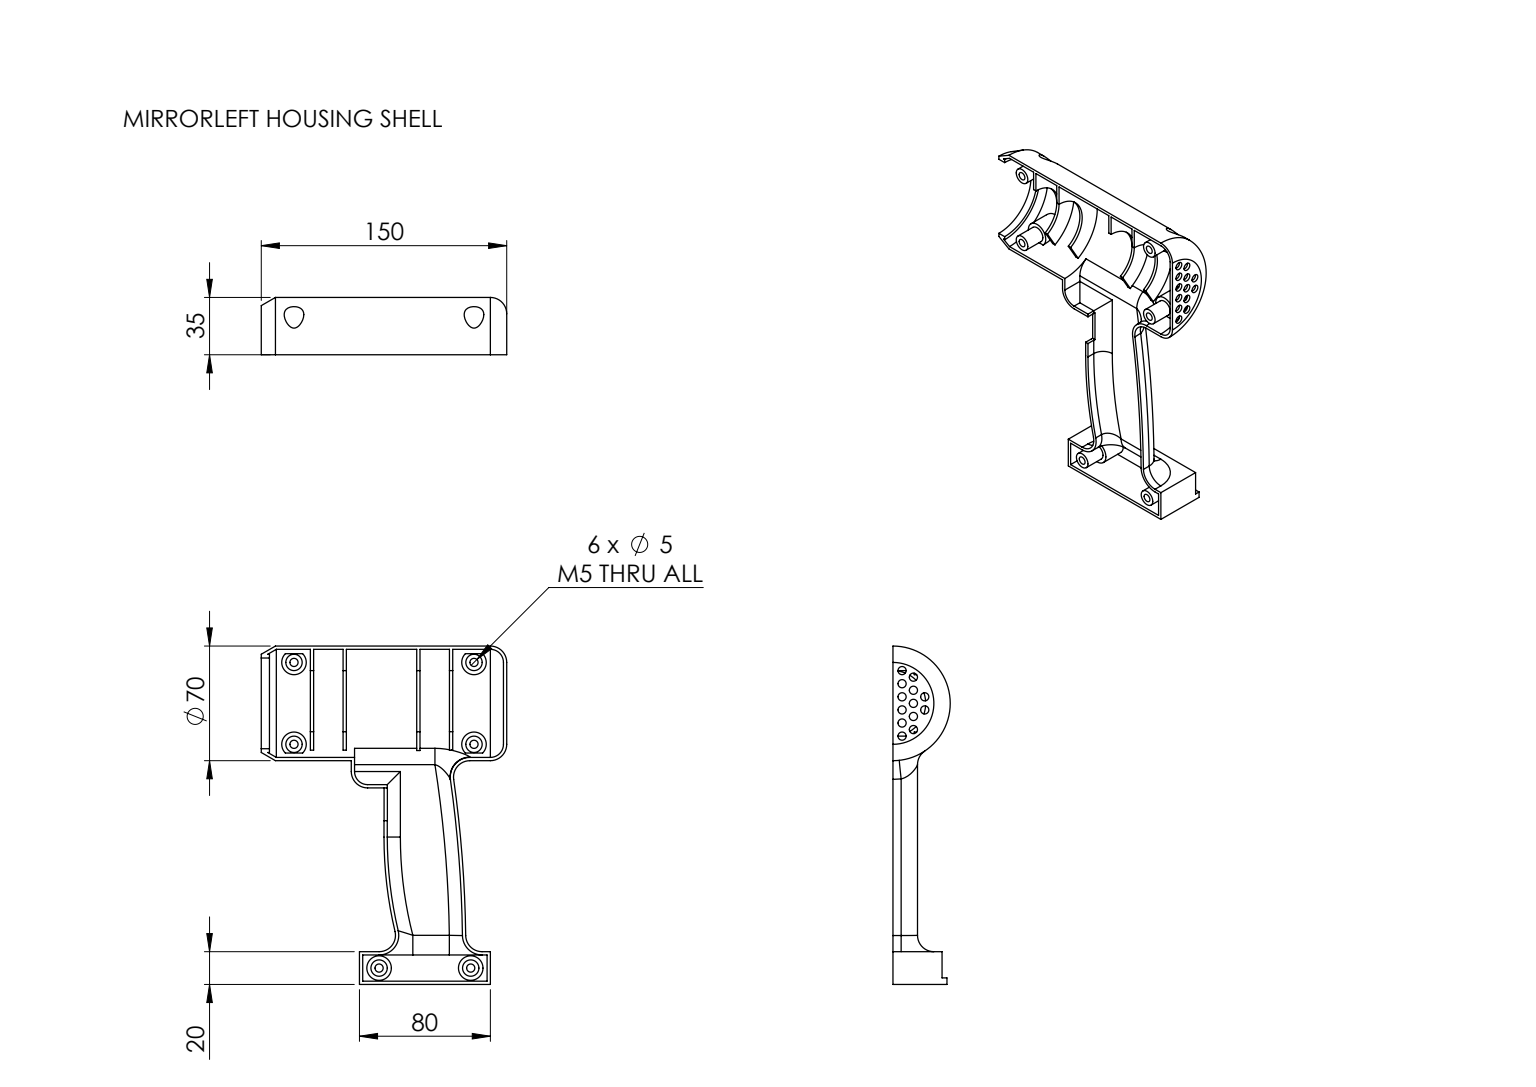
ISO-10303-21;
HEADER;
FILE_DESCRIPTION (('STEP AP214'),
    '1' );
FILE_NAME ('MirrorLeft Housing Shell.step',
    '2026-10-05T20:22:16',
    ( '' ),
    ( '' ),
    'SwSTEP 2.0',
    'SolidWorks 2026',
    '' );
FILE_SCHEMA (( 'AUTOMOTIVE_DESIGN' ));
ENDSEC;

DATA;
#1=B_SPLINE_CURVE_WITH_KNOTS ( 'NONE', 3,
 ( #12352, #9685, #8096, #1383, #14752, #16256, #12262, #13513, #2624, #1474, #13417, #8273, #9424, #10672, #226, #14828, #5538, #2709, #8188, #5630, #16442, #6792, #7929, #6603, #12185, #55, #13336, #5455, #10843, #10926, #4124, #11996, #2798, #16348, #13681, #6869, #9602, #15004, #9865, #16607, #8540, #3321, #16516, #15178, #7128, #4646, #4480, #11188, #15272, #15441 ),
 .UNSPECIFIED., .F., .F.,
 ( 4, 2, 2, 2, 2, 2, 2, 2, 2, 2, 2, 2, 2, 2, 2, 2, 2, 2, 2, 2, 2, 2, 2, 2, 4 ),
 ( 0.02172192739389853383, 0.02251948391625541862, 0.02331704043861230341, 0.02491215348332601748, 0.02650726652803973155, 0.02810237957275344908, 0.02969749261746715968, 0.03129260566218088069, 0.03209016218453770303, 0.03288771870689453231, 0.03328649696807296082, 0.03368527522925138240, 0.03448283175160819780, 0.03528038827396501320, 0.03567916653514340702, 0.03607794479632180085, 0.03687550131867862319, 0.03767305784103544553, 0.03847061436339226786, 0.03926817088574909020, 0.04086328393046270713, 0.04245839697517631711, 0.04405351001988992710, 0.04564862306460354402, 0.04724373610931716094 ),
 .UNSPECIFIED. ) ;
#5=DIRECTION ( 'NONE',  ( 0.000000000000000000, 0.000000000000000000, 1.000000000000000000 ) ) ;
#6=CARTESIAN_POINT ( 'NONE',  ( 27.15273249069231198, 18.00000000000000000, -20.88767039909325973 ) ) ;
#7=CARTESIAN_POINT ( 'NONE',  ( 25.49876332522149625, 18.00000000000000000, -21.99427390110736624 ) ) ;
#8=CYLINDRICAL_SURFACE ( 'NONE', #14336, 2.500000000000000444 ) ;
#9=DIRECTION ( 'NONE',  ( -1.000000000000000000, 0.000000000000000000, 0.000000000000000000 ) ) ;
#10=DIRECTION ( 'NONE',  ( -1.000000000000000000, -0.000000000000000000, -0.000000000000000000 ) ) ;
#13=CARTESIAN_POINT ( 'NONE',  ( 16.03791926353974162, 127.7299327228906520, -9.742640703122631862 ) ) ;
#14=CIRCLE ( 'NONE', #9896, 10.00000000000000178 ) ;
#18=CIRCLE ( 'NONE', #14435, 20.00000000000000355 ) ;
#23=ORIENTED_EDGE ( 'NONE', *, *, #10609, .T. ) ;
#26=AXIS2_PLACEMENT_3D ( 'NONE', #12707, #5981, #16782 ) ;
#28=AXIS2_PLACEMENT_3D ( 'NONE', #8615, #16596, #11271 ) ;
#31=DIRECTION ( 'NONE',  ( 0.000000000000000000, 0.000000000000000000, -1.000000000000000000 ) ) ;
#35=ORIENTED_EDGE ( 'NONE', *, *, #2235, .F. ) ;
#37=ORIENTED_EDGE ( 'NONE', *, *, #4762, .T. ) ;
#38=CARTESIAN_POINT ( 'NONE',  ( -80.30638721710498373, 189.1234298779548624, -27.97726104294732963 ) ) ;
#43=ORIENTED_EDGE ( 'NONE', *, *, #9422, .T. ) ;
#48=FACE_OUTER_BOUND ( 'NONE', #5615, .T. ) ;
#50=CARTESIAN_POINT ( 'NONE',  ( -48.00000000000000000, 143.0439382767972347, -16.49999999999984368 ) ) ;
#55=CARTESIAN_POINT ( 'NONE',  ( -79.71276265205243305, 202.6220268295897711, -16.24950730846250835 ) ) ;
#57=CARTESIAN_POINT ( 'NONE',  ( -95.00000000000000000, 171.6227766016838245, 0.000000000000000000 ) ) ;
#60=DIRECTION ( 'NONE',  ( 1.000000000000000000, 0.000000000000000000, 0.000000000000000000 ) ) ;
#62=ORIENTED_EDGE ( 'NONE', *, *, #6340, .T. ) ;
#65=SHAPE_REPRESENTATION_RELATIONSHIP ( 'NONE' , 'NONE' ,  #7924, #8036 ) ;
#67=DIRECTION ( 'NONE',  ( 8.673617379884037937E-17, 0.000000000000000000, 1.000000000000000000 ) ) ;
#70=EDGE_LOOP ( 'NONE', ( #17465, #2421, #13202, #13512 ) ) ;
#72=CARTESIAN_POINT ( 'NONE',  ( -48.00000000000000000, 191.6227766016837961, 1.224646799147353454E-15 ) ) ;
#73=DIRECTION ( 'NONE',  ( 1.000000000000000000, 0.000000000000000000, 0.000000000000000000 ) ) ;
#75=CARTESIAN_POINT ( 'NONE',  ( 15.93460003626540100, 136.8193095811535045, -3.708327557688629206 ) ) ;
#79=ORIENTED_EDGE ( 'NONE', *, *, #12627, .T. ) ;
#80=DIRECTION ( 'NONE',  ( 1.000000000000000000, 0.000000000000000000, 0.000000000000000000 ) ) ;
#82=LINE ( 'NONE', #2908, #5241 ) ;
#84=CARTESIAN_POINT ( 'NONE',  ( -74.45226540305546337, 194.3303362407250177, -26.63481108765543581 ) ) ;
#88=CARTESIAN_POINT ( 'NONE',  ( 24.94691999498327206, 18.00000000000000711, -22.32501294936691139 ) ) ;
#89=CARTESIAN_POINT ( 'NONE',  ( 23.77503517897901375, 18.00000000000000000, -22.95135521423614833 ) ) ;
#90=CARTESIAN_POINT ( 'NONE',  ( 37.50000000000000711, 196.6227766016838245, -35.00200000000000244 ) ) ;
#93=CARTESIAN_POINT ( 'NONE',  ( 26.85005685037350176, 141.4992599418080772, -17.82476597062854040 ) ) ;
#94=ORIENTED_EDGE ( 'NONE', *, *, #1318, .F. ) ;
#95=CARTESIAN_POINT ( 'NONE',  ( 6.927042533203191965, 134.0880917650273716, -15.00000000000000533 ) ) ;
#97=DIRECTION ( 'NONE',  ( 0.000000000000000000, 0.000000000000000000, 1.000000000000000000 ) ) ;
#98=CARTESIAN_POINT ( 'NONE',  ( 225.0000000000000000, 89.99999999999997158, -4.999999999999999112 ) ) ;
#101=LINE ( 'NONE', #8243, #15842 ) ;
#102=VERTEX_POINT ( 'NONE', #8434 ) ;
#107=CARTESIAN_POINT ( 'NONE',  ( 33.99999999999998579, 9.999999999999998224, -35.00000000000000000 ) ) ;
#108=ORIENTED_EDGE ( 'NONE', *, *, #12256, .F. ) ;
#110=ORIENTED_EDGE ( 'NONE', *, *, #17517, .F. ) ;
#112=EDGE_CURVE ( 'NONE', #17297, #3029, #16627, .T. ) ;
#113=ORIENTED_EDGE ( 'NONE', *, *, #13886, .F. ) ;
#114=EDGE_CURVE ( 'NONE', #730, #9326, #14586, .T. ) ;
#115=CARTESIAN_POINT ( 'NONE',  ( -78.86500048027876630, 189.1866491494219815, -27.93804624201380804 ) ) ;
#116=DIRECTION ( 'NONE',  ( 0.000000000000000000, 0.000000000000000000, 1.000000000000000000 ) ) ;
#117=( BOUNDED_SURFACE ( )  B_SPLINE_SURFACE ( 3, 2, ( 
 ( #14255, #2119, #7358 ),
 ( #807, #6197, #12760 ),
 ( #632, #11415, #4699 ),
 ( #16827, #8771, #2299 ),
 ( #9106, #17259, #13450 ),
 ( #5135, #5041, #10344 ),
 ( #3799, #16120, #1322 ),
 ( #15926, #965, #13280 ),
 ( #13364, #6550, #2476 ),
 ( #14512, #14600, #10434 ),
 ( #15848, #1058, #6637 ),
 ( #11850, #2379, #3721 ),
 ( #6458, #16018, #11941 ),
 ( #8042, #15754, #7870 ),
 ( #7772, #5213, #10523 ),
 ( #10610, #6729, #9194 ),
 ( #13185, #1148, #17343 ),
 ( #3900, #9284, #12126 ),
 ( #3631, #4951, #3997 ),
 ( #14695, #11759, #2575 ),
 ( #7961, #1231, #9021 ),
 ( #14436, #7692, #9377 ),
 ( #13099, #12030, #17435 ),
 ( #6362, #5310, #17170 ),
 ( #14779, #10704, #2651 ),
 ( #13711, #13812, #9715 ),
 ( #11051, #256, #7075 ),
 ( #1415, #4329, #341 ),
 ( #4156, #8392, #9541 ),
 ( #8220, #1582, #3039 ) ),
 .UNSPECIFIED., .F., .F., .F. ) 
 B_SPLINE_SURFACE_WITH_KNOTS ( ( 4, 2, 2, 2, 2, 2, 2, 2, 2, 2, 2, 2, 2, 2, 4 ),
 ( 3, 3 ),
 ( 0.01165250788892075590, 0.01579789672993321681, 0.01787059115043944726, 0.01890693836069256423, 0.01994328557094567772, 0.02408867441195813863, 0.02616136883246436562, 0.02823406325297059608, 0.03030675767347682653, 0.03237945209398305352, 0.03652484093499551443, 0.03859753535550174142, 0.03963388256575485491, 0.04067022977600797534, 0.04481561861702043625 ),
 ( 0.000000000000000000, 1.000000000000000000 ),
 .UNSPECIFIED. ) 
 GEOMETRIC_REPRESENTATION_ITEM ( )  RATIONAL_B_SPLINE_SURFACE ( (
 ( 1.000000000000000000, 0.8819171036881968684, 1.000000000000000000),
 ( 1.000000000000000000, 0.8793942645247271317, 1.000000000000000000),
 ( 1.000000000000000000, 0.8749458316895473153, 1.000000000000000000),
 ( 1.000000000000000000, 0.8656814021268807169, 1.000000000000000000),
 ( 1.000000000000000000, 0.8621600075895787807, 1.000000000000000000),
 ( 1.000000000000000000, 0.8562492930711512740, 1.000000000000000000),
 ( 1.000000000000000000, 0.8541736901086096623, 1.000000000000000000),
 ( 1.000000000000000000, 0.8498659178638878764, 1.000000000000000000),
 ( 1.000000000000000000, 0.8476283308600994770, 1.000000000000000000),
 ( 1.000000000000000000, 0.8360458749413697266, 1.000000000000000000),
 ( 1.000000000000000000, 0.8255221978283152628, 1.000000000000000000),
 ( 1.000000000000000000, 0.8082270345000643896, 1.000000000000000000),
 ( 1.000000000000000000, 0.8022128341713220534, 1.000000000000000000),
 ( 1.000000000000000000, 0.7899684886175323273, 1.000000000000000000),
 ( 1.000000000000000000, 0.7837128169312477244, 1.000000000000000000),
 ( 1.000000000000000000, 0.7710263478628327505, 1.000000000000000000),
 ( 1.000000000000000000, 0.7645952338537677084, 1.000000000000000000),
 ( 1.000000000000000000, 0.7516613202047349729, 1.000000000000000000),
 ( 1.000000000000000000, 0.7451386183435962929, 1.000000000000000000),
 ( 1.000000000000000000, 0.7257808243687768890, 1.000000000000000000),
 ( 1.000000000000000000, 0.7133953845776382918, 1.000000000000000000),
 ( 1.000000000000000000, 0.6965170042221158209, 1.000000000000000000),
 ( 1.000000000000000000, 0.6911767420096451842, 1.000000000000000000),
 ( 1.000000000000000000, 0.6837405640632109316, 1.000000000000000000),
 ( 1.000000000000000000, 0.6813577907324296357, 1.000000000000000000),
 ( 1.000000000000000000, 0.6768117804540668692, 1.000000000000000000),
 ( 1.000000000000000000, 0.6746439590912666207, 1.000000000000000000),
 ( 1.000000000000000000, 0.6645663254999827352, 1.000000000000000000),
 ( 1.000000000000000000, 0.6588263891900785207, 1.000000000000000000),
 ( 1.000000000000000000, 0.6558243695371216431, 1.000000000000000000) ) ) 
 REPRESENTATION_ITEM ( '' )  SURFACE ( )  );
#125=ADVANCED_FACE ( 'NONE', ( #16843, #6296, #6218, #3209, #822 ), #15422, .T. ) ;
#128=DIRECTION ( 'NONE',  ( -1.000000000000000000, -0.000000000000000000, -0.000000000000000000 ) ) ;
#129=DIRECTION ( 'NONE',  ( 0.000000000000000000, 0.000000000000000000, 1.000000000000000000 ) ) ;
#130=CARTESIAN_POINT ( 'NONE',  ( 22.12508471281541134, 29.85770821936580433, -8.546410110412809402 ) ) ;
#136=CIRCLE ( 'NONE', #10306, 12.00000000000000000 ) ;
#137=CARTESIAN_POINT ( 'NONE',  ( 34.80468147095351128, 20.00000000000000000, -7.619145204522578041 ) ) ;
#141=ORIENTED_EDGE ( 'NONE', *, *, #16389, .F. ) ;
#147=ORIENTED_EDGE ( 'NONE', *, *, #10920, .T. ) ;
#149=CARTESIAN_POINT ( 'NONE',  ( 15.95607457768013404, 136.6882381644216196, -2.475222843548684715 ) ) ;
#150=LINE ( 'NONE', #5809, #16568 ) ;
#152=VERTEX_POINT ( 'NONE', #7624 ) ;
#158=CIRCLE ( 'NONE', #16310, 33.00000000000000000 ) ;
#159=CARTESIAN_POINT ( 'NONE',  ( 20.41303537792882139, 140.1262507166239573, -15.26811025958205015 ) ) ;
#160=VERTEX_POINT ( 'NONE', #11356 ) ;
#162=FACE_OUTER_BOUND ( 'NONE', #7033, .T. ) ;
#164=CARTESIAN_POINT ( 'NONE',  ( -76.63222342921277175, 191.6397216241467163, -28.71272404723380234 ) ) ;
#166=AXIS2_PLACEMENT_3D ( 'NONE', #4042, #9504, #12180 ) ;
#169=DIRECTION ( 'NONE',  ( -1.000000000000000000, -0.000000000000000000, 0.000000000000000000 ) ) ;
#173=ADVANCED_FACE ( 'NONE', ( #16682 ), #11434, .F. ) ;
#175=FACE_OUTER_BOUND ( 'NONE', #10777, .T. ) ;
#176=EDGE_CURVE ( 'NONE', #5792, #4284, #10914, .T. ) ;
#180=EDGE_LOOP ( 'NONE', ( #8241, #14719, #12649, #3237 ) ) ;
#182=CIRCLE ( 'NONE', #5556, 239.9999999999999716 ) ;
#183=AXIS2_PLACEMENT_3D ( 'NONE', #7714, #6580, #13125 ) ;
#184=CARTESIAN_POINT ( 'NONE',  ( -50.00000000000000000, 204.6227766016838245, 2.020667218593133100E-15 ) ) ;
#185=VECTOR ( 'NONE', #14301, 1000.000000000000114 ) ;
#191=CARTESIAN_POINT ( 'NONE',  ( 36.34904889156061358, 150.6223998522366685, -25.45681811525070515 ) ) ;
#192=ORIENTED_EDGE ( 'NONE', *, *, #2912, .T. ) ;
#194=CARTESIAN_POINT ( 'NONE',  ( -40.00000000000000000, 4.000000000000000000, -30.00000000000000711 ) ) ;
#196=EDGE_LOOP ( 'NONE', ( #16642, #10984, #15395, #3760 ) ) ;
#197=EDGE_CURVE ( 'NONE', #6224, #17297, #182, .T. ) ;
#201=ORIENTED_EDGE ( 'NONE', *, *, #8299, .T. ) ;
#203=ORIENTED_EDGE ( 'NONE', *, *, #13054, .T. ) ;
#204=CARTESIAN_POINT ( 'NONE',  ( -87.34717144291671787, 195.0632477915243896, -23.23525722188765741 ) ) ;
#207=CARTESIAN_POINT ( 'NONE',  ( 48.00000000000000711, 175.6227766016838245, -5.571800142134975431 ) ) ;
#209=VERTEX_POINT ( 'NONE', #8951 ) ;
#211=AXIS2_PLACEMENT_3D ( 'NONE', #6627, #17422, #13266 ) ;
#214=DIRECTION ( 'NONE',  ( 0.000000000000000000, -1.000000000000000000, -6.123233995736762338E-17 ) ) ;
#218=DIRECTION ( 'NONE',  ( 1.000000000000000000, 0.000000000000000000, -0.000000000000000000 ) ) ;
#219=ADVANCED_FACE ( 'NONE', ( #14195 ), #2057, .T. ) ;
#220=CARTESIAN_POINT ( 'NONE',  ( 32.50000000000000711, 146.6227766016838245, -16.00000000000000000 ) ) ;
#221=CARTESIAN_POINT ( 'NONE',  ( 17.51497691750854813, 29.94811823131043127, -12.57651788136221072 ) ) ;
#222=CARTESIAN_POINT ( 'NONE',  ( -40.00000000000000000, 0.000000000000000000, -33.00000000000000711 ) ) ;
#226=CARTESIAN_POINT ( 'NONE',  ( -83.14616744761717371, 201.7487681645689577, -17.82060658420953203 ) ) ;
#227=DIRECTION ( 'NONE',  ( 0.000000000000000000, 0.000000000000000000, 1.000000000000000000 ) ) ;
#228=CARTESIAN_POINT ( 'NONE',  ( -72.50000000000002842, 146.6227766016838245, -35.00200000000000244 ) ) ;
#230=VECTOR ( 'NONE', #15433, 1000.000000000000000 ) ;
#234=CARTESIAN_POINT ( 'NONE',  ( 48.00000000000000000, 171.6227766016838245, 0.000000000000000000 ) ) ;
#238=AXIS2_PLACEMENT_3D ( 'NONE', #16301, #6473, #17358 ) ;
#240=EDGE_CURVE ( 'NONE', #15883, #846, #6193, .T. ) ;
#242=CARTESIAN_POINT ( 'NONE',  ( -95.00000000000000000, 171.6227766016838245, 0.000000000000000000 ) ) ;
#243=VERTEX_POINT ( 'NONE', #13302 ) ;
#246=DIRECTION ( 'NONE',  ( -0.000000000000000000, -0.000000000000000000, -1.000000000000000000 ) ) ;
#251=AXIS2_PLACEMENT_3D ( 'NONE', #3268, #2197, #881 ) ;
#253=CARTESIAN_POINT ( 'NONE',  ( 14.17453072134883030, 137.9246278893784847, -11.09209212451273352 ) ) ;
#256=CARTESIAN_POINT ( 'NONE',  ( 14.12141184870282196, 138.6801925718470443, -3.743222489502411321 ) ) ;
#257=ORIENTED_EDGE ( 'NONE', *, *, #3098, .T. ) ;
#259=CARTESIAN_POINT ( 'NONE',  ( -80.44925623706835438, 190.6352453962669813, -29.38582951075080985 ) ) ;
#260=DIRECTION ( 'NONE',  ( -0.000000000000000000, -0.000000000000000000, -1.000000000000000000 ) ) ;
#263=CARTESIAN_POINT ( 'NONE',  ( -43.00000000000000000, 130.0000000000000000, -15.00000000000000000 ) ) ;
#267=CARTESIAN_POINT ( 'NONE',  ( 11.38015211399644500, 143.8700659084811093, -17.85516819212570638 ) ) ;
#269=ORIENTED_EDGE ( 'NONE', *, *, #1597, .F. ) ;
#270=ORIENTED_EDGE ( 'NONE', *, *, #12627, .F. ) ;
#271=CARTESIAN_POINT ( 'NONE',  ( 24.41196201396447663, 19.99999999999999645, -8.570466955472159754 ) ) ;
#274=CARTESIAN_POINT ( 'NONE',  ( 24.00000000000000000, 196.6227766016838245, -16.00000000000000000 ) ) ;
#275=ORIENTED_EDGE ( 'NONE', *, *, #16105, .F. ) ;
#278=DIRECTION ( 'NONE',  ( 1.000000000000000000, 0.000000000000000000, 0.000000000000000000 ) ) ;
#281=EDGE_CURVE ( 'NONE', #6275, #15920, #15863, .T. ) ;
#282=CARTESIAN_POINT ( 'NONE',  ( -50.00000000000000000, 171.6227766016838245, 0.000000000000000000 ) ) ;
#286=AXIS2_PLACEMENT_3D ( 'NONE', #5190, #14314, #1029 ) ;
#289=PLANE ( 'NONE',  #9740 ) ;
#290=CIRCLE ( 'NONE', #10181, 33.00000000000000000 ) ;
#293=CARTESIAN_POINT ( 'NONE',  ( 225.0000000000000000, 89.99999999999997158, -4.999999999999999112 ) ) ;
#295=CARTESIAN_POINT ( 'NONE',  ( -72.55951795904178425, 195.6584727333609521, -22.61345334826514630 ) ) ;
#296=FACE_BOUND ( 'NONE', #6496, .T. ) ;
#298=ORIENTED_EDGE ( 'NONE', *, *, #12256, .T. ) ;
#299=EDGE_LOOP ( 'NONE', ( #9917, #12342, #13408, #14524 ) ) ;
#300=CARTESIAN_POINT ( 'NONE',  ( -90.80384757729339640, 204.6227766016838245, 0.000000000000000000 ) ) ;
#305=EDGE_CURVE ( 'NONE', #13136, #4801, #3737, .T. ) ;
#309=DIRECTION ( 'NONE',  ( -0.000000000000000000, -0.000000000000000000, -1.000000000000000000 ) ) ;
#316=FACE_OUTER_BOUND ( 'NONE', #16097, .T. ) ;
#318=CARTESIAN_POINT ( 'NONE',  ( -45.00000000000000000, 130.0000000000000000, 0.000000000000000000 ) ) ;
#325=AXIS2_PLACEMENT_3D ( 'NONE', #12063, #5342, #16056 ) ;
#328=CARTESIAN_POINT ( 'NONE',  ( -16.30611068361787019, 32.76923076923078781, -4.999999999999999112 ) ) ;
#329=LINE ( 'NONE', #4059, #732 ) ;
#332=EDGE_LOOP ( 'NONE', ( #9563, #15113 ) ) ;
#338=CARTESIAN_POINT ( 'NONE',  ( 25.02538947967125793, 138.3580044269788800, -10.92703196337285299 ) ) ;
#340=CARTESIAN_POINT ( 'NONE',  ( -74.59180618087658843, 149.2475623141791061, -26.91697313366100985 ) ) ;
#341=CARTESIAN_POINT ( 'NONE',  ( 27.25143353317894324, 139.0964629073462220, -5.659441210211040740 ) ) ;
#344=CARTESIAN_POINT ( 'NONE',  ( -77.78509460342800708, 191.0296277843087296, -29.12775510238319399 ) ) ;
#346=DIRECTION ( 'NONE',  ( 0.000000000000000000, 0.000000000000000000, -1.000000000000000000 ) ) ;
#352=DIRECTION ( 'NONE',  ( 1.000000000000000000, 0.000000000000000000, 0.000000000000000000 ) ) ;
#355=CARTESIAN_POINT ( 'NONE',  ( 34.93420767782698988, 19.99999999999999645, -6.321724734770472587 ) ) ;
#356=B_SPLINE_CURVE_WITH_KNOTS ( 'NONE', 3,
 ( #7684, #11748, #15744, #10079, #15575, #885, #3452, #9097, #3622, #16818, #9013, #14426, #12830, #2290, #14173, #621, #2110, #11499, #13092, #10426, #17157, #3713, #6274, #15486, #7510, #10172, #957, #3367, #2372, #8840, #14245, #8761, #2034, #12919, #15652, #11589, #16996, #4863, #6352, #3529, #14505, #8920, #11664, #8122, #3791, #2468, #11934, #9443, #9277, #16010 ),
 .UNSPECIFIED., .F., .F.,
 ( 4, 2, 2, 2, 2, 2, 2, 2, 2, 2, 2, 2, 2, 2, 2, 2, 2, 2, 2, 2, 2, 2, 2, 2, 4 ),
 ( 0.02172192739389855118, 0.02251948391625536658, 0.02331704043861218198, 0.02491215348332581278, 0.02650726652803944358, 0.02810237957275307438, 0.02969749261746670171, 0.03129260566218033252, 0.03209016218453714098, 0.03288771870689394250, 0.03328649696807235020, 0.03368527522925075790, 0.03448283175160756636, 0.03528038827396437482, 0.03567916653514278946, 0.03607794479632120410, 0.03687550131867804726, 0.03767305784103488348, 0.03847061436339171969, 0.03926817088574855591, 0.04086328393046227692, 0.04245839697517599792, 0.04405351001988971893, 0.04564862306460343994, 0.04724373610931716094 ),
 .UNSPECIFIED. ) ;
#357=DIRECTION ( 'NONE',  ( 8.673617379884037937E-17, 0.000000000000000000, 1.000000000000000000 ) ) ;
#358=EDGE_LOOP ( 'NONE', ( #12471, #2318, #7218, #8842 ) ) ;
#361=CYLINDRICAL_SURFACE ( 'NONE', #2522, 248.0000000000000000 ) ;
#362=ORIENTED_EDGE ( 'NONE', *, *, #2234, .T. ) ;
#363=CARTESIAN_POINT ( 'NONE',  ( 37.21337428997476593, 198.7412861714591941, -18.82352572523459600 ) ) ;
#369=CARTESIAN_POINT ( 'NONE',  ( -100.0000000000000000, 142.8100939375178200, -16.63501009223129756 ) ) ;
#371=ORIENTED_EDGE ( 'NONE', *, *, #3539, .F. ) ;
#372=CARTESIAN_POINT ( 'NONE',  ( 24.48161681970857018, 138.6020828307752879, -11.64873334838780572 ) ) ;
#373=EDGE_CURVE ( 'NONE', #8849, #8796, #6836, .T. ) ;
#376=CARTESIAN_POINT ( 'NONE',  ( -8.461393309425545795, 30.35704578695612099, -12.95687587100684368 ) ) ;
#377=EDGE_LOOP ( 'NONE', ( #3921, #10271, #6852, #11471 ) ) ;
#379=LINE ( 'NONE', #5779, #16244 ) ;
#384=LINE ( 'NONE', #14028, #11479 ) ;
#390=DIRECTION ( 'NONE',  ( 0.000000000000000000, 0.000000000000000000, 1.000000000000000000 ) ) ;
#392=ADVANCED_FACE ( 'NONE', ( #6907 ), #7804, .F. ) ;
#393=DIRECTION ( 'NONE',  ( 1.000000000000000000, 0.000000000000000000, 0.000000000000000000 ) ) ;
#395=CARTESIAN_POINT ( 'NONE',  ( 27.15273249069231198, 19.99999999999999645, -20.88767039909325973 ) ) ;
#397=DIRECTION ( 'NONE',  ( -0.000000000000000000, -0.000000000000000000, 1.000000000000000000 ) ) ;
#398=AXIS2_PLACEMENT_3D ( 'NONE', #9363, #2641, #5198 ) ;
#399=VERTEX_POINT ( 'NONE', #184 ) ;
#406=CIRCLE ( 'NONE', #6632, 12.00000000000000000 ) ;
#408=CARTESIAN_POINT ( 'NONE',  ( -24.99999999999999289, 100.0000000000000142, -15.00000000000000000 ) ) ;
#410=CARTESIAN_POINT ( 'NONE',  ( 29.53214135918722505, 18.00000000000000000, -18.68621337607990185 ) ) ;
#413=DIRECTION ( 'NONE',  ( 0.000000000000000000, 0.000000000000000000, 1.000000000000000000 ) ) ;
#415=LINE ( 'NONE', #5821, #443 ) ;
#417=PLANE ( 'NONE',  #8765 ) ;
#418=AXIS2_PLACEMENT_3D ( 'NONE', #14483, #7741, #8010 ) ;
#419=ORIENTED_EDGE ( 'NONE', *, *, #3121, .F. ) ;
#421=EDGE_LOOP ( 'NONE', ( #5552, #2069, #2676, #10202 ) ) ;
#422=CARTESIAN_POINT ( 'NONE',  ( -75.17085894487867392, 193.0398713882428012, -27.68487141596273915 ) ) ;
#424=LINE ( 'NONE', #5834, #8946 ) ;
#428=CARTESIAN_POINT ( 'NONE',  ( -95.00000000000000000, 171.6227766016838245, 0.000000000000000000 ) ) ;
#433=FACE_BOUND ( 'NONE', #13642, .T. ) ;
#434=ORIENTED_EDGE ( 'NONE', *, *, #16551, .T. ) ;
#436=CARTESIAN_POINT ( 'NONE',  ( 24.40970717605596718, 29.87515913883691354, -8.215055496182330330 ) ) ;
#437=CARTESIAN_POINT ( 'NONE',  ( 27.04079503965286690, 139.2301514590222098, -6.313402927548398047 ) ) ;
#441=VECTOR ( 'NONE', #9945, 1000.000000000000000 ) ;
#443=VECTOR ( 'NONE', #15203, 1000.000000000000000 ) ;
#444=DIRECTION ( 'NONE',  ( -1.000000000000000000, -0.000000000000000000, -0.000000000000000000 ) ) ;
#447=DIRECTION ( 'NONE',  ( -0.000000000000000000, -0.000000000000000000, -1.000000000000000000 ) ) ;
#451=CARTESIAN_POINT ( 'NONE',  ( -74.40218896425085404, 141.6107120069882512, -13.74530841833676220 ) ) ;
#452=AXIS2_PLACEMENT_3D ( 'NONE', #1785, #447, #9743 ) ;
#453=VERTEX_POINT ( 'NONE', #5588 ) ;
#457=VERTEX_POINT ( 'NONE', #10979 ) ;
#458=EDGE_CURVE ( 'NONE', #11543, #11435, #15731, .T. ) ;
#460=EDGE_CURVE ( 'NONE', #8505, #14597, #2443, .T. ) ;
#463=DIRECTION ( 'NONE',  ( 1.000000000000000000, 0.000000000000000000, 0.000000000000000000 ) ) ;
#464=CYLINDRICAL_SURFACE ( 'NONE', #1410, 2.499999999999998668 ) ;
#467=AXIS2_PLACEMENT_3D ( 'NONE', #16027, #3907, #7967 ) ;
#468=ORIENTED_EDGE ( 'NONE', *, *, #15742, .T. ) ;
#470=ADVANCED_FACE ( 'NONE', ( #12227 ), #3105, .T. ) ;
#474=DIRECTION ( 'NONE',  ( -1.000000000000000000, 0.000000000000000000, 0.000000000000000000 ) ) ;
#479=CARTESIAN_POINT ( 'NONE',  ( -7.379000772444995526, 30.00000000000000000, -13.00000000000000178 ) ) ;
#483=CARTESIAN_POINT ( 'NONE',  ( 32.91012024024373517, 19.99999999999999289, -13.86436652238006673 ) ) ;
#486=ORIENTED_EDGE ( 'NONE', *, *, #6340, .F. ) ;
#489=VERTEX_POINT ( 'NONE', #13915 ) ;
#490=ORIENTED_EDGE ( 'NONE', *, *, #17231, .F. ) ;
#492=CYLINDRICAL_SURFACE ( 'NONE', #1416, 10.00000000000000178 ) ;
#496=EDGE_CURVE ( 'NONE', #16329, #13265, #6750, .T. ) ;
#497=EDGE_CURVE ( 'NONE', #6006, #5256, #4292, .T. ) ;
#498=DIRECTION ( 'NONE',  ( -1.000000000000000000, -0.000000000000000000, 0.000000000000000000 ) ) ;
#500=CIRCLE ( 'NONE', #10943, 10.00000000000000178 ) ;
#503=CARTESIAN_POINT ( 'NONE',  ( -45.00000000000000000, 130.0000000000000000, -15.00000000000000000 ) ) ;
#510=DIRECTION ( 'NONE',  ( -1.000000000000000000, 0.000000000000000000, 0.000000000000000000 ) ) ;
#511=CARTESIAN_POINT ( 'NONE',  ( -8.766611209710754693, 19.99999999999771916, -14.60748648876205458 ) ) ;
#516=ORIENTED_EDGE ( 'NONE', *, *, #7943, .F. ) ;
#523=DIRECTION ( 'NONE',  ( 1.000000000000000000, 0.000000000000000000, 0.000000000000000000 ) ) ;
#525=CARTESIAN_POINT ( 'NONE',  ( -725.0000000000000000, 30.00000000000000000, -25.00000000000000000 ) ) ;
#537=CARTESIAN_POINT ( 'NONE',  ( 24.72170379509201865, 19.99999999999999645, -7.619165077982883894 ) ) ;
#538=CARTESIAN_POINT ( 'NONE',  ( 19.59022622986824302, 142.1737554346910599, -14.89790021284453303 ) ) ;
#539=VERTEX_POINT ( 'NONE', #274 ) ;
#543=AXIS2_PLACEMENT_3D ( 'NONE', #9206, #16030, #16296 ) ;
#546=PLANE ( 'NONE',  #7342 ) ;
#553=CARTESIAN_POINT ( 'NONE',  ( -72.50000000000002842, 146.6227766016838245, -21.54065922853802562 ) ) ;
#555=CYLINDRICAL_SURFACE ( 'NONE', #8157, 33.00000000000000000 ) ;
#559=ORIENTED_EDGE ( 'NONE', *, *, #15927, .T. ) ;
#561=VECTOR ( 'NONE', #2674, 1000.000000000000000 ) ;
#562=CARTESIAN_POINT ( 'NONE',  ( -26.10410744458347665, 18.00000000000000000, -13.37721135299797304 ) ) ;
#564=EDGE_CURVE ( 'NONE', #4853, #5097, #11488, .T. ) ;
#566=DIRECTION ( 'NONE',  ( 0.000000000000000000, 0.000000000000000000, -1.000000000000000000 ) ) ;
#568=AXIS2_PLACEMENT_3D ( 'NONE', #14760, #4313, #60 ) ;
#569=AXIS2_PLACEMENT_3D ( 'NONE', #5580, #6650, #6830 ) ;
#571=CARTESIAN_POINT ( 'NONE',  ( 37.99999999999999289, 2.000000000000000000, -8.789265611615818404E-15 ) ) ;
#574=DIRECTION ( 'NONE',  ( 0.000000000000000000, 1.000000000000000000, 0.000000000000000000 ) ) ;
#575=EDGE_CURVE ( 'NONE', #8346, #5702, #12911, .T. ) ;
#579=CARTESIAN_POINT ( 'NONE',  ( -68.00000000000000000, 204.6227766016838245, 0.000000000000000000 ) ) ;
#583=VERTEX_POINT ( 'NONE', #4786 ) ;
#584=DIRECTION ( 'NONE',  ( 0.000000000000000000, 0.000000000000000000, 1.000000000000000000 ) ) ;
#585=CARTESIAN_POINT ( 'NONE',  ( -45.00000000000000000, 122.0000000000000142, -4.999999999999999112 ) ) ;
#588=VERTEX_POINT ( 'NONE', #3277 ) ;
#590=VECTOR ( 'NONE', #14056, 1000.000000000000000 ) ;
#593=DIRECTION ( 'NONE',  ( 1.000000000000000000, 0.000000000000000000, 0.000000000000000000 ) ) ;
#599=AXIS2_PLACEMENT_3D ( 'NONE', #14005, #3199, #15140 ) ;
#600=CARTESIAN_POINT ( 'NONE',  ( 25.00000000000000711, 146.6227766016838245, -12.99999999999999822 ) ) ;
#602=ORIENTED_EDGE ( 'NONE', *, *, #14098, .F. ) ;
#606=CARTESIAN_POINT ( 'NONE',  ( -8.792264229871568304, 30.31966024794114745, -14.93731107458715357 ) ) ;
#608=AXIS2_PLACEMENT_3D ( 'NONE', #6490, #13127, #6395 ) ;
#609=FACE_OUTER_BOUND ( 'NONE', #3195, .T. ) ;
#613=EDGE_LOOP ( 'NONE', ( #6152, #6292 ) ) ;
#614=CARTESIAN_POINT ( 'NONE',  ( -85.77828040291200296, 194.9977432358044496, -26.05112671349591125 ) ) ;
#615=DIRECTION ( 'NONE',  ( 0.000000000000000000, 1.000000000000000000, 0.000000000000000000 ) ) ;
#617=ORIENTED_EDGE ( 'NONE', *, *, #4810, .T. ) ;
#619=CYLINDRICAL_SURFACE ( 'NONE', #11277, 6.000000000000005329 ) ;
#621=CARTESIAN_POINT ( 'NONE',  ( 27.40877793924366301, 202.0384121146825578, -17.31838511551978144 ) ) ;
#624=EDGE_CURVE ( 'NONE', #1718, #6006, #5357, .T. ) ;
#625=EDGE_CURVE ( 'NONE', #4234, #16058, #12632, .T. ) ;
#626=ORIENTED_EDGE ( 'NONE', *, *, #13035, .T. ) ;
#627=CARTESIAN_POINT ( 'NONE',  ( 30.00000000000001066, 146.6227766016838245, -35.00200000000000244 ) ) ;
#631=DIRECTION ( 'NONE',  ( 0.000000000000000000, 0.000000000000000000, -1.000000000000000000 ) ) ;
#632=CARTESIAN_POINT ( 'NONE',  ( 7.290380404777190293, 133.8591131982526008, -12.94327073059132971 ) ) ;
#633=ORIENTED_EDGE ( 'NONE', *, *, #12413, .F. ) ;
#643=FACE_OUTER_BOUND ( 'NONE', #1205, .T. ) ;
#665=EDGE_LOOP ( 'NONE', ( #2497, #10383, #12994, #3390 ) ) ;
#667=DIRECTION ( 'NONE',  ( -1.000000000000000000, 0.000000000000000000, 0.000000000000000000 ) ) ;
#668=VERTEX_POINT ( 'NONE', #6105 ) ;
#671=EDGE_CURVE ( 'NONE', #11068, #15447, #12662, .T. ) ;
#679=CARTESIAN_POINT ( 'NONE',  ( 37.50000000000000711, 146.0561595177564129, -20.88304578468306261 ) ) ;
#680=EDGE_CURVE ( 'NONE', #399, #15865, #9191, .T. ) ;
#681=EDGE_LOOP ( 'NONE', ( #12915, #11101, #10298, #13282 ) ) ;
#683=CARTESIAN_POINT ( 'NONE',  ( 17.58250999373992585, 125.2198453306090329, 1.325401613797208934E-14 ) ) ;
#684=CARTESIAN_POINT ( 'NONE',  ( -80.00000000000002842, 146.6227766016838245, -16.00000000000000000 ) ) ;
#685=CARTESIAN_POINT ( 'NONE',  ( -13.51825462539708056, 19.99999999999884892, -10.94502331224290259 ) ) ;
#697=CARTESIAN_POINT ( 'NONE',  ( -85.89524066039361117, 195.4942584061382149, -25.59693137756977421 ) ) ;
#698=AXIS2_PLACEMENT_3D ( 'NONE', #16846, #8791, #6045 ) ;
#701=CARTESIAN_POINT ( 'NONE',  ( 15.53715976346056493, 125.3980538582347748, -5.670872899454017180 ) ) ;
#702=ORIENTED_EDGE ( 'NONE', *, *, #13472, .T. ) ;
#707=VECTOR ( 'NONE', #1161, 1000.000000000000000 ) ;
#709=VECTOR ( 'NONE', #13927, 1000.000000000000000 ) ;
#711=CARTESIAN_POINT ( 'NONE',  ( 24.93034343272635667, 19.99999999999999645, -22.33460256652156062 ) ) ;
#717=FACE_BOUND ( 'NONE', #9395, .T. ) ;
#718=CIRCLE ( 'NONE', #10601, 249.9999999999999716 ) ;
#720=EDGE_CURVE ( 'NONE', #16285, #7408, #500, .T. ) ;
#721=ADVANCED_FACE ( 'NONE', ( #6455 ), #11074, .F. ) ;
#726=CARTESIAN_POINT ( 'NONE',  ( 40.00000000000000711, 206.6227766016838245, 0.000000000000000000 ) ) ;
#727=CARTESIAN_POINT ( 'NONE',  ( 30.13973646015553243, 140.6228917578588948, -16.24829651775490902 ) ) ;
#730=VERTEX_POINT ( 'NONE', #10789 ) ;
#731=DIRECTION ( 'NONE',  ( 0.000000000000000000, 0.000000000000000000, 1.000000000000000000 ) ) ;
#732=VECTOR ( 'NONE', #9698, 1000.000000000000000 ) ;
#737=AXIS2_PLACEMENT_3D ( 'NONE', #15583, #12931, #3375 ) ;
#741=EDGE_CURVE ( 'NONE', #12240, #12970, #15109, .T. ) ;
#749=ORIENTED_EDGE ( 'NONE', *, *, #15171, .F. ) ;
#750=CYLINDRICAL_SURFACE ( 'NONE', #2202, 7.500000000000007105 ) ;
#752=EDGE_LOOP ( 'NONE', ( #6021, #16237, #7652, #6565 ) ) ;
#754=PLANE ( 'NONE',  #14591 ) ;
#755=ORIENTED_EDGE ( 'NONE', *, *, #1160, .T. ) ;
#756=ORIENTED_EDGE ( 'NONE', *, *, #9201, .F. ) ;
#761=ORIENTED_EDGE ( 'NONE', *, *, #2314, .F. ) ;
#770=EDGE_LOOP ( 'NONE', ( #2866, #6515, #15048, #9121 ) ) ;
#776=CARTESIAN_POINT ( 'NONE',  ( -14.56452549316047040, 20.00000000000115818, -9.027778560947799846 ) ) ;
#778=AXIS2_PLACEMENT_3D ( 'NONE', #2025, #16643, #10064 ) ;
#779=ADVANCED_FACE ( 'NONE', ( #2020 ), #5919, .F. ) ;
#780=CARTESIAN_POINT ( 'NONE',  ( 196.0000000000000000, 159.6227766016838814, -5.571800142134975431 ) ) ;
#784=ORIENTED_EDGE ( 'NONE', *, *, #496, .T. ) ;
#788=CIRCLE ( 'NONE', #8131, 5.000000000000000888 ) ;
#793=VERTEX_POINT ( 'NONE', #4418 ) ;
#794=CARTESIAN_POINT ( 'NONE',  ( 34.93420767853316988, 19.99999999999999645, 0.000000000000000000 ) ) ;
#795=CARTESIAN_POINT ( 'NONE',  ( 24.93507336697352628, 29.86842105263157876, -4.999999999999999112 ) ) ;
#796=PLANE ( 'NONE',  #12731 ) ;
#797=ORIENTED_EDGE ( 'NONE', *, *, #4142, .T. ) ;
#799=AXIS2_PLACEMENT_3D ( 'NONE', #5793, #6057, #1903 ) ;
#800=ORIENTED_EDGE ( 'NONE', *, *, #1703, .F. ) ;
#801=CARTESIAN_POINT ( 'NONE',  ( 17.68052782483612617, 29.96314637258912583, -14.61659083303745632 ) ) ;
#804=CARTESIAN_POINT ( 'NONE',  ( 25.63134405897505985, 139.9845197017440057, -9.403501633128708903 ) ) ;
#807=CARTESIAN_POINT ( 'NONE',  ( 6.714477151836450552, 134.0780154003031726, -13.00000000000000000 ) ) ;
#809=DIRECTION ( 'NONE',  ( 0.000000000000000000, 0.000000000000000000, 1.000000000000000000 ) ) ;
#815=LINE ( 'NONE', #15940, #707 ) ;
#820=FACE_OUTER_BOUND ( 'NONE', #4191, .T. ) ;
#821=VECTOR ( 'NONE', #4007, 1000.000000000000000 ) ;
#822=FACE_OUTER_BOUND ( 'NONE', #15885, .T. ) ;
#825=ORIENTED_EDGE ( 'NONE', *, *, #845, .T. ) ;
#829=ORIENTED_EDGE ( 'NONE', *, *, #7545, .T. ) ;
#833=CARTESIAN_POINT ( 'NONE',  ( -15.84744341939753021, 31.82541372190370055, -11.32583567006417624 ) ) ;
#835=CARTESIAN_POINT ( 'NONE',  ( 49.99999999999998579, 167.6227766016838814, -19.42820660268601074 ) ) ;
#838=CYLINDRICAL_SURFACE ( 'NONE', #7299, 5.000000000000000888 ) ;
#839=CARTESIAN_POINT ( 'NONE',  ( -26.10410744458348020, 20.00000000000000000, -13.37721135299797659 ) ) ;
#842=CARTESIAN_POINT ( 'NONE',  ( -40.00000000000000000, 4.000000000000000000, -33.00000000000000711 ) ) ;
#843=EDGE_CURVE ( 'NONE', #7078, #17487, #4766, .T. ) ;
#844=ORIENTED_EDGE ( 'NONE', *, *, #10151, .T. ) ;
#845=EDGE_CURVE ( 'NONE', #12168, #14104, #5943, .T. ) ;
#846=VERTEX_POINT ( 'NONE', #7154 ) ;
#848=ORIENTED_EDGE ( 'NONE', *, *, #17042, .F. ) ;
#852=VECTOR ( 'NONE', #2578, 1000.000000000000000 ) ;
#853=EDGE_LOOP ( 'NONE', ( #13360, #10360 ) ) ;
#858=DIRECTION ( 'NONE',  ( 0.000000000000000000, 0.000000000000000000, 1.000000000000000000 ) ) ;
#860=EDGE_LOOP ( 'NONE', ( #844, #11416 ) ) ;
#863=DIRECTION ( 'NONE',  ( 0.000000000000000000, 0.000000000000000000, -1.000000000000000000 ) ) ;
#865=ADVANCED_FACE ( 'NONE', ( #12551, #9893 ), #417, .F. ) ;
#867=CARTESIAN_POINT ( 'NONE',  ( -15.30535435590778448, 19.99999999999766587, -5.925683940270866756 ) ) ;
#874=VERTEX_POINT ( 'NONE', #7331 ) ;
#876=AXIS2_PLACEMENT_3D ( 'NONE', #4470, #9943, #1984 ) ;
#879=ORIENTED_EDGE ( 'NONE', *, *, #15983, .F. ) ;
#881=DIRECTION ( 'NONE',  ( 0.000000000000000000, 1.000000000000000000, 0.000000000000000000 ) ) ;
#884=EDGE_CURVE ( 'NONE', #11970, #4566, #15562, .T. ) ;
#885=CARTESIAN_POINT ( 'NONE',  ( 24.16572647217576275, 198.0686797691926131, -22.93241811017415088 ) ) ;
#888=ORIENTED_EDGE ( 'NONE', *, *, #11863, .T. ) ;
#889=CARTESIAN_POINT ( 'NONE',  ( 22.52789404479186786, 19.99999999999999289, -11.66574595783169954 ) ) ;
#890=CARTESIAN_POINT ( 'NONE',  ( 10.67016715011969374, 138.9541284244158419, -13.78020913810582115 ) ) ;
#894=CARTESIAN_POINT ( 'NONE',  ( 27.50000000000001066, 146.6227766016838245, -16.00000000000000000 ) ) ;
#896=DIRECTION ( 'NONE',  ( 1.000000000000000000, 0.000000000000000000, -0.000000000000000000 ) ) ;
#897=DIRECTION ( 'NONE',  ( 1.000000000000000000, 0.000000000000000000, -0.000000000000000000 ) ) ;
#898=( BOUNDED_SURFACE ( )  B_SPLINE_SURFACE ( 3, 2, ( 
 ( #1065, #3809, #6207 ),
 ( #2308, #11859, #5143 ),
 ( #9204, #14610, #2482 ),
 ( #7880, #13289, #14785 ),
 ( #2750, #13372, #9295 ),
 ( #6736, #8475, #13891 ),
 ( #1750, #7145, #13552 ),
 ( #12137, #6646, #3074 ),
 ( #15197, #4004, #16129 ),
 ( #10716, #16028, #12041 ),
 ( #7968, #4078, #6826 ),
 ( #8051, #12218, #12544 ),
 ( #5488, #10619, #410 ),
 ( #16212, #1335, #9384 ),
 ( #2659, #5320, #13461 ),
 ( #1426, #9459, #7 ),
 ( #5411, #10802, #5816 ),
 ( #14869, #8140, #89 ),
 ( #11207, #5223, #10875 ),
 ( #3908, #16294, #14705 ),
 ( #4166, #9550, #2583 ),
 ( #1239, #17446, #16102 ),
 ( #3614, #7675, #2458 ),
 ( #9003, #13170, #1132 ),
 ( #5291, #3977, #11924 ),
 ( #7756, #13084, #1216 ),
 ( #14496, #10690, #9361 ),
 ( #13262, #7947, #2364 ) ),
 .UNSPECIFIED., .F., .F., .F. ) 
 B_SPLINE_SURFACE_WITH_KNOTS ( ( 4, 2, 2, 2, 2, 2, 2, 2, 2, 2, 2, 2, 2, 4 ),
 ( 3, 3 ),
 ( 0.01342997177288655399, 0.01733910390705692070, 0.01929366997414210666, 0.02124823604122728915, 0.02515736817539765760, 0.02711193424248284356, 0.02906650030956802605, 0.03297563244373839797, 0.03493019851082358046, 0.03688476457790876295, 0.03883933064499394544, 0.03981661367853653322, 0.04079389671207912793, 0.04470302884624949985 ),
 ( 0.000000000000000000, 1.000000000000000000 ),
 .UNSPECIFIED. ) 
 GEOMETRIC_REPRESENTATION_ITEM ( )  RATIONAL_B_SPLINE_SURFACE ( (
 ( 1.000000000000000000, 0.7117435966472906994, 1.000000000000000000),
 ( 1.000000000000000000, 0.7117434842622243352, 1.000000000000000000),
 ( 1.000000000000000000, 0.7117144184577041122, 1.000000000000000000),
 ( 1.000000000000000000, 0.7116285301813174424, 1.000000000000000000),
 ( 1.000000000000000000, 0.7115928256594988843, 1.000000000000000000),
 ( 1.000000000000000000, 0.7115068832447583036, 1.000000000000000000),
 ( 1.000000000000000000, 0.7114564033772057261, 1.000000000000000000),
 ( 1.000000000000000000, 0.7112861117249480447, 1.000000000000000000),
 ( 1.000000000000000000, 0.7111469280185451769, 1.000000000000000000),
 ( 1.000000000000000000, 0.7108993804763810154, 1.000000000000000000),
 ( 1.000000000000000000, 0.7108100171490865371, 1.000000000000000000),
 ( 1.000000000000000000, 0.7106191415567553182, 1.000000000000000000),
 ( 1.000000000000000000, 0.7105185320923615988, 1.000000000000000000),
 ( 1.000000000000000000, 0.7102014790723295556, 1.000000000000000000),
 ( 1.000000000000000000, 0.7099699576740480245, 1.000000000000000000),
 ( 1.000000000000000000, 0.7095909300315041968, 1.000000000000000000),
 ( 1.000000000000000000, 0.7094593121158984106, 1.000000000000000000),
 ( 1.000000000000000000, 0.7091910831477740151, 1.000000000000000000),
 ( 1.000000000000000000, 0.7090537746377550965, 1.000000000000000000),
 ( 1.000000000000000000, 0.7087727591781153302, 1.000000000000000000),
 ( 1.000000000000000000, 0.7086290523620303317, 1.000000000000000000),
 ( 1.000000000000000000, 0.7084085592173990920, 1.000000000000000000),
 ( 1.000000000000000000, 0.7083342380281847372, 1.000000000000000000),
 ( 1.000000000000000000, 0.7081839094109132482, 1.000000000000000000),
 ( 1.000000000000000000, 0.7081077478408333015, 1.000000000000000000),
 ( 1.000000000000000000, 0.7077267031860466906, 1.000000000000000000),
 ( 1.000000000000000000, 0.7074184602291956336, 1.000000000000000000),
 ( 1.000000000000000000, 0.7071067811865476838, 1.000000000000000000) ) ) 
 REPRESENTATION_ITEM ( '' )  SURFACE ( )  );
#902=CARTESIAN_POINT ( 'NONE',  ( 28.95071320099337697, 140.7094120356993585, -16.41247553121493041 ) ) ;
#904=FACE_OUTER_BOUND ( 'NONE', #13730, .T. ) ;
#905=ORIENTED_EDGE ( 'NONE', *, *, #16605, .T. ) ;
#909=CARTESIAN_POINT ( 'NONE',  ( -80.00000000000001421, 196.6227766016838245, -12.99999999999999822 ) ) ;
#910=ADVANCED_FACE ( 'NONE', ( #609 ), #8658, .F. ) ;
#913=ORIENTED_EDGE ( 'NONE', *, *, #1538, .F. ) ;
#914=CARTESIAN_POINT ( 'NONE',  ( 48.00000000000000711, 175.6227766016838530, -19.42820660268601074 ) ) ;
#916=DIRECTION ( 'NONE',  ( 0.000000000000000000, 0.000000000000000000, 1.000000000000000000 ) ) ;
#918=CARTESIAN_POINT ( 'NONE',  ( -9.672962866393921999, 30.74839102026217574, -12.74052981562734388 ) ) ;
#919=VERTEX_POINT ( 'NONE', #8995 ) ;
#921=ORIENTED_EDGE ( 'NONE', *, *, #5460, .T. ) ;
#922=CARTESIAN_POINT ( 'NONE',  ( 36.00000000000000711, 196.6227766016838245, -24.49489742783179125 ) ) ;
#927=CARTESIAN_POINT ( 'NONE',  ( -86.08967107480829384, 151.0287754819113957, -25.78994361341036168 ) ) ;
#930=CARTESIAN_POINT ( 'NONE',  ( 15.60228996708985072, 124.9392590763940518, -1.450155947765682260E-14 ) ) ;
#931=LINE ( 'NONE', #1013, #7504 ) ;
#932=CARTESIAN_POINT ( 'NONE',  ( 25.68041636605677525, 150.8057096996395217, -28.13880055569950400 ) ) ;
#933=ADVANCED_FACE ( 'NONE', ( #1126 ), #13158, .F. ) ;
#936=CARTESIAN_POINT ( 'NONE',  ( -50.00000000000000000, 191.6227766016837961, 1.224646799147353454E-15 ) ) ;
#937=EDGE_CURVE ( 'NONE', #1279, #14899, #10582, .T. ) ;
#939=CARTESIAN_POINT ( 'NONE',  ( 48.00000000000000711, 179.6227766016838245, -12.50000337241049309 ) ) ;
#940=CARTESIAN_POINT ( 'NONE',  ( 20.22393135579957502, 29.92951751662230109, -13.49252536210626197 ) ) ;
#946=ORIENTED_EDGE ( 'NONE', *, *, #5353, .F. ) ;
#947=DIRECTION ( 'NONE',  ( 0.000000000000000000, 0.000000000000000000, -1.000000000000000000 ) ) ;
#951=CARTESIAN_POINT ( 'NONE',  ( 49.99999999999998579, 183.6227766016837961, -5.571800142134975431 ) ) ;
#952=CARTESIAN_POINT ( 'NONE',  ( 7.438682885632053932, 133.7774783946093464, -12.91151668396746111 ) ) ;
#953=ORIENTED_EDGE ( 'NONE', *, *, #16168, .T. ) ;
#954=LINE ( 'NONE', #17334, #5584 ) ;
#955=CARTESIAN_POINT ( 'NONE',  ( 0.000000000000000000, 2.000000000000000000, 0.000000000000000000 ) ) ;
#957=CARTESIAN_POINT ( 'NONE',  ( 30.55142212064656704, 202.6030615872001590, -16.28580987144873404 ) ) ;
#960=CARTESIAN_POINT ( 'NONE',  ( 14.93242934743711814, 20.00000000000000000, -24.99999999999999645 ) ) ;
#962=CARTESIAN_POINT ( 'NONE',  ( 8.038468667238035437, 139.4170824625289242, -14.76281475457819070 ) ) ;
#964=CARTESIAN_POINT ( 'NONE',  ( -76.65341708795939724, 151.6073998100962399, -28.71242994986354446 ) ) ;
#965=CARTESIAN_POINT ( 'NONE',  ( 10.58901158398830766, 139.9616134764785329, -11.54438095561596000 ) ) ;
#966=ORIENTED_EDGE ( 'NONE', *, *, #5460, .F. ) ;
#969=DIRECTION ( 'NONE',  ( -1.000000000000000000, -0.000000000000000000, -0.000000000000000000 ) ) ;
#970=FACE_OUTER_BOUND ( 'NONE', #1823, .T. ) ;
#971=VECTOR ( 'NONE', #8694, 1000.000000000000000 ) ;
#975=CARTESIAN_POINT ( 'NONE',  ( 48.00000000000000711, 151.6227766016839098, -5.571800142134973655 ) ) ;
#979=CARTESIAN_POINT ( 'NONE',  ( -27.99999999999998224, 10.00000000000000000, -35.00200000000000244 ) ) ;
#987=EDGE_CURVE ( 'NONE', #6662, #12168, #15905, .T. ) ;
#988=ORIENTED_EDGE ( 'NONE', *, *, #13000, .T. ) ;
#993=CARTESIAN_POINT ( 'NONE',  ( -12.63609539511579527, 18.00000000000000000, -24.35132453916584794 ) ) ;
#994=EDGE_CURVE ( 'NONE', #3454, #1173, #14, .T. ) ;
#997=DIRECTION ( 'NONE',  ( 0.000000000000000000, 0.000000000000000000, 1.000000000000000000 ) ) ;
#998=VECTOR ( 'NONE', #6430, 1000.000000000000000 ) ;
#1000=CARTESIAN_POINT ( 'NONE',  ( 24.96063036748655506, 193.3606217133605298, -27.43184792633611480 ) ) ;
#1003=ORIENTED_EDGE ( 'NONE', *, *, #9588, .F. ) ;
#1004=ORIENTED_EDGE ( 'NONE', *, *, #6432, .T. ) ;
#1006=CARTESIAN_POINT ( 'NONE',  ( -87.46328901163954583, 147.3890553372962700, -22.40111672564486867 ) ) ;
#1008=AXIS2_PLACEMENT_3D ( 'NONE', #5879, #5974, #474 ) ;
#1012=AXIS2_PLACEMENT_3D ( 'NONE', #2075, #11376, #7558 ) ;
#1013=CARTESIAN_POINT ( 'NONE',  ( 21.99999999999998224, 9.999999999999998224, -35.00000000000000000 ) ) ;
#1016=DIRECTION ( 'NONE',  ( 1.000000000000000000, 0.000000000000000000, -0.000000000000000000 ) ) ;
#1017=ORIENTED_EDGE ( 'NONE', *, *, #8652, .T. ) ;
#1019=CARTESIAN_POINT ( 'NONE',  ( -25.49999999999998579, 10.00000000000000000, -16.00000000000000000 ) ) ;
#1022=DIRECTION ( 'NONE',  ( 0.000000000000000000, -1.000000000000000000, -6.123233995736762338E-17 ) ) ;
#1025=AXIS2_PLACEMENT_3D ( 'NONE', #98, #12307, #8152 ) ;
#1029=DIRECTION ( 'NONE',  ( 1.000000000000000000, 0.000000000000000000, 0.000000000000000000 ) ) ;
#1030=EDGE_CURVE ( 'NONE', #160, #8896, #6960, .T. ) ;
#1031=EDGE_CURVE ( 'NONE', #9988, #1445, #13577, .T. ) ;
#1032=ADVANCED_FACE ( 'NONE', ( #10848 ), #9355, .F. ) ;
#1037=( LENGTH_UNIT ( ) NAMED_UNIT ( * ) SI_UNIT ( .MILLI., .METRE. ) );
#1040=DIRECTION ( 'NONE',  ( 1.000000000000000000, 0.000000000000000000, 0.000000000000000000 ) ) ;
#1041=CARTESIAN_POINT ( 'NONE',  ( -85.96511341109068383, 145.8838445361196818, -23.72313757307397708 ) ) ;
#1042=CIRCLE ( 'NONE', #1617, 12.00000000000000000 ) ;
#1043=CARTESIAN_POINT ( 'NONE',  ( 12.04170873690402566, 130.2202688438208327, -11.06482237631273868 ) ) ;
#1047=CARTESIAN_POINT ( 'NONE',  ( 196.0000000000000000, 179.6227766016838245, -10.00000337241049309 ) ) ;
#1053=ADVANCED_FACE ( 'NONE', ( #4053 ), #5637, .F. ) ;
#1054=AXIS2_PLACEMENT_3D ( 'NONE', #7576, #6422, #2176 ) ;
#1055=VERTEX_POINT ( 'NONE', #13520 ) ;
#1057=EDGE_CURVE ( 'NONE', #5440, #4930, #14430, .T. ) ;
#1058=CARTESIAN_POINT ( 'NONE',  ( 12.23870813552851722, 139.5070109101417302, -10.31054875319186515 ) ) ;
#1060=DIRECTION ( 'NONE',  ( 1.000000000000000000, 0.000000000000000000, 0.000000000000000000 ) ) ;
#1064=DIRECTION ( 'NONE',  ( -0.000000000000000000, -0.000000000000000000, 1.000000000000000000 ) ) ;
#1065=CARTESIAN_POINT ( 'NONE',  ( 22.93524650466160253, 29.84210526315789025, -5.000000000000003553 ) ) ;
#1067=CARTESIAN_POINT ( 'NONE',  ( -72.50000000000002842, 146.6227766016838245, -13.00000000000000000 ) ) ;
#1070=AXIS2_PLACEMENT_3D ( 'NONE', #12538, #13961, #9879 ) ;
#1071=CARTESIAN_POINT ( 'NONE',  ( -45.00000000000003553, 120.0000000000000142, -4.999999999999999112 ) ) ;
#1072=ORIENTED_EDGE ( 'NONE', *, *, #10985, .T. ) ;
#1077=DIRECTION ( 'NONE',  ( -0.000000000000000000, -0.000000000000000000, 1.000000000000000000 ) ) ;
#1078=ORIENTED_EDGE ( 'NONE', *, *, #14042, .F. ) ;
#1079=CARTESIAN_POINT ( 'NONE',  ( 48.00000000000000000, 171.6227766016838245, -15.00000337241049131 ) ) ;
#1081=ORIENTED_EDGE ( 'NONE', *, *, #7693, .F. ) ;
#1083=CARTESIAN_POINT ( 'NONE',  ( -151.9615242270660929, 171.6227766016838245, 0.000000000000000000 ) ) ;
#1084=VECTOR ( 'NONE', #3089, 1000.000000000000000 ) ;
#1088=DIRECTION ( 'NONE',  ( 0.000000000000000000, 0.000000000000000000, 1.000000000000000000 ) ) ;
#1089=CARTESIAN_POINT ( 'NONE',  ( -13.45813206906208848, 31.92660440999782523, -10.88283926110020516 ) ) ;
#1092=AXIS2_PLACEMENT_3D ( 'NONE', #293, #5694, #5962 ) ;
#1093=ORIENTED_EDGE ( 'NONE', *, *, #6614, .F. ) ;
#1094=EDGE_CURVE ( 'NONE', #9959, #11327, #2634, .T. ) ;
#1095=CARTESIAN_POINT ( 'NONE',  ( 24.58901960448729085, 194.0039740083362858, -26.91197613625888607 ) ) ;
#1096=CIRCLE ( 'NONE', #12121, 750.0000000000001137 ) ;
#1097=LINE ( 'NONE', #6676, #9215 ) ;
#1100=VERTEX_POINT ( 'NONE', #10936 ) ;
#1101=EDGE_CURVE ( 'NONE', #2967, #7107, #9049, .T. ) ;
#1102=CARTESIAN_POINT ( 'NONE',  ( -87.44048204095830101, 147.5870804700067822, -22.61345334826514630 ) ) ;
#1105=ORIENTED_EDGE ( 'NONE', *, *, #4082, .F. ) ;
#1111=CARTESIAN_POINT ( 'NONE',  ( 33.34658291204065250, 151.6073998100962399, -28.71242994986355868 ) ) ;
#1114=ORIENTED_EDGE ( 'NONE', *, *, #6133, .T. ) ;
#1116=CARTESIAN_POINT ( 'NONE',  ( 24.93507336697352628, 29.86842105263157876, -4.999999999999999112 ) ) ;
#1119=CARTESIAN_POINT ( 'NONE',  ( -17.89548297089572060, 32.23709896788771090, -7.636891392351368602 ) ) ;
#1121=CARTESIAN_POINT ( 'NONE',  ( -77.50000000000002842, 146.6227766016838245, -16.00000000000000000 ) ) ;
#1123=CIRCLE ( 'NONE', #11293, 33.00000000000000000 ) ;
#1126=FACE_OUTER_BOUND ( 'NONE', #11539, .T. ) ;
#1127=ORIENTED_EDGE ( 'NONE', *, *, #12799, .F. ) ;
#1128=CYLINDRICAL_SURFACE ( 'NONE', #12151, 2.499999999999998668 ) ;
#1129=EDGE_CURVE ( 'NONE', #15972, #15553, #1392, .T. ) ;
#1131=CARTESIAN_POINT ( 'NONE',  ( -100.0000000000000000, 201.6227766016838245, 0.000000000000000000 ) ) ;
#1132=CARTESIAN_POINT ( 'NONE',  ( 19.47274266584701508, 18.00000000000000000, -24.48069943974689266 ) ) ;
#1133=CARTESIAN_POINT ( 'NONE',  ( -74.13623385059629811, 145.1725333695280256, -22.94453145061436672 ) ) ;
#1134=AXIS2_PLACEMENT_3D ( 'NONE', #14330, #2289, #13091 ) ;
#1135=AXIS2_PLACEMENT_3D ( 'NONE', #9812, #3088, #5745 ) ;
#1140=EDGE_CURVE ( 'NONE', #11894, #1799, #5659, .T. ) ;
#1142=ORIENTED_EDGE ( 'NONE', *, *, #11588, .F. ) ;
#1143=EDGE_LOOP ( 'NONE', ( #15959, #17118, #14386, #12047, #15475, #7216, #8312 ) ) ;
#1146=CARTESIAN_POINT ( 'NONE',  ( -81.80240525860705247, 152.3499437555877591, -29.21584945930381139 ) ) ;
#1148=CARTESIAN_POINT ( 'NONE',  ( 14.24852413927196970, 138.7494242586804489, -7.288003809479805639 ) ) ;
#1149=ORIENTED_EDGE ( 'NONE', *, *, #15369, .T. ) ;
#1153=DIRECTION ( 'NONE',  ( -1.000000000000000000, 0.000000000000000000, 0.000000000000000000 ) ) ;
#1156=CARTESIAN_POINT ( 'NONE',  ( -74.00000000000002842, 146.6227766016838245, -24.49489742783179125 ) ) ;
#1160=EDGE_CURVE ( 'NONE', #5721, #668, #2888, .T. ) ;
#1161=DIRECTION ( 'NONE',  ( -1.000000000000000000, -0.000000000000000000, 0.000000000000000000 ) ) ;
#1162=EDGE_CURVE ( 'NONE', #12168, #12804, #12449, .T. ) ;
#1163=CYLINDRICAL_SURFACE ( 'NONE', #14285, 2.500000000000000444 ) ;
#1166=CARTESIAN_POINT ( 'NONE',  ( -24.80114670877660643, 19.99999999999999289, -15.70637264050929538 ) ) ;
#1167=EDGE_LOOP ( 'NONE', ( #9373, #13594, #16037, #1479, #35, #4200 ) ) ;
#1170=VERTEX_POINT ( 'NONE', #2233 ) ;
#1173=VERTEX_POINT ( 'NONE', #8548 ) ;
#1174=CARTESIAN_POINT ( 'NONE',  ( -82.50000000000002842, 146.6227766016838245, -16.00000000000000000 ) ) ;
#1177=CARTESIAN_POINT ( 'NONE',  ( 22.65282855708332121, 195.0632477915244181, -23.23525722188764675 ) ) ;
#1179=CARTESIAN_POINT ( 'NONE',  ( -12.51506868919167026, 18.00000000000000000, -7.695309128566540480 ) ) ;
#1183=CARTESIAN_POINT ( 'NONE',  ( -74.54484354042847372, 191.4518784269448588, -26.38258506112510915 ) ) ;
#1185=VERTEX_POINT ( 'NONE', #15776 ) ;
#1188=CARTESIAN_POINT ( 'NONE',  ( -86.35693927557340999, 150.6299487802827457, -25.46745035168473237 ) ) ;
#1192=CARTESIAN_POINT ( 'NONE',  ( 15.60228996707308191, 124.9392590765123998, -1.671679228207827439 ) ) ;
#1194=DIRECTION ( 'NONE',  ( 0.000000000000000000, 0.000000000000000000, 1.000000000000000000 ) ) ;
#1195=ADVANCED_FACE ( 'NONE', ( #4395 ), #492, .F. ) ;
#1196=CARTESIAN_POINT ( 'NONE',  ( 32.20193699137669086, 152.2211730668986149, -29.13124974281948809 ) ) ;
#1197=DIRECTION ( 'NONE',  ( 1.000000000000000000, 0.000000000000000000, 0.000000000000000000 ) ) ;
#1203=CARTESIAN_POINT ( 'NONE',  ( -87.50000000000004263, 146.6227766016838245, -21.54065922853802562 ) ) ;
#1205=EDGE_LOOP ( 'NONE', ( #1850, #12761, #371, #14836, #141 ) ) ;
#1206=CARTESIAN_POINT ( 'NONE',  ( -87.43684327452987759, 145.5208630140649859, -20.20962120078074165 ) ) ;
#1209=DIRECTION ( 'NONE',  ( -1.000000000000000000, 0.000000000000000000, 0.000000000000000000 ) ) ;
#1210=CARTESIAN_POINT ( 'NONE',  ( 30.00000000000001066, 146.6227766016838245, -13.00000000000000000 ) ) ;
#1216=CARTESIAN_POINT ( 'NONE',  ( 17.53546816055560953, 18.00000000000000000, -24.87355917367171187 ) ) ;
#1217=CARTESIAN_POINT ( 'NONE',  ( -76.83884856045256129, 141.5060039278119177, -17.83622402891603542 ) ) ;
#1223=DIRECTION ( 'NONE',  ( 0.000000000000000000, 0.000000000000000000, 1.000000000000000000 ) ) ;
#1226=EDGE_CURVE ( 'NONE', #3871, #7408, #17464, .T. ) ;
#1228=CARTESIAN_POINT ( 'NONE',  ( 10.91733900447607830, 142.2434614804602404, -19.02291218241819593 ) ) ;
#1231=CARTESIAN_POINT ( 'NONE',  ( 14.60960092688903700, 138.5353766997065179, -5.001077596136161318 ) ) ;
#1239=CARTESIAN_POINT ( 'NONE',  ( 17.13110662433428288, 29.95577564710725227, -12.69327266642979168 ) ) ;
#1241=DIRECTION ( 'NONE',  ( -1.000000000000000000, -0.000000000000000000, 0.000000000000000000 ) ) ;
#1242=DIRECTION ( 'NONE',  ( 0.000000000000000000, 0.000000000000000000, 1.000000000000000000 ) ) ;
#1243=DIRECTION ( 'NONE',  ( -1.000000000000000000, -0.000000000000000000, 0.000000000000000000 ) ) ;
#1245=VERTEX_POINT ( 'NONE', #7094 ) ;
#1246=CARTESIAN_POINT ( 'NONE',  ( 17.51892952578853979, 125.6677330052578014, -5.783603459598163354 ) ) ;
#1248=DIRECTION ( 'NONE',  ( 1.000000000000000000, 0.000000000000000000, 0.000000000000000000 ) ) ;
#1250=VERTEX_POINT ( 'NONE', #13649 ) ;
#1253=ADVANCED_FACE ( 'NONE', ( #4444 ), #13571, .T. ) ;
#1254=ORIENTED_EDGE ( 'NONE', *, *, #6754, .F. ) ;
#1256=CARTESIAN_POINT ( 'NONE',  ( -43.00000000000000000, 140.0000000000000000, -15.00000000000000000 ) ) ;
#1258=AXIS2_PLACEMENT_3D ( 'NONE', #13743, #7018, #2858 ) ;
#1264=CARTESIAN_POINT ( 'NONE',  ( -12.79675654462651124, 17.99999999999533529, -5.581853174322293221 ) ) ;
#1268=CARTESIAN_POINT ( 'NONE',  ( -5.000000000000000888, 154.3022685259950038, -9.999999999999900524 ) ) ;
#1272=ORIENTED_EDGE ( 'NONE', *, *, #5599, .F. ) ;
#1273=VECTOR ( 'NONE', #10193, 1000.000000000000000 ) ;
#1275=ORIENTED_EDGE ( 'NONE', *, *, #16170, .T. ) ;
#1278=EDGE_CURVE ( 'NONE', #16623, #14931, #1441, .T. ) ;
#1279=VERTEX_POINT ( 'NONE', #9735 ) ;
#1283=AXIS2_PLACEMENT_3D ( 'NONE', #13329, #1194, #11989 ) ;
#1284=CARTESIAN_POINT ( 'NONE',  ( 30.00000000000000355, 196.6227766016838245, 1.387778780781445676E-14 ) ) ;
#1285=CARTESIAN_POINT ( 'NONE',  ( -45.00000000000000000, 142.5209969267753820, -19.44444444444444997 ) ) ;
#1286=CARTESIAN_POINT ( 'NONE',  ( -27.98221281347037959, 18.00000000000000355, -4.999999999999999112 ) ) ;
#1290=AXIS2_PLACEMENT_3D ( 'NONE', #12383, #12474, #5403 ) ;
#1291=CARTESIAN_POINT ( 'NONE',  ( 23.92262868871285519, 29.88142130320016676, -9.432657661123421633 ) ) ;
#1294=ORIENTED_EDGE ( 'NONE', *, *, #176, .T. ) ;
#1295=DIRECTION ( 'NONE',  ( -1.000000000000000000, 0.000000000000000000, 0.000000000000000000 ) ) ;
#1296=EDGE_CURVE ( 'NONE', #457, #14780, #101, .T. ) ;
#1298=CARTESIAN_POINT ( 'NONE',  ( -82.50000000000002842, 146.6227766016838245, -16.00000000000000000 ) ) ;
#1299=DIRECTION ( 'NONE',  ( -1.000000000000000000, 0.000000000000000000, 0.000000000000000000 ) ) ;
#1306=B_SPLINE_CURVE_WITH_KNOTS ( 'NONE', 3,
 ( #17039, #4907, #5174, #10296, #4835, #9065, #15703, #11713, #2423, #13325, #6594, #7824, #13232, #6243, #10563, #6410, #6316, #2255, #17120, #8977, #3584, #9240, #15623, #15796, #2165, #11985, #7651, #14388, #9146, #2338, #10223, #4997, #14552, #17304, #13061, #927, #1188, #3679, #14474, #7728, #13138, #1102, #1006, #3498, #8886, #11804 ),
 .UNSPECIFIED., .F., .F.,
 ( 4, 2, 2, 2, 2, 2, 2, 2, 2, 2, 2, 2, 2, 2, 2, 2, 2, 2, 2, 2, 2, 2, 4 ),
 ( 0.01035378412632265675, 0.01206629175607497849, 0.01377879938582729849, 0.01549130701557962023, 0.01634756083045581232, 0.01720381464533200441, 0.01806006846020819651, 0.01891632227508438860, 0.02062882990483675544, 0.02148508371971293712, 0.02234133753458911881, 0.02319759134946530049, 0.02405384516434148218, 0.02576635279409380738, 0.02747886042384612565, 0.02833511423872230733, 0.02919136805359848902, 0.03090387568335084545, 0.03261638331310320188, 0.03432889094285555831, 0.03604139857260792168, 0.03689765238748409643, 0.03775390620236027117 ),
 .UNSPECIFIED. ) ;
#1307=CARTESIAN_POINT ( 'NONE',  ( -83.14994314962653732, 141.4992599418080488, -17.82476597062853685 ) ) ;
#1309=CIRCLE ( 'NONE', #7792, 6.000000000000005329 ) ;
#1310=VERTEX_POINT ( 'NONE', #4270 ) ;
#1311=DIRECTION ( 'NONE',  ( 1.000000000000000000, 0.000000000000000000, 0.000000000000000000 ) ) ;
#1314=CYLINDRICAL_SURFACE ( 'NONE', #2976, 250.0000000000000000 ) ;
#1315=ADVANCED_FACE ( 'NONE', ( #11245 ), #361, .F. ) ;
#1317=CARTESIAN_POINT ( 'NONE',  ( 15.14881438696876614, 128.6905335926829252, -10.89137921944116449 ) ) ;
#1318=EDGE_CURVE ( 'NONE', #10436, #10138, #2839, .T. ) ;
#1320=CARTESIAN_POINT ( 'NONE',  ( -78.88444202303340091, 152.5224481282687066, -29.32884290898093838 ) ) ;
#1322=CARTESIAN_POINT ( 'NONE',  ( 12.89436750745977989, 143.6582566230365501, -17.52127501928458031 ) ) ;
#1324=ORIENTED_EDGE ( 'NONE', *, *, #2716, .F. ) ;
#1327=DIRECTION ( 'NONE',  ( -0.000000000000000000, -0.000000000000000000, -1.000000000000000000 ) ) ;
#1328=EDGE_CURVE ( 'NONE', #7719, #846, #9653, .T. ) ;
#1330=AXIS2_PLACEMENT_3D ( 'NONE', #4533, #1952, #4869 ) ;
#1334=CARTESIAN_POINT ( 'NONE',  ( 19.49710218362280045, 17.99999999999999289, -24.48336163992366465 ) ) ;
#1335=CARTESIAN_POINT ( 'NONE',  ( 20.28823715622366919, 18.00000000000000000, -11.10707270023369730 ) ) ;
#1340=CARTESIAN_POINT ( 'NONE',  ( 27.40214814073310023, 141.2103550623191381, -17.32402235562967263 ) ) ;
#1341=ORIENTED_EDGE ( 'NONE', *, *, #12280, .F. ) ;
#1342=DIRECTION ( 'NONE',  ( 0.000000000000000000, 0.000000000000000000, 1.000000000000000000 ) ) ;
#1343=VECTOR ( 'NONE', #4860, 1000.000000000000000 ) ;
#1346=CARTESIAN_POINT ( 'NONE',  ( 48.00000000000000711, 179.6227766016838245, -15.00000337241049486 ) ) ;
#1347=STYLED_ITEM ( 'NONE', ( #12882 ), #17066 ) ;
#1352=DIRECTION ( 'NONE',  ( 1.000000000000000000, 0.000000000000000000, 0.000000000000000000 ) ) ;
#1353=ORIENTED_EDGE ( 'NONE', *, *, #8803, .T. ) ;
#1357=CARTESIAN_POINT ( 'NONE',  ( 37.49298393897301196, 196.2445469595302825, -21.97388680505722292 ) ) ;
#1358=CARTESIAN_POINT ( 'NONE',  ( 17.58250999373989742, 125.2198453306090045, -1.666666666666656749 ) ) ;
#1362=EDGE_CURVE ( 'NONE', #10642, #15641, #16945, .T. ) ;
#1363=ORIENTED_EDGE ( 'NONE', *, *, #15702, .F. ) ;
#1364=CARTESIAN_POINT ( 'NONE',  ( -83.07446265461977930, 189.7763206329742331, -27.55849099911373656 ) ) ;
#1367=VERTEX_POINT ( 'NONE', #16311 ) ;
#1371=AXIS2_PLACEMENT_3D ( 'NONE', #16024, #7965, #9288 ) ;
#1376=CARTESIAN_POINT ( 'NONE',  ( 48.00000000000000000, 171.6227766016838245, -12.50000337241049131 ) ) ;
#1378=CYLINDRICAL_SURFACE ( 'NONE', #9581, 7.500000000000020428 ) ;
#1383=CARTESIAN_POINT ( 'NONE',  ( -85.95768757437879515, 197.3572491277162726, -23.72357542124677110 ) ) ;
#1385=EDGE_CURVE ( 'NONE', #8108, #13207, #13001, .T. ) ;
#1386=DIRECTION ( 'NONE',  ( -1.000000000000000000, -0.000000000000000000, 0.000000000000000000 ) ) ;
#1387=EDGE_CURVE ( 'NONE', #6730, #17412, #1609, .T. ) ;
#1389=CARTESIAN_POINT ( 'NONE',  ( -80.00000000000002842, 146.6227766016838245, -16.00000000000000000 ) ) ;
#1392=LINE ( 'NONE', #8368, #6804 ) ;
#1394=ORIENTED_EDGE ( 'NONE', *, *, #564, .T. ) ;
#1395=CYLINDRICAL_SURFACE ( 'NONE', #17169, 2.499999999999998668 ) ;
#1398=( LENGTH_UNIT ( ) NAMED_UNIT ( * ) SI_UNIT ( .MILLI., .METRE. ) );
#1400=DIRECTION ( 'NONE',  ( 1.000000000000000000, 0.000000000000000000, -1.445602896647339163E-16 ) ) ;
#1409=CARTESIAN_POINT ( 'NONE',  ( 27.99999999999998224, 9.999999999999998224, -35.00200000000000244 ) ) ;
#1410=AXIS2_PLACEMENT_3D ( 'NONE', #3038, #15340, #566 ) ;
#1411=CARTESIAN_POINT ( 'NONE',  ( -27.99999999999998224, 10.00000000000000000, -13.00000000000000000 ) ) ;
#1412=CARTESIAN_POINT ( 'NONE',  ( 14.69130379018311316, 137.7259585328908713, -10.44822943247861247 ) ) ;
#1415=CARTESIAN_POINT ( 'NONE',  ( 15.45419697039644902, 125.5863960662987040, -6.086967932831932160 ) ) ;
#1416=AXIS2_PLACEMENT_3D ( 'NONE', #3060, #15359, #11113 ) ;
#1420=CYLINDRICAL_SURFACE ( 'NONE', #11309, 2.499999999999998668 ) ;
#1421=CARTESIAN_POINT ( 'NONE',  ( 48.00000000000000711, 159.6227766016838814, -3.071800142134975431 ) ) ;
#1425=CARTESIAN_POINT ( 'NONE',  ( 25.51458778375578973, 18.00000000000000000, -21.98440010584615578 ) ) ;
#1426=CARTESIAN_POINT ( 'NONE',  ( 19.16009641331746849, 29.91553747150882359, -11.79770956048753838 ) ) ;
#1427=FACE_OUTER_BOUND ( 'NONE', #12569, .T. ) ;
#1429=PLANE ( 'NONE',  #14696 ) ;
#1430=CARTESIAN_POINT ( 'NONE',  ( 28.01299615403722143, 140.9569246592376999, -16.87109569490920791 ) ) ;
#1432=LINE ( 'NONE', #14963, #6757 ) ;
#1433=VECTOR ( 'NONE', #8200, 1000.000000000000000 ) ;
#1441=LINE ( 'NONE', #10982, #5955 ) ;
#1443=CARTESIAN_POINT ( 'NONE',  ( 22.55951795904177004, 147.5870804700066685, -22.61345334826511078 ) ) ;
#1445=VERTEX_POINT ( 'NONE', #11509 ) ;
#1446=FACE_OUTER_BOUND ( 'NONE', #3207, .T. ) ;
#1447=CARTESIAN_POINT ( 'NONE',  ( -23.00000000000002132, 100.0000000000000142, -4.999999999999999112 ) ) ;
#1448=CARTESIAN_POINT ( 'NONE',  ( 17.54349574104648823, 125.4948194589026684, -4.999999999999997335 ) ) ;
#1451=ORIENTED_EDGE ( 'NONE', *, *, #15961, .F. ) ;
#1455=CARTESIAN_POINT ( 'NONE',  ( -40.00000000000000000, 4.000000000000000000, -33.00000000000000711 ) ) ;
#1457=EDGE_CURVE ( 'NONE', #1773, #6476, #6026, .T. ) ;
#1458=VECTOR ( 'NONE', #4893, 1000.000000000000000 ) ;
#1463=ORIENTED_EDGE ( 'NONE', *, *, #1965, .T. ) ;
#1467=DIRECTION ( 'NONE',  ( 0.000000000000000000, 1.000000000000000000, 0.000000000000000000 ) ) ;
#1468=CARTESIAN_POINT ( 'NONE',  ( 17.01457324639674695, 29.95810005730942649, -12.72891809691981102 ) ) ;
#1474=CARTESIAN_POINT ( 'NONE',  ( -84.99092202599167933, 199.9711820797445512, -20.53336423377503905 ) ) ;
#1475=CARTESIAN_POINT ( 'NONE',  ( 17.00000000000000000, 171.6227766016838245, 0.000000000000000000 ) ) ;
#1476=CARTESIAN_POINT ( 'NONE',  ( 34.26588824652853305, 20.00000000000000355, -10.16858984204336736 ) ) ;
#1479=ORIENTED_EDGE ( 'NONE', *, *, #2590, .F. ) ;
#1483=ORIENTED_EDGE ( 'NONE', *, *, #845, .F. ) ;
#1484=EDGE_CURVE ( 'NONE', #3419, #10551, #15402, .T. ) ;
#1485=EDGE_CURVE ( 'NONE', #17476, #8669, #11468, .T. ) ;
#1486=CARTESIAN_POINT ( 'NONE',  ( 15.96677753506825681, 136.6227766017765930, -1.239574023933634583 ) ) ;
#1489=VERTEX_POINT ( 'NONE', #13999 ) ;
#1491=DIRECTION ( 'NONE',  ( 1.000000000000000000, 0.000000000000000000, 0.000000000000000000 ) ) ;
#1495=CARTESIAN_POINT ( 'NONE',  ( 19.90854668962809626, 140.2883655178033848, -15.59737012465792461 ) ) ;
#1497=CARTESIAN_POINT ( 'NONE',  ( -27.99999999999998224, 10.00000000000000000, -16.00000000000000000 ) ) ;
#1499=ORIENTED_EDGE ( 'NONE', *, *, #13886, .T. ) ;
#1504=FACE_OUTER_BOUND ( 'NONE', #13698, .T. ) ;
#1506=CARTESIAN_POINT ( 'NONE',  ( -80.00000000000001421, 196.6227766016838245, -13.00000000000000000 ) ) ;
#1507=CARTESIAN_POINT ( 'NONE',  ( 24.50557348073514063, 144.1870492754457302, -21.73814637783849690 ) ) ;
#1509=CARTESIAN_POINT ( 'NONE',  ( -17.27091434876127707, 32.11264161353675917, -9.179609695281474302 ) ) ;
#1511=CARTESIAN_POINT ( 'NONE',  ( 196.0000000000000000, 179.6227766016838245, -12.50000337241049309 ) ) ;
#1516=CARTESIAN_POINT ( 'NONE',  ( 0.000000000000000000, 18.00000000000000355, -25.00000000000000000 ) ) ;
#1517=VERTEX_POINT ( 'NONE', #9919 ) ;
#1518=DIRECTION ( 'NONE',  ( -1.000000000000000000, 0.000000000000000000, 0.000000000000000000 ) ) ;
#1525=ORIENTED_EDGE ( 'NONE', *, *, #4841, .F. ) ;
#1526=CARTESIAN_POINT ( 'NONE',  ( -50.00000000000000000, 171.6227766016838245, -20.00000000000000355 ) ) ;
#1528=LINE ( 'NONE', #1268, #15237 ) ;
#1530=CARTESIAN_POINT ( 'NONE',  ( -9.527527117355448993, 30.70225384978374450, -12.78416694138776855 ) ) ;
#1531=ORIENTED_EDGE ( 'NONE', *, *, #11203, .F. ) ;
#1532=ORIENTED_EDGE ( 'NONE', *, *, #5703, .F. ) ;
#1534=VECTOR ( 'NONE', #15914, 1000.000000000000000 ) ;
#1535=CIRCLE ( 'NONE', #5210, 2.500000000000002220 ) ;
#1536=CARTESIAN_POINT ( 'NONE',  ( -72.50000000000000000, 196.6227766016838245, -21.54065922853802562 ) ) ;
#1538=EDGE_CURVE ( 'NONE', #3188, #13136, #6102, .T. ) ;
#1539=ORIENTED_EDGE ( 'NONE', *, *, #14098, .T. ) ;
#1550=DIRECTION ( 'NONE',  ( -0.000000000000000000, -0.000000000000000000, -1.000000000000000000 ) ) ;
#1553=FACE_OUTER_BOUND ( 'NONE', #6090, .T. ) ;
#1557=CARTESIAN_POINT ( 'NONE',  ( -68.00000000000000000, 171.6227766016838245, 0.000000000000000000 ) ) ;
#1558=ORIENTED_EDGE ( 'NONE', *, *, #17219, .F. ) ;
#1560=CIRCLE ( 'NONE', #9186, 6.000000000000008882 ) ;
#1561=VERTEX_POINT ( 'NONE', #16750 ) ;
#1566=TOROIDAL_SURFACE ( 'NONE', #3832, 25.00000000000000000, 10.00000000000000000 ) ;
#1567=CARTESIAN_POINT ( 'NONE',  ( -725.0000000000000000, 19.99999999999995737, 0.000000000000000000 ) ) ;
#1568=ORIENTED_EDGE ( 'NONE', *, *, #4182, .F. ) ;
#1572=CARTESIAN_POINT ( 'NONE',  ( 49.99999999999998579, 155.6227766016839098, -15.00000337241049486 ) ) ;
#1575=ADVANCED_FACE ( 'NONE', ( #8848 ), #117, .T. ) ;
#1578=AXIS2_PLACEMENT_3D ( 'NONE', #57, #11911, #5457 ) ;
#1579=CARTESIAN_POINT ( 'NONE',  ( 16.78995144247101123, 126.8031893778130410, -8.318227863269529010 ) ) ;
#1580=ORIENTED_EDGE ( 'NONE', *, *, #10878, .T. ) ;
#1582=CARTESIAN_POINT ( 'NONE',  ( 13.63270490666636192, 138.8028880870465969, -3.449993069226350517 ) ) ;
#1584=CARTESIAN_POINT ( 'NONE',  ( -79.76522515338450603, 190.6230697630495001, -29.39368741583861677 ) ) ;
#1587=CARTESIAN_POINT ( 'NONE',  ( -22.99999999999999645, 90.00000000000000000, 0.000000000000000000 ) ) ;
#1589=CYLINDRICAL_SURFACE ( 'NONE', #12637, 9.999999999999994671 ) ;
#1591=DIRECTION ( 'NONE',  ( -5.638339401448894059E-16, -0.000000000000000000, -1.000000000000000000 ) ) ;
#1594=FACE_BOUND ( 'NONE', #9557, .T. ) ;
#1595=EDGE_LOOP ( 'NONE', ( #13949, #10949, #5695, #10028 ) ) ;
#1596=CARTESIAN_POINT ( 'NONE',  ( -19.26597175465490963, 19.99999999999999645, -21.35691006828317384 ) ) ;
#1597=EDGE_CURVE ( 'NONE', #1517, #16267, #2739, .T. ) ;
#1599=EDGE_CURVE ( 'NONE', #2257, #15641, #8923, .T. ) ;
#1600=EDGE_LOOP ( 'NONE', ( #2861, #12870, #15823, #5940 ) ) ;
#1602=VECTOR ( 'NONE', #10888, 1000.000000000000000 ) ;
#1604=CARTESIAN_POINT ( 'NONE',  ( 22.93524650466160963, 29.84210526315773748, -15.00000000000000000 ) ) ;
#1605=VECTOR ( 'NONE', #16210, 1000.000000000000000 ) ;
#1606=ORIENTED_EDGE ( 'NONE', *, *, #13785, .T. ) ;
#1609=LINE ( 'NONE', #7008, #15259 ) ;
#1610=ORIENTED_EDGE ( 'NONE', *, *, #13821, .F. ) ;
#1611=CARTESIAN_POINT ( 'NONE',  ( 30.30638721710497663, 154.1221233254128151, -27.97726104294732608 ) ) ;
#1612=CARTESIAN_POINT ( 'NONE',  ( -21.99999999999998579, 10.00000000000000000, -35.00000000000000000 ) ) ;
#1615=CARTESIAN_POINT ( 'NONE',  ( 37.34664361473878103, 195.0609035571773404, -23.23759988234784046 ) ) ;
#1617=AXIS2_PLACEMENT_3D ( 'NONE', #9296, #13195, #13373 ) ;
#1621=DIRECTION ( 'NONE',  ( -1.000000000000000000, 0.000000000000000000, 0.000000000000000000 ) ) ;
#1622=ORIENTED_EDGE ( 'NONE', *, *, #11806, .T. ) ;
#1624=ORIENTED_EDGE ( 'NONE', *, *, #15388, .T. ) ;
#1626=LINE ( 'NONE', #12244, #17139 ) ;
#1629=EDGE_LOOP ( 'NONE', ( #3743, #16683, #6844, #9775 ) ) ;
#1637=CARTESIAN_POINT ( 'NONE',  ( 27.50000000000001066, 146.6227766016838245, 1.387778780781445676E-14 ) ) ;
#1639=CARTESIAN_POINT ( 'NONE',  ( 15.46067906867578046, 29.98929614515185804, -13.00000000000000533 ) ) ;
#1640=CARTESIAN_POINT ( 'NONE',  ( 49.99999999999998579, 167.6227766016838530, -5.571800142134975431 ) ) ;
#1642=EDGE_CURVE ( 'NONE', #4930, #5440, #7783, .T. ) ;
#1647=CARTESIAN_POINT ( 'NONE',  ( 16.25302816831168329, 19.99999999999999645, -25.00000000000000000 ) ) ;
#1649=CIRCLE ( 'NONE', #10973, 2.500000000000002220 ) ;
#1653=EDGE_CURVE ( 'NONE', #13207, #13081, #82, .T. ) ;
#1656=EDGE_CURVE ( 'NONE', #7107, #399, #16284, .T. ) ;
#1658=EDGE_LOOP ( 'NONE', ( #1744, #8467, #2560, #5454, #5419, #7001 ) ) ;
#1660=ORIENTED_EDGE ( 'NONE', *, *, #7972, .T. ) ;
#1661=CARTESIAN_POINT ( 'NONE',  ( 17.54349574104652021, 125.4948194589026684, -5.000000000000000888 ) ) ;
#1665=FACE_OUTER_BOUND ( 'NONE', #17509, .T. ) ;
#1669=FACE_OUTER_BOUND ( 'NONE', #6501, .T. ) ;
#1671=AXIS2_PLACEMENT_3D ( 'NONE', #11024, #4308, #9688 ) ;
#1672=AXIS2_PLACEMENT_3D ( 'NONE', #15684, #2507, #11883 ) ;
#1673=ADVANCED_FACE ( 'NONE', ( #162 ), #12026, .F. ) ;
#1674=CARTESIAN_POINT ( 'NONE',  ( 27.42233524417435930, 136.9585154912620908, -4.953423069178740867 ) ) ;
#1676=CARTESIAN_POINT ( 'NONE',  ( -74.00000000000005684, 147.2627523208502112, -25.14806991105193035 ) ) ;
#1678=ORIENTED_EDGE ( 'NONE', *, *, #13570, .T. ) ;
#1679=CARTESIAN_POINT ( 'NONE',  ( -81.78007429493302993, 190.8885537947572857, -29.22050223063088836 ) ) ;
#1680=CARTESIAN_POINT ( 'NONE',  ( -80.00000000000002842, 146.6227766016838245, -35.00200000000000244 ) ) ;
#1681=AXIS2_PLACEMENT_3D ( 'NONE', #8742, #863, #6079 ) ;
#1683=CIRCLE ( 'NONE', #13723, 6.000000000000008882 ) ;
#1685=AXIS2_PLACEMENT_3D ( 'NONE', #2929, #1783, #1518 ) ;
#1688=CARTESIAN_POINT ( 'NONE',  ( -100.0000000000000000, 143.9321776784423150, 5.086680500673126297E-15 ) ) ;
#1690=DIRECTION ( 'NONE',  ( 0.000000000000000000, 0.000000000000000000, 1.000000000000000000 ) ) ;
#1693=DIRECTION ( 'NONE',  ( -0.000000000000000000, -0.000000000000000000, 1.000000000000000000 ) ) ;
#1701=CARTESIAN_POINT ( 'NONE',  ( 37.50000000000001421, 197.1883573205068103, -20.88424858573644372 ) ) ;
#1703=EDGE_CURVE ( 'NONE', #15972, #8380, #13516, .T. ) ;
#1710=CARTESIAN_POINT ( 'NONE',  ( -22.99999999999998224, 10.00000000000000000, -12.99999999999999822 ) ) ;
#1711=CIRCLE ( 'NONE', #3418, 2.500000000000002220 ) ;
#1712=CARTESIAN_POINT ( 'NONE',  ( -3.000000000000000888, 154.3022685259950038, -9.999999999999900524 ) ) ;
#1713=ORIENTED_EDGE ( 'NONE', *, *, #15281, .T. ) ;
#1715=ORIENTED_EDGE ( 'NONE', *, *, #6823, .F. ) ;
#1717=CARTESIAN_POINT ( 'NONE',  ( -11.09520285051611488, 31.19962993084977398, -12.30130330100619673 ) ) ;
#1718=VERTEX_POINT ( 'NONE', #17503 ) ;
#1720=CARTESIAN_POINT ( 'NONE',  ( 34.93420767853316988, 18.00000000000000355, 0.000000000000000000 ) ) ;
#1725=ORIENTED_EDGE ( 'NONE', *, *, #15661, .T. ) ;
#1726=CARTESIAN_POINT ( 'NONE',  ( 196.0000000000000000, 179.6227766016838245, -12.50000337241049309 ) ) ;
#1727=EDGE_CURVE ( 'NONE', #1279, #14060, #14855, .T. ) ;
#1729=DIRECTION ( 'NONE',  ( 0.000000000000000000, 0.000000000000000000, 1.000000000000000000 ) ) ;
#1732=ORIENTED_EDGE ( 'NONE', *, *, #12889, .T. ) ;
#1733=CARTESIAN_POINT ( 'NONE',  ( 27.48361012698976324, 138.6227766016838245, -1.226160068396871639 ) ) ;
#1734=CIRCLE ( 'NONE', #6249, 2.499999999999998668 ) ;
#1737=FACE_OUTER_BOUND ( 'NONE', #5723, .T. ) ;
#1740=ORIENTED_EDGE ( 'NONE', *, *, #6843, .T. ) ;
#1743=ADVANCED_FACE ( 'NONE', ( #5373 ), #6520, .F. ) ;
#1744=ORIENTED_EDGE ( 'NONE', *, *, #1140, .F. ) ;
#1746=DIRECTION ( 'NONE',  ( 1.000000000000000000, 0.000000000000000000, 0.000000000000000000 ) ) ;
#1750=CARTESIAN_POINT ( 'NONE',  ( 22.42543865150203075, 29.85191494357712116, -7.821916630904659939 ) ) ;
#1751=ORIENTED_EDGE ( 'NONE', *, *, #5331, .T. ) ;
#1756=DIRECTION ( 'NONE',  ( 1.000000000000000000, 0.000000000000000000, 0.000000000000000000 ) ) ;
#1757=VERTEX_POINT ( 'NONE', #13153 ) ;
#1759=CARTESIAN_POINT ( 'NONE',  ( 30.00000000000001066, 146.6227766016838245, -35.00200000000000244 ) ) ;
#1762=CARTESIAN_POINT ( 'NONE',  ( -82.20184637777194325, 191.0369151440704343, -29.12214185324409499 ) ) ;
#1764=ADVANCED_FACE ( 'NONE', ( #14755 ), #1566, .T. ) ;
#1768=ADVANCED_FACE ( 'NONE', ( #5103 ), #17404, .F. ) ;
#1769=CARTESIAN_POINT ( 'NONE',  ( 27.50000000000000355, 196.6227766016838245, -16.00000000000000000 ) ) ;
#1770=DIRECTION ( 'NONE',  ( -1.000000000000000000, -0.000000000000000000, 0.000000000000000000 ) ) ;
#1772=FACE_BOUND ( 'NONE', #15279, .T. ) ;
#1773=VERTEX_POINT ( 'NONE', #1203 ) ;
#1775=CARTESIAN_POINT ( 'NONE',  ( -96.00000000000001421, 201.6227766016838245, 0.000000000000000000 ) ) ;
#1776=CARTESIAN_POINT ( 'NONE',  ( 30.00000000000000355, 196.6227766016838245, -13.00000000000000000 ) ) ;
#1777=ADVANCED_FACE ( 'NONE', ( #12000 ), #5275, .T. ) ;
#1783=DIRECTION ( 'NONE',  ( -0.000000000000000000, -0.000000000000000000, -1.000000000000000000 ) ) ;
#1784=LINE ( 'NONE', #1612, #17271 ) ;
#1785=CARTESIAN_POINT ( 'NONE',  ( 27.99999999999998224, 9.999999999999998224, -16.00000000000000000 ) ) ;
#1786=CARTESIAN_POINT ( 'NONE',  ( -14.99999999999998579, 90.00000000000000000, -4.999999999999999112 ) ) ;
#1791=CARTESIAN_POINT ( 'NONE',  ( 20.99355996702781724, 139.9415946336124534, -14.89340340269096785 ) ) ;
#1793=CARTESIAN_POINT ( 'NONE',  ( -72.53671098836048259, 195.8564978660713791, -22.40111672564487222 ) ) ;
#1794=EDGE_CURVE ( 'NONE', #8971, #9872, #3149, .T. ) ;
#1795=CARTESIAN_POINT ( 'NONE',  ( -13.87134331504352325, 32.05147385205248867, -10.53504704850738705 ) ) ;
#1797=ORIENTED_EDGE ( 'NONE', *, *, #12196, .F. ) ;
#1799=VERTEX_POINT ( 'NONE', #11023 ) ;
#1800=DIRECTION ( 'NONE',  ( 0.000000000000000000, 0.000000000000000000, -1.000000000000000000 ) ) ;
#1807=DIRECTION ( 'NONE',  ( -0.000000000000000000, -0.000000000000000000, -1.000000000000000000 ) ) ;
#1810=EDGE_LOOP ( 'NONE', ( #10775, #17313, #13497, #14550 ) ) ;
#1812=DIRECTION ( 'NONE',  ( 0.000000000000000000, 0.000000000000000000, 1.000000000000000000 ) ) ;
#1813=CARTESIAN_POINT ( 'NONE',  ( 29.54149365486396661, 20.00000000000000711, -18.67620474358521676 ) ) ;
#1814=PLANE ( 'NONE',  #9010 ) ;
#1815=CARTESIAN_POINT ( 'NONE',  ( -25.00000000000002132, 100.0000000000000142, -4.999999999999999112 ) ) ;
#1817=ADVANCED_FACE ( 'NONE', ( #1553 ), #12613, .F. ) ;
#1820=VERTEX_POINT ( 'NONE', #2883 ) ;
#1823=EDGE_LOOP ( 'NONE', ( #3154, #257, #5205, #13680 ) ) ;
#1826=CARTESIAN_POINT ( 'NONE',  ( 22.56315672547017925, 145.5208630140649859, -20.20962120078073454 ) ) ;
#1829=CARTESIAN_POINT ( 'NONE',  ( 36.65363293176816484, 143.1278587772777087, -16.66575456205189454 ) ) ;
#1834=DIRECTION ( 'NONE',  ( -0.000000000000000000, -0.000000000000000000, 1.000000000000000000 ) ) ;
#1837=CIRCLE ( 'NONE', #14558, 2.499999999999998668 ) ;
#1839=CIRCLE ( 'NONE', #4672, 7.500000000000007105 ) ;
#1845=LINE ( 'NONE', #12745, #6506 ) ;
#1846=ORIENTED_EDGE ( 'NONE', *, *, #1094, .T. ) ;
#1850=ORIENTED_EDGE ( 'NONE', *, *, #14310, .F. ) ;
#1851=CARTESIAN_POINT ( 'NONE',  ( -100.0000000000000000, 142.5209969267753820, -19.44444444444445352 ) ) ;
#1856=CIRCLE ( 'NONE', #11734, 2.499999999999998668 ) ;
#1861=CARTESIAN_POINT ( 'NONE',  ( 23.61360151038711308, 29.88540148010350705, -10.01045486545366181 ) ) ;
#1863=DIRECTION ( 'NONE',  ( 0.000000000000000000, 0.000000000000000000, 1.000000000000000000 ) ) ;
#1865=EDGE_CURVE ( 'NONE', #5946, #12617, #3846, .T. ) ;
#1872=VECTOR ( 'NONE', #8173, 1000.000000000000000 ) ;
#1876=DIRECTION ( 'NONE',  ( -0.000000000000000000, -1.000000000000000000, 0.000000000000000000 ) ) ;
#1878=DIRECTION ( 'NONE',  ( -1.000000000000000000, 0.000000000000000000, 0.000000000000000000 ) ) ;
#1881=CIRCLE ( 'NONE', #5844, 5.000000000000000888 ) ;
#1882=ORIENTED_EDGE ( 'NONE', *, *, #197, .T. ) ;
#1887=ORIENTED_EDGE ( 'NONE', *, *, #1457, .T. ) ;
#1891=AXIS2_PLACEMENT_3D ( 'NONE', #13371, #6643, #4336 ) ;
#1894=CIRCLE ( 'NONE', #10919, 12.00000000000000000 ) ;
#1895=DIRECTION ( 'NONE',  ( 0.000000000000000000, 1.000000000000000000, 0.000000000000000000 ) ) ;
#1896=CIRCLE ( 'NONE', #15172, 2.500000000000002220 ) ;
#1902=VERTEX_POINT ( 'NONE', #2277 ) ;
#1903=DIRECTION ( 'NONE',  ( -1.000000000000000000, 0.000000000000000000, 0.000000000000000000 ) ) ;
#1904=LINE ( 'NONE', #9686, #15577 ) ;
#1907=FACE_BOUND ( 'NONE', #613, .T. ) ;
#1909=ORIENTED_EDGE ( 'NONE', *, *, #7068, .F. ) ;
#1912=DIRECTION ( 'NONE',  ( -1.000000000000000000, -0.000000000000000000, 0.000000000000000000 ) ) ;
#1913=ORIENTED_EDGE ( 'NONE', *, *, #11163, .F. ) ;
#1915=CARTESIAN_POINT ( 'NONE',  ( 22.50000000000001421, 146.6227766016838245, -21.54065922853802562 ) ) ;
#1918=EDGE_CURVE ( 'NONE', #4489, #16184, #15822, .T. ) ;
#1920=CARTESIAN_POINT ( 'NONE',  ( 37.04838423995397534, 144.0140295085317064, -18.09598853029519105 ) ) ;
#1921=CIRCLE ( 'NONE', #9253, 2.500000000000002220 ) ;
#1922=EDGE_CURVE ( 'NONE', #3029, #13521, #6943, .T. ) ;
#1924=ORIENTED_EDGE ( 'NONE', *, *, #5514, .T. ) ;
#1927=LINE ( 'NONE', #11214, #7366 ) ;
#1928=CARTESIAN_POINT ( 'NONE',  ( -8.097611523673213796, 19.99999999997653788, -14.83628426572637693 ) ) ;
#1929=CARTESIAN_POINT ( 'NONE',  ( 36.00000000000002132, 146.6227766016838245, -24.49489742783179125 ) ) ;
#1931=DIRECTION ( 'NONE',  ( 1.000000000000000000, 0.000000000000000000, 0.000000000000000000 ) ) ;
#1933=ORIENTED_EDGE ( 'NONE', *, *, #4250, .F. ) ;
#1937=CARTESIAN_POINT ( 'NONE',  ( -86.00000000000005684, 196.3062978594714707, -24.81790219152272670 ) ) ;
#1938=FACE_OUTER_BOUND ( 'NONE', #299, .T. ) ;
#1940=ORIENTED_EDGE ( 'NONE', *, *, #11689, .T. ) ;
#1942=FACE_OUTER_BOUND ( 'NONE', #13572, .T. ) ;
#1945=CIRCLE ( 'NONE', #11827, 33.00000000000000000 ) ;
#1948=ORIENTED_EDGE ( 'NONE', *, *, #9700, .F. ) ;
#1949=CARTESIAN_POINT ( 'NONE',  ( 22.45383620668762248, 29.90040889522806111, -11.60055593449971845 ) ) ;
#1950=CARTESIAN_POINT ( 'NONE',  ( 23.20616110506447072, 140.9816209840972192, -12.26578303444138207 ) ) ;
#1951=ORIENTED_EDGE ( 'NONE', *, *, #3992, .F. ) ;
#1952=DIRECTION ( 'NONE',  ( -1.000000000000000000, -0.000000000000000000, 0.000000000000000000 ) ) ;
#1954=EDGE_LOOP ( 'NONE', ( #11743, #9542, #6065, #9181 ) ) ;
#1958=EDGE_CURVE ( 'NONE', #4419, #16184, #4351, .T. ) ;
#1965=EDGE_CURVE ( 'NONE', #11878, #1245, #15252, .T. ) ;
#1966=DIRECTION ( 'NONE',  ( -0.000000000000000000, -0.000000000000000000, -1.000000000000000000 ) ) ;
#1971=EDGE_LOOP ( 'NONE', ( #2339, #6500, #6406, #10517 ) ) ;
#1975=ORIENTED_EDGE ( 'NONE', *, *, #7736, .T. ) ;
#1981=VECTOR ( 'NONE', #15313, 1000.000000000000000 ) ;
#1984=DIRECTION ( 'NONE',  ( -1.000000000000000000, 0.000000000000000000, 0.000000000000000000 ) ) ;
#1985=CIRCLE ( 'NONE', #5948, 20.00000000000000355 ) ;
#1988=EDGE_CURVE ( 'NONE', #14929, #13466, #5112, .T. ) ;
#1991=DIRECTION ( 'NONE',  ( 0.000000000000000000, 0.000000000000000000, 1.000000000000000000 ) ) ;
#1996=DIRECTION ( 'NONE',  ( -1.000000000000000000, -0.000000000000000000, 0.000000000000000000 ) ) ;
#1997=ORIENTED_EDGE ( 'NONE', *, *, #14906, .T. ) ;
#1998=CARTESIAN_POINT ( 'NONE',  ( -72.50000000000000000, 196.6227766016838245, -35.00200000000000244 ) ) ;
#1999=LINE ( 'NONE', #585, #12329 ) ;
#2002=VERTEX_POINT ( 'NONE', #6264 ) ;
#2004=AXIS2_PLACEMENT_3D ( 'NONE', #16969, #3501, #1746 ) ;
#2007=ORIENTED_EDGE ( 'NONE', *, *, #6851, .F. ) ;
#2010=DIRECTION ( 'NONE',  ( 1.000000000000000000, 0.000000000000000000, 0.000000000000000000 ) ) ;
#2013=CARTESIAN_POINT ( 'NONE',  ( 25.00000000000000000, 196.6227766016838245, -35.00200000000000244 ) ) ;
#2014=ORIENTED_EDGE ( 'NONE', *, *, #3196, .T. ) ;
#2018=CARTESIAN_POINT ( 'NONE',  ( -17.59086657693882927, 19.99999999999999645, -22.42595686383492293 ) ) ;
#2019=CIRCLE ( 'NONE', #4851, 2.500000000000000000 ) ;
#2020=FACE_OUTER_BOUND ( 'NONE', #13499, .T. ) ;
#2022=EDGE_CURVE ( 'NONE', #1170, #5007, #4928, .T. ) ;
#2023=ADVANCED_FACE ( 'NONE', ( #13259 ), #1128, .F. ) ;
#2024=ORIENTED_EDGE ( 'NONE', *, *, #10632, .T. ) ;
#2025=CARTESIAN_POINT ( 'NONE',  ( -100.0000000000000000, 171.6227766016838245, 0.000000000000000000 ) ) ;
#2028=DIRECTION ( 'NONE',  ( 0.8660254037844378194, -0.5000000000000015543, -0.000000000000000000 ) ) ;
#2029=DIRECTION ( 'NONE',  ( 0.000000000000000000, 1.000000000000000000, 0.000000000000000000 ) ) ;
#2033=CARTESIAN_POINT ( 'NONE',  ( 196.0000000000000000, 175.6227766016838530, -21.92820660268601074 ) ) ;
#2034=CARTESIAN_POINT ( 'NONE',  ( 32.00249589297860808, 202.2831825963720007, -16.88100368216889180 ) ) ;
#2036=( BOUNDED_CURVE ( )  B_SPLINE_CURVE ( 3, ( #15011, #2884, #8276, #13685 ),
 .UNSPECIFIED., .F., .F. ) 
 B_SPLINE_CURVE_WITH_KNOTS ( ( 4, 4 ),
 ( -8.881784197001252323E-16, 1.570796326794898556 ),
 .UNSPECIFIED. ) 
 CURVE ( )  GEOMETRIC_REPRESENTATION_ITEM ( )  RATIONAL_B_SPLINE_CURVE ( ( 1.000000000000000000, 0.8047378541243643824, 0.8047378541243643824, 1.000000000000000000 ) ) 
 REPRESENTATION_ITEM ( '' )  );
#2038=CARTESIAN_POINT ( 'NONE',  ( 17.53130567297317910, 19.99999999999999289, -14.69383831151754727 ) ) ;
#2039=CARTESIAN_POINT ( 'NONE',  ( 24.26130280265436667, 140.5733633045254578, -11.19213049117091785 ) ) ;
#2042=FACE_OUTER_BOUND ( 'NONE', #14630, .T. ) ;
#2043=CARTESIAN_POINT ( 'NONE',  ( -27.99999999999998224, 10.00000000000000000, 0.000000000000000000 ) ) ;
#2048=CARTESIAN_POINT ( 'NONE',  ( 30.00000000000000355, 196.6227766016838245, -35.00000000000000000 ) ) ;
#2050=DIRECTION ( 'NONE',  ( -1.156482317317868274E-16, 1.000000000000000000, 0.000000000000000000 ) ) ;
#2051=CARTESIAN_POINT ( 'NONE',  ( 34.07201977579011043, 142.2001748967346657, -18.96071578072433184 ) ) ;
#2052=ORIENTED_EDGE ( 'NONE', *, *, #13053, .F. ) ;
#2057=CYLINDRICAL_SURFACE ( 'NONE', #12618, 5.000000000000004441 ) ;
#2065=CARTESIAN_POINT ( 'NONE',  ( -8.730345434444062747, 30.30576128541687453, -14.94291915632153334 ) ) ;
#2066=CARTESIAN_POINT ( 'NONE',  ( -45.00000000000000000, 136.6227766016838245, 0.000000000000000000 ) ) ;
#2069=ORIENTED_EDGE ( 'NONE', *, *, #1865, .F. ) ;
#2071=CARTESIAN_POINT ( 'NONE',  ( -21.35874126517689930, 20.00000000000000000, -19.71585776365618869 ) ) ;
#2073=EDGE_CURVE ( 'NONE', #919, #14342, #2530, .T. ) ;
#2075=CARTESIAN_POINT ( 'NONE',  ( 30.00000000000001066, 146.6227766016838245, -13.00000000000000000 ) ) ;
#2076=ORIENTED_EDGE ( 'NONE', *, *, #2779, .F. ) ;
#2077=EDGE_LOOP ( 'NONE', ( #16454, #10005, #10809, #13155, #15622, #14602, #921 ) ) ;
#2079=EDGE_CURVE ( 'NONE', #16820, #5595, #3132, .T. ) ;
#2083=CARTESIAN_POINT ( 'NONE',  ( 24.40238044657793992, 141.6105225557631115, -13.74486639216963368 ) ) ;
#2087=ORIENTED_EDGE ( 'NONE', *, *, #15388, .F. ) ;
#2089=CARTESIAN_POINT ( 'NONE',  ( 27.50000000000001066, 146.6227766016838245, -16.00000000000000000 ) ) ;
#2090=DIRECTION ( 'NONE',  ( -0.000000000000000000, -0.000000000000000000, -1.000000000000000000 ) ) ;
#2091=B_SPLINE_CURVE_WITH_KNOTS ( 'NONE', 3,
 ( #9558, #1246, #6653, #9209, #4011, #13, #17453, #7886, #6746, #14616, #13559, #6566, #15943, #12224, #3916, #13467, #5495, #4172, #5418, #16034, #95, #12142 ),
 .UNSPECIFIED., .F., .F.,
 ( 4, 2, 2, 2, 2, 2, 2, 2, 2, 2, 4 ),
 ( 0.000000000000000000, 0.002375333402909271790, 0.004750666805818540978, 0.007126000208727810599, 0.009501333611637081955, 0.01068900031309169378, 0.01187666701454630908, 0.01425200041745553273, 0.01543966711891012200, 0.01662733382036471128, 0.01900266722327392452 ),
 .UNSPECIFIED. ) ;
#2092=CARTESIAN_POINT ( 'NONE',  ( -14.24512928960374225, 19.99999999999770139, -9.752520130898352235 ) ) ;
#2100=CARTESIAN_POINT ( 'NONE',  ( 48.00000000000000711, 191.6227766016837677, -3.071800142134975431 ) ) ;
#2101=AXIS2_PLACEMENT_3D ( 'NONE', #11436, #7542, #11616 ) ;
#2103=PLANE ( 'NONE',  #7180 ) ;
#2109=FACE_OUTER_BOUND ( 'NONE', #16606, .T. ) ;
#2110=CARTESIAN_POINT ( 'NONE',  ( 27.60418301405396235, 202.1282835878848800, -17.15932559113868905 ) ) ;
#2112=ORIENTED_EDGE ( 'NONE', *, *, #4056, .T. ) ;
#2114=ORIENTED_EDGE ( 'NONE', *, *, #7525, .F. ) ;
#2115=CARTESIAN_POINT ( 'NONE',  ( 19.08196460475218714, 19.99999999999773337, -14.16502029867040235 ) ) ;
#2119=CARTESIAN_POINT ( 'NONE',  ( 6.134011831684059501, 140.6204725398426092, -12.99999999999999822 ) ) ;
#2120=ORIENTED_EDGE ( 'NONE', *, *, #1162, .F. ) ;
#2121=DIRECTION ( 'NONE',  ( 1.000000000000000000, 0.000000000000000000, -0.000000000000000000 ) ) ;
#2123=AXIS2_PLACEMENT_3D ( 'NONE', #9388, #10806, #4260 ) ;
#2124=AXIS2_PLACEMENT_3D ( 'NONE', #8738, #12629, #5732 ) ;
#2125=CARTESIAN_POINT ( 'NONE',  ( -87.50000000000004263, 146.6227766016838245, -13.00000000000000000 ) ) ;
#2128=ADVANCED_FACE ( 'NONE', ( #8344 ), #464, .F. ) ;
#2133=CARTESIAN_POINT ( 'NONE',  ( -27.99999999999998224, 10.00000000000000000, -35.00000000000000000 ) ) ;
#2135=DIRECTION ( 'NONE',  ( 0.000000000000000000, 0.000000000000000000, -1.000000000000000000 ) ) ;
#2136=VERTEX_POINT ( 'NONE', #13938 ) ;
#2137=CARTESIAN_POINT ( 'NONE',  ( 196.0000000000000000, 187.6227766016837961, -15.00000337241049486 ) ) ;
#2138=VECTOR ( 'NONE', #8112, 1000.000000000000000 ) ;
#2145=EDGE_CURVE ( 'NONE', #1902, #17455, #2219, .T. ) ;
#2149=CARTESIAN_POINT ( 'NONE',  ( -9.725435201701724708, 30.52647059548997888, -14.77261045527475147 ) ) ;
#2152=DIRECTION ( 'NONE',  ( 0.000000000000000000, 0.000000000000000000, 1.000000000000000000 ) ) ;
#2154=CARTESIAN_POINT ( 'NONE',  ( -7.379000772444994638, 30.00000000000000000, -15.00000000000000000 ) ) ;
#2155=CARTESIAN_POINT ( 'NONE',  ( -25.81010901361623056, 20.00000000000000000, -13.97188021846430850 ) ) ;
#2159=EDGE_LOOP ( 'NONE', ( #192, #9491, #3409, #5257, #559 ) ) ;
#2160=ORIENTED_EDGE ( 'NONE', *, *, #9048, .T. ) ;
#2163=CIRCLE ( 'NONE', #3012, 35.00000000000000000 ) ;
#2165=CARTESIAN_POINT ( 'NONE',  ( -79.69361278289508732, 154.1221233254128720, -27.97726104294734029 ) ) ;
#2171=DIRECTION ( 'NONE',  ( -1.156482317317868274E-16, 1.000000000000000000, 0.000000000000000000 ) ) ;
#2174=CARTESIAN_POINT ( 'NONE',  ( 48.00000000000000711, 179.6227766016838245, -12.50000337241049309 ) ) ;
#2175=ORIENTED_EDGE ( 'NONE', *, *, #5274, .F. ) ;
#2176=DIRECTION ( 'NONE',  ( 0.000000000000000000, 0.000000000000000000, 1.000000000000000000 ) ) ;
#2178=CIRCLE ( 'NONE', #6713, 6.000000000000005329 ) ;
#2182=ADVANCED_FACE ( 'NONE', ( #2767 ), #7800, .T. ) ;
#2187=EDGE_LOOP ( 'NONE', ( #14896, #16863, #4548, #13228 ) ) ;
#2197=DIRECTION ( 'NONE',  ( 1.000000000000000000, 0.000000000000000000, -0.000000000000000000 ) ) ;
#2198=DIRECTION ( 'NONE',  ( 0.000000000000000000, -0.4999999999999952816, 0.8660254037844413721 ) ) ;
#2202=AXIS2_PLACEMENT_3D ( 'NONE', #17296, #5166, #15531 ) ;
#2204=CARTESIAN_POINT ( 'NONE',  ( 19.47274266584531333, 19.99999999999999645, -24.48069943974461538 ) ) ;
#2212=EDGE_CURVE ( 'NONE', #3871, #2837, #9312, .T. ) ;
#2213=DIRECTION ( 'NONE',  ( 1.000000000000000000, 0.000000000000000000, 0.000000000000000000 ) ) ;
#2214=AXIS2_PLACEMENT_3D ( 'NONE', #3386, #7619, #14523 ) ;
#2215=VECTOR ( 'NONE', #2028, 1000.000000000000000 ) ;
#2219=B_SPLINE_CURVE_WITH_KNOTS ( 'NONE', 3,
 ( #1536, #6934, #16431, #4293, #9672, #12860, #3656, #16769, #3398, #8864 ),
 .UNSPECIFIED., .F., .F.,
 ( 4, 2, 2, 2, 4 ),
 ( 0.03775390620236033362, 0.04033669301524714368, 0.04291947982813395374, 0.04550226664102076379, 0.04808505345390757385 ),
 .UNSPECIFIED. ) ;
#2221=CARTESIAN_POINT ( 'NONE',  ( 30.67194674767677753, 140.6591056634353549, -16.31724425057294070 ) ) ;
#2223=LINE ( 'NONE', #12944, #11262 ) ;
#2225=LINE ( 'NONE', #12854, #3091 ) ;
#2233=CARTESIAN_POINT ( 'NONE',  ( -43.00000000000003553, 134.2062027339443944, -13.00000000000000000 ) ) ;
#2234=EDGE_CURVE ( 'NONE', #17297, #2257, #15871, .T. ) ;
#2235=EDGE_CURVE ( 'NONE', #14130, #4871, #3742, .T. ) ;
#2237=EDGE_CURVE ( 'NONE', #15620, #3735, #12426, .T. ) ;
#2239=DIRECTION ( 'NONE',  ( 0.000000000000000000, 0.000000000000000000, -1.000000000000000000 ) ) ;
#2242=CARTESIAN_POINT ( 'NONE',  ( -10.05507621332305668, 30.59909908010286372, -14.70163937327580328 ) ) ;
#2244=CARTESIAN_POINT ( 'NONE',  ( -16.41264213764166513, 18.00000000000000000, -23.02790928165778794 ) ) ;
#2247=ORIENTED_EDGE ( 'NONE', *, *, #5384, .T. ) ;
#2248=CARTESIAN_POINT ( 'NONE',  ( 31.79926070065823041, 190.8809388003084280, -29.22564348704268511 ) ) ;
#2249=FACE_BOUND ( 'NONE', #13044, .T. ) ;
#2255=CARTESIAN_POINT ( 'NONE',  ( -76.92553734538029175, 153.4692325703934728, -27.55849099911372946 ) ) ;
#2257=VERTEX_POINT ( 'NONE', #6758 ) ;
#2261=LINE ( 'NONE', #17395, #13838 ) ;
#2262=DIRECTION ( 'NONE',  ( -1.000000000000000000, -0.000000000000000000, 0.000000000000000000 ) ) ;
#2264=EDGE_LOOP ( 'NONE', ( #516, #5165, #2426, #7820 ) ) ;
#2266=VECTOR ( 'NONE', #1756, 1000.000000000000000 ) ;
#2267=AXIS2_PLACEMENT_3D ( 'NONE', #1409, #16276, #6629 ) ;
#2271=VERTEX_POINT ( 'NONE', #1174 ) ;
#2273=ADVANCED_FACE ( 'NONE', ( #7985 ), #13386, .T. ) ;
#2277=CARTESIAN_POINT ( 'NONE',  ( -72.50000000000000000, 196.6227766016838245, -21.54065922853802562 ) ) ;
#2281=B_SPLINE_CURVE_WITH_KNOTS ( 'NONE', 3,
 ( #6926, #5350, #3942, #204, #9409, #8257, #13492, #6855, #10999, #9666, #5519, #14812, #5610, #11978, #6771, #16061, #8335, #1364, #16157, #12331, #16238, #5252, #12243, #10655, #38, #5437, #115, #16421, #14736, #9323, #4285, #10828, #14900, #8171, #1183, #6588, #17379, #2609, #7994, #15336, #15152, #295, #1793, #11167, #16586, #10008 ),
 .UNSPECIFIED., .F., .F.,
 ( 4, 2, 2, 2, 2, 2, 2, 2, 2, 2, 2, 2, 2, 2, 2, 2, 2, 2, 2, 2, 2, 2, 4 ),
 ( 0.01035378412632265502, 0.01206629175607501145, 0.01377879938582736614, 0.01549130701557972084, 0.01634756083045589559, 0.01720381464533207033, 0.01806006846020824508, 0.01891632227508441982, 0.02062882990483679013, 0.02148508371971297182, 0.02234133753458915350, 0.02319759134946533866, 0.02405384516434152381, 0.02576635279409384555, 0.02747886042384617075, 0.02833511423872235591, 0.02919136805359853412, 0.03090387568335089402, 0.03261638331310325739, 0.03432889094285561382, 0.03604139857260797719, 0.03689765238748415888, 0.03775390620236033362 ),
 .UNSPECIFIED. ) ;
#2282=AXIS2_PLACEMENT_3D ( 'NONE', #5784, #9767, #16689 ) ;
#2283=DIRECTION ( 'NONE',  ( 0.000000000000000000, 0.000000000000000000, -1.000000000000000000 ) ) ;
#2284=CARTESIAN_POINT ( 'NONE',  ( -77.39307936938270416, 141.2146784997055704, -17.33162689407163271 ) ) ;
#2285=CARTESIAN_POINT ( 'NONE',  ( 49.99999999999998579, 171.6227766016838245, -10.00000337241048953 ) ) ;
#2287=CYLINDRICAL_SURFACE ( 'NONE', #8127, 11.99999999999999645 ) ;
#2288=PLANE ( 'NONE',  #3649 ) ;
#2289=DIRECTION ( 'NONE',  ( -1.000000000000000000, -0.000000000000000000, -0.000000000000000000 ) ) ;
#2290=CARTESIAN_POINT ( 'NONE',  ( 26.52485666266940711, 201.5283731665715834, -18.18938113080312391 ) ) ;
#2293=VERTEX_POINT ( 'NONE', #12154 ) ;
#2294=EDGE_CURVE ( 'NONE', #15865, #14137, #11855, .T. ) ;
#2295=CARTESIAN_POINT ( 'NONE',  ( 16.23725950538873164, 20.00000000000000000, -24.99999999984155252 ) ) ;
#2296=CARTESIAN_POINT ( 'NONE',  ( 12.26645298401004425, 138.5600601684519120, -12.85897773338031946 ) ) ;
#2298=CARTESIAN_POINT ( 'NONE',  ( -77.01821113640596650, 151.8338245663404678, -28.86895077895843542 ) ) ;
#2299=CARTESIAN_POINT ( 'NONE',  ( 10.91733900447548322, 143.9222794873857652, -17.93588862913478366 ) ) ;
#2300=ADVANCED_FACE ( 'NONE', ( #13921 ), #15238, .F. ) ;
#2304=EDGE_CURVE ( 'NONE', #4489, #453, #4357, .T. ) ;
#2308=CARTESIAN_POINT ( 'NONE',  ( 22.93524650466135739, 29.84210526317653489, -5.528689893908154573 ) ) ;
#2311=DIRECTION ( 'NONE',  ( 1.000000000000000000, 0.000000000000000000, 0.000000000000000000 ) ) ;
#2314=EDGE_CURVE ( 'NONE', #14544, #10995, #3072, .T. ) ;
#2315=EDGE_LOOP ( 'NONE', ( #13827, #3262, #5910, #7155, #15380, #5304 ) ) ;
#2316=CARTESIAN_POINT ( 'NONE',  ( -80.00000000000001421, 196.6227766016838245, -35.00200000000000244 ) ) ;
#2318=ORIENTED_EDGE ( 'NONE', *, *, #7734, .F. ) ;
#2323=DIRECTION ( 'NONE',  ( -1.000000000000000000, -0.000000000000000000, -0.000000000000000000 ) ) ;
#2326=CARTESIAN_POINT ( 'NONE',  ( -9.480043248728311056, 17.99999999999769784, -11.96743332394513715 ) ) ;
#2330=ADVANCED_FACE ( 'NONE', ( #14094 ), #5951, .T. ) ;
#2333=CARTESIAN_POINT ( 'NONE',  ( -22.99999999999999289, 120.0000000000000142, 0.000000000000000000 ) ) ;
#2337=EDGE_LOOP ( 'NONE', ( #4983, #602, #8567, #12974 ) ) ;
#2338=CARTESIAN_POINT ( 'NONE',  ( -83.54345905997189448, 153.2387635573000750, -27.40528370530128299 ) ) ;
#2339=ORIENTED_EDGE ( 'NONE', *, *, #14502, .F. ) ;
#2343=CARTESIAN_POINT ( 'NONE',  ( 37.50000000000000711, 146.6227766016838245, -21.54065922853802562 ) ) ;
#2348=CARTESIAN_POINT ( 'NONE',  ( 18.77390920412167929, 29.94862569121198348, -14.25030649093772972 ) ) ;
#2349=EDGE_CURVE ( 'NONE', #13323, #6602, #10155, .T. ) ;
#2350=ADVANCED_FACE ( 'NONE', ( #6028, #10348 ), #6283, .F. ) ;
#2351=DIRECTION ( 'NONE',  ( -1.000000000000000000, 0.000000000000000000, 0.000000000000000000 ) ) ;
#2353=CARTESIAN_POINT ( 'NONE',  ( 17.00000000000000000, 206.6227766016838245, 2.143131898507868248E-15 ) ) ;
#2355=EDGE_LOOP ( 'NONE', ( #14326, #11383, #6376, #8501 ) ) ;
#2359=PLANE ( 'NONE',  #14622 ) ;
#2364=CARTESIAN_POINT ( 'NONE',  ( 14.93242934743710570, 18.00000000000000000, -25.00000000000000000 ) ) ;
#2365=LINE ( 'NONE', #3883, #4770 ) ;
#2368=EDGE_LOOP ( 'NONE', ( #953, #11410 ) ) ;
#2369=CARTESIAN_POINT ( 'NONE',  ( -27.98221281347037959, 30.00000000000000000, -15.00000000000000000 ) ) ;
#2371=CARTESIAN_POINT ( 'NONE',  ( -50.00000000000000000, 171.6227766016838245, 0.000000000000000000 ) ) ;
#2372=CARTESIAN_POINT ( 'NONE',  ( 31.06650171500291790, 202.5285685493725794, -16.42664996635052432 ) ) ;
#2374=ORIENTED_EDGE ( 'NONE', *, *, #9161, .T. ) ;
#2378=DIRECTION ( 'NONE',  ( -0.000000000000000000, -0.000000000000000000, 1.000000000000000000 ) ) ;
#2379=CARTESIAN_POINT ( 'NONE',  ( 13.00433657606611604, 139.2454419355441928, -9.442801289195550396 ) ) ;
#2380=ORIENTED_EDGE ( 'NONE', *, *, #3707, .F. ) ;
#2385=ADVANCED_FACE ( 'NONE', ( #4872, #7522 ), #546, .T. ) ;
#2392=CARTESIAN_POINT ( 'NONE',  ( 34.78805733343664741, 142.9896906294144969, -20.13387259562453480 ) ) ;
#2397=LINE ( 'NONE', #2137, #12148 ) ;
#2400=EDGE_LOOP ( 'NONE', ( #9524, #14647 ) ) ;
#2407=AXIS2_PLACEMENT_3D ( 'NONE', #7831, #3428, #8894 ) ;
#2410=CARTESIAN_POINT ( 'NONE',  ( 48.00000000000000711, 183.6227766016837961, -3.071800142134975431 ) ) ;
#2411=CARTESIAN_POINT ( 'NONE',  ( -17.03105419742079363, 32.06459626301238330, -9.633022903854756791 ) ) ;
#2412=CARTESIAN_POINT ( 'NONE',  ( -12.73428483635692210, 18.00000000000460787, -6.504128904294631752 ) ) ;
#2414=VERTEX_POINT ( 'NONE', #4953 ) ;
#2418=CARTESIAN_POINT ( 'NONE',  ( 34.02269566797333056, 192.1516832787069404, -28.34894355864044613 ) ) ;
#2421=ORIENTED_EDGE ( 'NONE', *, *, #7525, .T. ) ;
#2423=CARTESIAN_POINT ( 'NONE',  ( -73.65095110843941484, 150.6223998522366401, -25.45681811525069804 ) ) ;
#2425=AXIS2_PLACEMENT_3D ( 'NONE', #2873, #8268, #13676 ) ;
#2426=ORIENTED_EDGE ( 'NONE', *, *, #671, .T. ) ;
#2428=CARTESIAN_POINT ( 'NONE',  ( 13.66341101666136382, 138.6227766017534293, -1.153153160029659841 ) ) ;
#2431=CARTESIAN_POINT ( 'NONE',  ( 30.20986408795699418, 152.6234490708242220, -29.39431159376453095 ) ) ;
#2435=ORIENTED_EDGE ( 'NONE', *, *, #12533, .F. ) ;
#2440=LINE ( 'NONE', #2353, #8732 ) ;
#2443=CIRCLE ( 'NONE', #14599, 7.500000000000000000 ) ;
#2445=CIRCLE ( 'NONE', #16307, 5.000000000000000888 ) ;
#2448=ORIENTED_EDGE ( 'NONE', *, *, #13761, .F. ) ;
#2456=ADVANCED_FACE ( 'NONE', ( #717, #6114 ), #11511, .F. ) ;
#2458=CARTESIAN_POINT ( 'NONE',  ( 20.11141720500412333, 18.00000000000000000, -24.32074799214299077 ) ) ;
#2459=CARTESIAN_POINT ( 'NONE',  ( -74.00000000000002842, 146.6227766016838245, -24.49489742783179125 ) ) ;
#2460=AXIS2_PLACEMENT_3D ( 'NONE', #8576, #7506, #8495 ) ;
#2468=CARTESIAN_POINT ( 'NONE',  ( 35.74205400282647815, 198.3976433773784152, -22.54711430683565254 ) ) ;
#2471=CARTESIAN_POINT ( 'NONE',  ( 8.608950980928550933, 133.4921716645119432, -14.72901497434506091 ) ) ;
#2474=CARTESIAN_POINT ( 'NONE',  ( -84.31958363394323897, 150.8057096996395785, -28.13880055569950400 ) ) ;
#2476=CARTESIAN_POINT ( 'NONE',  ( 13.85534145189780197, 143.5014890223674229, -17.26861023069377410 ) ) ;
#2480=LINE ( 'NONE', #7877, #4714 ) ;
#2482=CARTESIAN_POINT ( 'NONE',  ( 34.80444759354871564, 18.00000000000000000, -7.621511755358874929 ) ) ;
#2483=DIRECTION ( 'NONE',  ( 1.000000000000000000, -1.243449787580175325E-14, 0.000000000000000000 ) ) ;
#2484=CYLINDRICAL_SURFACE ( 'NONE', #17506, 2.500000000000000444 ) ;
#2486=VECTOR ( 'NONE', #6462, 1000.000000000000000 ) ;
#2491=CARTESIAN_POINT ( 'NONE',  ( -25.15885279626527193, 20.00000000000000355, -15.13659797665870776 ) ) ;
#2496=ADVANCED_FACE ( 'NONE', ( #13189 ), #14781, .T. ) ;
#2497=ORIENTED_EDGE ( 'NONE', *, *, #12512, .F. ) ;
#2503=VECTOR ( 'NONE', #5389, 1000.000000000000114 ) ;
#2504=EDGE_LOOP ( 'NONE', ( #10553, #11632 ) ) ;
#2507=DIRECTION ( 'NONE',  ( 0.000000000000000000, 0.000000000000000000, 1.000000000000000000 ) ) ;
#2508=DIRECTION ( 'NONE',  ( 0.000000000000000000, 0.000000000000000000, 1.000000000000000000 ) ) ;
#2509=CARTESIAN_POINT ( 'NONE',  ( -13.91527097789399292, 18.00000000000000000, -23.98152295253420618 ) ) ;
#2510=EDGE_LOOP ( 'NONE', ( #15619, #16735, #9470, #1525 ) ) ;
#2516=CARTESIAN_POINT ( 'NONE',  ( -87.50000000000005684, 197.1893936856112362, -20.88304578468306616 ) ) ;
#2517=ORIENTED_EDGE ( 'NONE', *, *, #12004, .T. ) ;
#2518=EDGE_LOOP ( 'NONE', ( #5778, #8527, #8409, #3295, #5549, #10328, #13109, #13182, #5802, #8393 ) ) ;
#2519=EDGE_LOOP ( 'NONE', ( #17207, #12810, #15335, #13234 ) ) ;
#2522=AXIS2_PLACEMENT_3D ( 'NONE', #5850, #6839, #2849 ) ;
#2525=ORIENTED_EDGE ( 'NONE', *, *, #3118, .T. ) ;
#2528=FACE_OUTER_BOUND ( 'NONE', #2510, .T. ) ;
#2530=CIRCLE ( 'NONE', #8469, 20.00000000000000355 ) ;
#2537=DIRECTION ( 'NONE',  ( 1.000000000000000000, 0.000000000000000000, -0.000000000000000000 ) ) ;
#2539=DIRECTION ( 'NONE',  ( -0.000000000000000000, -0.000000000000000000, 1.000000000000000000 ) ) ;
#2540=DIRECTION ( 'NONE',  ( 0.000000000000000000, -8.673617379884035472E-17, -1.000000000000000000 ) ) ;
#2542=ORIENTED_EDGE ( 'NONE', *, *, #197, .F. ) ;
#2544=VECTOR ( 'NONE', #16275, 1000.000000000000114 ) ;
#2545=EDGE_CURVE ( 'NONE', #10551, #6443, #4251, .T. ) ;
#2546=AXIS2_PLACEMENT_3D ( 'NONE', #282, #444, #5594 ) ;
#2551=EDGE_LOOP ( 'NONE', ( #10113, #15537, #14761, #2542 ) ) ;
#2554=CARTESIAN_POINT ( 'NONE',  ( 15.00000000000000000, 143.0344144757318929, -16.50549856913627877 ) ) ;
#2556=CARTESIAN_POINT ( 'NONE',  ( -74.00000000000002842, 145.8714137932802544, -23.72804097270956802 ) ) ;
#2560=ORIENTED_EDGE ( 'NONE', *, *, #12281, .T. ) ;
#2561=CARTESIAN_POINT ( 'NONE',  ( 40.00000000000000711, 171.6227766016838245, 0.000000000000000000 ) ) ;
#2568=ORIENTED_EDGE ( 'NONE', *, *, #1094, .F. ) ;
#2571=CARTESIAN_POINT ( 'NONE',  ( 9.380362127004868711, 139.2112497869900949, -14.33999639901018242 ) ) ;
#2573=CARTESIAN_POINT ( 'NONE',  ( -84.03010877036541615, 151.0873486859324828, -28.34424093584476623 ) ) ;
#2574=CIRCLE ( 'NONE', #2004, 7.500000000000000000 ) ;
#2575=CARTESIAN_POINT ( 'NONE',  ( 24.34257225596280350, 140.5456842492515932, -11.13195485280035513 ) ) ;
#2578=DIRECTION ( 'NONE',  ( -0.000000000000000000, -0.000000000000000000, -1.000000000000000000 ) ) ;
#2581=DIRECTION ( 'NONE',  ( -1.000000000000000000, 0.000000000000000000, 0.000000000000000000 ) ) ;
#2583=CARTESIAN_POINT ( 'NONE',  ( 21.36708699129047773, 18.00000000000000000, -23.94811280430834088 ) ) ;
#2587=FACE_OUTER_BOUND ( 'NONE', #180, .T. ) ;
#2588=ORIENTED_EDGE ( 'NONE', *, *, #6679, .F. ) ;
#2590=EDGE_CURVE ( 'NONE', #4871, #8198, #7069, .T. ) ;
#2594=ORIENTED_EDGE ( 'NONE', *, *, #4717, .T. ) ;
#2599=CARTESIAN_POINT ( 'NONE',  ( -725.0000000000000000, 30.00000000000000000, -13.00000000000000000 ) ) ;
#2604=CARTESIAN_POINT ( 'NONE',  ( -11.94789857657465681, 18.00000000000115108, -9.192893430571174918 ) ) ;
#2609=CARTESIAN_POINT ( 'NONE',  ( -73.19504936680527862, 193.4351830419512623, -24.76910924193871466 ) ) ;
#2611=( BOUNDED_SURFACE ( )  B_SPLINE_SURFACE ( 3, 2, ( 
 ( #9823, #16659, #4528 ),
 ( #9914, #7003, #355 ),
 ( #4611, #16399, #3104 ),
 ( #9646, #9989, #12399 ),
 ( #7170, #537, #12570 ),
 ( #436, #11337, #15398 ),
 ( #4265, #271, #5842 ),
 ( #5677, #12660, #8677 ),
 ( #1861, #14087, #15317 ),
 ( #16480, #3190, #7258 ),
 ( #15129, #5942, #3276 ),
 ( #1949, #889, #15489 ),
 ( #15579, #8843, #13014 ),
 ( #4945, #11411, #3455 ),
 ( #14334, #7432, #3370 ),
 ( #16910, #4866, #14251 ),
 ( #14177, #4785, #711 ),
 ( #3537, #12833, #6104 ),
 ( #9017, #2115, #10175 ),
 ( #7513, #10083, #11502 ),
 ( #14429, #12923, #16823 ),
 ( #801, #7603, #6192 ),
 ( #11592, #2038, #7687 ),
 ( #11667, #17000, #2204 ),
 ( #10256, #15655, #8925 ),
 ( #6277, #17075, #10339 ),
 ( #15747, #3625, #2295 ),
 ( #8764, #13095, #960 ) ),
 .UNSPECIFIED., .F., .F., .F. ) 
 B_SPLINE_SURFACE_WITH_KNOTS ( ( 4, 2, 2, 2, 2, 2, 2, 2, 2, 2, 2, 2, 2, 4 ),
 ( 3, 3 ),
 ( 0.01342997177288654184, 0.01733910390705691029, 0.01929366997414209278, 0.02124823604122727527, 0.02515736817539764372, 0.02711193424248282968, 0.02906650030956801217, 0.03297563244373838409, 0.03493019851082356658, 0.03688476457790874907, 0.03883933064499393156, 0.03981661367853651934, 0.04079389671207911405, 0.04470302884624948597 ),
 ( 0.000000000000000000, 1.000000000000000000 ),
 .UNSPECIFIED. ) 
 GEOMETRIC_REPRESENTATION_ITEM ( )  RATIONAL_B_SPLINE_SURFACE ( (
 ( 1.000000000000000000, 0.7117435966472906994, 1.000000000000000000),
 ( 1.000000000000000000, 0.7117434842622788471, 1.000000000000000000),
 ( 1.000000000000000000, 0.7117144184576317256, 1.000000000000000000),
 ( 1.000000000000000000, 0.7116285301813536357, 1.000000000000000000),
 ( 1.000000000000000000, 0.7115928256594988843, 1.000000000000000000),
 ( 1.000000000000000000, 0.7115068832447583036, 1.000000000000000000),
 ( 1.000000000000000000, 0.7114564033771691998, 1.000000000000000000),
 ( 1.000000000000000000, 0.7112861117250206533, 1.000000000000000000),
 ( 1.000000000000000000, 0.7111469280185451769, 1.000000000000000000),
 ( 1.000000000000000000, 0.7108993804763810154, 1.000000000000000000),
 ( 1.000000000000000000, 0.7108100171490498997, 1.000000000000000000),
 ( 1.000000000000000000, 0.7106191415567917335, 1.000000000000000000),
 ( 1.000000000000000000, 0.7105185320923617098, 1.000000000000000000),
 ( 1.000000000000000000, 0.7102014790723296667, 1.000000000000000000),
 ( 1.000000000000000000, 0.7099699576741209661, 1.000000000000000000),
 ( 1.000000000000000000, 0.7095909300314675594, 1.000000000000000000),
 ( 1.000000000000000000, 0.7094593121158619953, 1.000000000000000000),
 ( 1.000000000000000000, 0.7091910831478104305, 1.000000000000000000),
 ( 1.000000000000000000, 0.7090537746377190143, 1.000000000000000000),
 ( 1.000000000000000000, 0.7087727591781516345, 1.000000000000000000),
 ( 1.000000000000000000, 0.7086290523620303317, 1.000000000000000000),
 ( 1.000000000000000000, 0.7084085592173990920, 1.000000000000000000),
 ( 1.000000000000000000, 0.7083342380282030559, 1.000000000000000000),
 ( 1.000000000000000000, 0.7081839094108949295, 1.000000000000000000),
 ( 1.000000000000000000, 0.7081077478408516201, 1.000000000000000000),
 ( 1.000000000000000000, 0.7077267031859736379, 1.000000000000000000),
 ( 1.000000000000000000, 0.7074184602292508117, 1.000000000000000000),
 ( 1.000000000000000000, 0.7071067811865475727, 1.000000000000000000) ) ) 
 REPRESENTATION_ITEM ( '' )  SURFACE ( )  );
#2614=EDGE_LOOP ( 'NONE', ( #6751, #6307, #16661, #2906 ) ) ;
#2618=DIRECTION ( 'NONE',  ( -1.000000000000000000, 0.000000000000000000, 0.000000000000000000 ) ) ;
#2619=CARTESIAN_POINT ( 'NONE',  ( 36.00000000000002132, 146.6227766016838245, -24.49489742783179125 ) ) ;
#2624=CARTESIAN_POINT ( 'NONE',  ( -85.34459197722598844, 199.3716779298525807, -21.33657927093678808 ) ) ;
#2625=CARTESIAN_POINT ( 'NONE',  ( 18.16062352778163813, 29.95676120085481386, -14.47054584901207619 ) ) ;
#2627=DIRECTION ( 'NONE',  ( 1.000000000000000000, -0.000000000000000000, -0.000000000000000000 ) ) ;
#2630=CARTESIAN_POINT ( 'NONE',  ( -87.21337428997478014, 144.5042670319084550, -18.82352572523458889 ) ) ;
#2631=EDGE_CURVE ( 'NONE', #8768, #6671, #15852, .T. ) ;
#2633=FACE_OUTER_BOUND ( 'NONE', #2614, .T. ) ;
#2634=LINE ( 'NONE', #4132, #9607 ) ;
#2636=DIRECTION ( 'NONE',  ( 0.000000000000000000, 0.000000000000000000, 1.000000000000000000 ) ) ;
#2638=CARTESIAN_POINT ( 'NONE',  ( 39.99999999999998579, 4.000000000000000000, -33.00000000000000711 ) ) ;
#2639=DIRECTION ( 'NONE',  ( 1.000000000000000000, 0.000000000000000000, 0.000000000000000000 ) ) ;
#2640=CARTESIAN_POINT ( 'NONE',  ( -81.04928679900669408, 140.7094120356993585, -16.41247553121493752 ) ) ;
#2641=DIRECTION ( 'NONE',  ( 0.000000000000000000, 0.000000000000000000, 1.000000000000000000 ) ) ;
#2648=CARTESIAN_POINT ( 'NONE',  ( 22.72753210816244618, 139.3086630800672765, -13.45249220522710232 ) ) ;
#2649=ORIENTED_EDGE ( 'NONE', *, *, #16804, .F. ) ;
#2650=CARTESIAN_POINT ( 'NONE',  ( -79.79013591204304134, 152.6234490708242504, -29.39431159376453806 ) ) ;
#2651=CARTESIAN_POINT ( 'NONE',  ( 26.57417986947462651, 139.5089559931849692, -7.600184560211070917 ) ) ;
#2654=DIRECTION ( 'NONE',  ( 1.000000000000000000, 0.000000000000000000, -0.000000000000000000 ) ) ;
#2656=ADVANCED_FACE ( 'NONE', ( #13544 ), #9718, .T. ) ;
#2657=DIRECTION ( 'NONE',  ( -0.000000000000000000, -0.000000000000000000, 1.000000000000000000 ) ) ;
#2658=CARTESIAN_POINT ( 'NONE',  ( 21.38845554303141938, 18.00000000000000000, -23.94082098111162082 ) ) ;
#2659=CARTESIAN_POINT ( 'NONE',  ( 19.81659905433974700, 29.90262535319825332, -11.35915249282563444 ) ) ;
#2661=LINE ( 'NONE', #7970, #10421 ) ;
#2667=ORIENTED_EDGE ( 'NONE', *, *, #8607, .F. ) ;
#2673=ORIENTED_EDGE ( 'NONE', *, *, #15766, .T. ) ;
#2674=DIRECTION ( 'NONE',  ( 1.000000000000000000, 0.000000000000000000, 0.000000000000000000 ) ) ;
#2676=ORIENTED_EDGE ( 'NONE', *, *, #10954, .T. ) ;
#2677=ADVANCED_FACE ( 'NONE', ( #12557 ), #1420, .F. ) ;
#2678=EDGE_CURVE ( 'NONE', #14137, #7753, #1985, .T. ) ;
#2680=EDGE_CURVE ( 'NONE', #14929, #9167, #6822, .T. ) ;
#2683=CARTESIAN_POINT ( 'NONE',  ( 37.50000000000001421, 196.4352734575233228, -21.75827460206395614 ) ) ;
#2684=CARTESIAN_POINT ( 'NONE',  ( 17.58250999373992585, 125.2198453306090329, 1.325401613797208934E-14 ) ) ;
#2686=ORIENTED_EDGE ( 'NONE', *, *, #9891, .F. ) ;
#2688=ORIENTED_EDGE ( 'NONE', *, *, #5475, .F. ) ;
#2689=CARTESIAN_POINT ( 'NONE',  ( 32.50000000000000000, 196.6227766016838245, -16.00000000000000000 ) ) ;
#2695=ORIENTED_EDGE ( 'NONE', *, *, #4283, .F. ) ;
#2696=EDGE_CURVE ( 'NONE', #2293, #8849, #17025, .T. ) ;
#2700=CARTESIAN_POINT ( 'NONE',  ( 17.00000000000000000, 171.6227766016838245, 0.000000000000000000 ) ) ;
#2703=CARTESIAN_POINT ( 'NONE',  ( -100.0000000000000000, 136.6227766016838245, 0.000000000000000000 ) ) ;
#2709=CARTESIAN_POINT ( 'NONE',  ( -81.97708560105468223, 202.2921397697441535, -16.86471387523356213 ) ) ;
#2710=CARTESIAN_POINT ( 'NONE',  ( 36.00000000000002132, 146.6227766016838245, -35.00000000000000000 ) ) ;
#2715=DIRECTION ( 'NONE',  ( 1.000000000000000000, 0.000000000000000000, 0.000000000000000000 ) ) ;
#2716=EDGE_CURVE ( 'NONE', #2293, #11521, #11401, .T. ) ;
#2720=ORIENTED_EDGE ( 'NONE', *, *, #2073, .T. ) ;
#2723=CARTESIAN_POINT ( 'NONE',  ( 27.99999999999998224, 9.999999999999998224, -28.00000000000001066 ) ) ;
#2724=CARTESIAN_POINT ( 'NONE',  ( 22.99999999999997868, 9.999999999999998224, -12.99999999999999822 ) ) ;
#2729=ORIENTED_EDGE ( 'NONE', *, *, #2545, .T. ) ;
#2732=AXIS2_PLACEMENT_3D ( 'NONE', #4392, #15182, #13954 ) ;
#2736=VERTEX_POINT ( 'NONE', #10244 ) ;
#2739=LINE ( 'NONE', #6820, #16011 ) ;
#2741=ORIENTED_EDGE ( 'NONE', *, *, #5382, .T. ) ;
#2743=AXIS2_PLACEMENT_3D ( 'NONE', #10908, #116, #4366 ) ;
#2745=CIRCLE ( 'NONE', #12641, 2.500000000000000000 ) ;
#2746=CARTESIAN_POINT ( 'NONE',  ( -38.00000000000000000, 20.00000000000000000, 0.000000000000000000 ) ) ;
#2748=CARTESIAN_POINT ( 'NONE',  ( 31.20890926080315353, 18.00000000000000000, -16.64259892333393154 ) ) ;
#2749=EDGE_CURVE ( 'NONE', #8947, #11114, #1845, .T. ) ;
#2750=CARTESIAN_POINT ( 'NONE',  ( 22.66736643345232949, 29.84725565559530480, -7.069278529401977984 ) ) ;
#2753=LINE ( 'NONE', #7973, #6503 ) ;
#2754=CARTESIAN_POINT ( 'NONE',  ( 24.03488658890935525, 145.8838445361197387, -23.72313757307398419 ) ) ;
#2755=ORIENTED_EDGE ( 'NONE', *, *, #14042, .T. ) ;
#2756=CARTESIAN_POINT ( 'NONE',  ( 196.0000000000000000, 167.6227766016838814, -16.92820660268601429 ) ) ;
#2757=VECTOR ( 'NONE', #5489, 1000.000000000000000 ) ;
#2761=DIRECTION ( 'NONE',  ( -0.000000000000000000, -0.000000000000000000, 1.000000000000000000 ) ) ;
#2767=FACE_OUTER_BOUND ( 'NONE', #10728, .T. ) ;
#2770=VECTOR ( 'NONE', #3759, 1000.000000000000000 ) ;
#2773=FACE_OUTER_BOUND ( 'NONE', #6459, .T. ) ;
#2774=ORIENTED_EDGE ( 'NONE', *, *, #6823, .T. ) ;
#2777=DIRECTION ( 'NONE',  ( 0.000000000000000000, 0.000000000000000000, 1.000000000000000000 ) ) ;
#2778=DIRECTION ( 'NONE',  ( 1.000000000000000000, 0.000000000000000000, 0.000000000000000000 ) ) ;
#2779=EDGE_CURVE ( 'NONE', #14060, #5354, #14319, .T. ) ;
#2782=AXIS2_PLACEMENT_3D ( 'NONE', #8873, #5076, #17031 ) ;
#2789=VERTEX_POINT ( 'NONE', #2100 ) ;
#2791=CARTESIAN_POINT ( 'NONE',  ( 49.99999999999998579, 191.6227766016837677, -8.071800142134975431 ) ) ;
#2797=VERTEX_POINT ( 'NONE', #7500 ) ;
#2798=CARTESIAN_POINT ( 'NONE',  ( -77.99750410702147008, 202.2831825963720007, -16.88100368216885983 ) ) ;
#2799=DIRECTION ( 'NONE',  ( 0.000000000000000000, 0.000000000000000000, -1.000000000000000000 ) ) ;
#2800=CARTESIAN_POINT ( 'NONE',  ( 31.20890926080315353, 19.99999999999999289, -16.64259892333393154 ) ) ;
#2803=ORIENTED_EDGE ( 'NONE', *, *, #3444, .F. ) ;
#2808=AXIS2_PLACEMENT_3D ( 'NONE', #1284, #6690, #15893 ) ;
#2811=DIRECTION ( 'NONE',  ( 0.000000000000000000, 0.000000000000000000, 1.000000000000000000 ) ) ;
#2812=DIRECTION ( 'NONE',  ( -1.000000000000000000, -0.000000000000000000, 0.000000000000000000 ) ) ;
#2817=CARTESIAN_POINT ( 'NONE',  ( -38.00000000000000000, 18.00000000000000355, 0.000000000000000000 ) ) ;
#2820=EDGE_CURVE ( 'NONE', #14506, #4234, #15645, .T. ) ;
#2822=CYLINDRICAL_SURFACE ( 'NONE', #15992, 747.9999999999998863 ) ;
#2826=CARTESIAN_POINT ( 'NONE',  ( -90.80384757729339640, 204.6227766016838245, 0.000000000000000000 ) ) ;
#2834=DIRECTION ( 'NONE',  ( 0.000000000000000000, 0.000000000000000000, -1.000000000000000000 ) ) ;
#2835=PLANE ( 'NONE',  #7064 ) ;
#2837=VERTEX_POINT ( 'NONE', #1131 ) ;
#2838=DIRECTION ( 'NONE',  ( -1.000000000000000000, -0.000000000000000000, 0.000000000000000000 ) ) ;
#2839=CIRCLE ( 'NONE', #10420, 2.500000000000002220 ) ;
#2844=DIRECTION ( 'NONE',  ( -0.000000000000000000, -0.000000000000000000, 1.000000000000000000 ) ) ;
#2849=DIRECTION ( 'NONE',  ( -1.000000000000000000, 0.000000000000000000, 0.000000000000000000 ) ) ;
#2851=CARTESIAN_POINT ( 'NONE',  ( 32.00760546193473033, 153.8546784850603615, -27.80828541846619473 ) ) ;
#2854=LINE ( 'NONE', #13739, #16594 ) ;
#2856=DIRECTION ( 'NONE',  ( 0.000000000000000000, 0.000000000000000000, 1.000000000000000000 ) ) ;
#2857=VERTEX_POINT ( 'NONE', #2638 ) ;
#2858=DIRECTION ( 'NONE',  ( -1.000000000000000000, 0.000000000000000000, 0.000000000000000000 ) ) ;
#2861=ORIENTED_EDGE ( 'NONE', *, *, #1727, .F. ) ;
#2863=CARTESIAN_POINT ( 'NONE',  ( 49.99999999999998579, 151.6227766016839098, -8.071800142134973655 ) ) ;
#2864=AXIS2_PLACEMENT_3D ( 'NONE', #14635, #2856, #10899 ) ;
#2866=ORIENTED_EDGE ( 'NONE', *, *, #14733, .T. ) ;
#2867=ORIENTED_EDGE ( 'NONE', *, *, #2545, .F. ) ;
#2872=DIRECTION ( 'NONE',  ( -0.000000000000000000, -0.000000000000000000, 1.000000000000000000 ) ) ;
#2873=CARTESIAN_POINT ( 'NONE',  ( -80.00000000000001421, 196.6227766016838245, -35.00200000000000244 ) ) ;
#2874=CARTESIAN_POINT ( 'NONE',  ( 48.00000000000000711, 175.6227766016838530, -21.92820660268601074 ) ) ;
#2877=EDGE_CURVE ( 'NONE', #15883, #4234, #17145, .T. ) ;
#2878=DIRECTION ( 'NONE',  ( 0.000000000000000000, -0.8660254037844413721, -0.4999999999999953371 ) ) ;
#2879=EDGE_CURVE ( 'NONE', #17378, #1367, #16100, .T. ) ;
#2880=ORIENTED_EDGE ( 'NONE', *, *, #16290, .F. ) ;
#2882=CARTESIAN_POINT ( 'NONE',  ( 30.00000000000000355, 196.6227766016838245, -13.00000000000000000 ) ) ;
#2883=CARTESIAN_POINT ( 'NONE',  ( -33.99999999999997868, 10.00000000000000000, -16.00000000000000000 ) ) ;
#2884=CARTESIAN_POINT ( 'NONE',  ( -43.00000000000001421, 125.3137084989847665, -13.00000000000000178 ) ) ;
#2885=CARTESIAN_POINT ( 'NONE',  ( -725.0000000000000000, 134.2062027339443944, -13.00000000000000000 ) ) ;
#2888=LINE ( 'NONE', #8279, #12730 ) ;
#2889=EDGE_LOOP ( 'NONE', ( #13229, #3520, #8309, #11572 ) ) ;
#2893=CARTESIAN_POINT ( 'NONE',  ( -100.0000000000000000, 201.9542783778900059, -13.00000000000000000 ) ) ;
#2898=ADVANCED_FACE ( 'NONE', ( #9435 ), #3273, .F. ) ;
#2899=ORIENTED_EDGE ( 'NONE', *, *, #13334, .T. ) ;
#2901=CARTESIAN_POINT ( 'NONE',  ( -45.00000000000000000, 171.6227766016838245, 0.000000000000000000 ) ) ;
#2902=DIRECTION ( 'NONE',  ( -1.000000000000000000, 0.000000000000000000, 0.000000000000000000 ) ) ;
#2903=DIRECTION ( 'NONE',  ( -1.000000000000000000, 0.000000000000000000, 0.000000000000000000 ) ) ;
#2905=CARTESIAN_POINT ( 'NONE',  ( 21.84350049701297536, 139.6359888969276426, -14.21326463380156646 ) ) ;
#2906=ORIENTED_EDGE ( 'NONE', *, *, #10774, .F. ) ;
#2908=CARTESIAN_POINT ( 'NONE',  ( 196.0000000000000000, 183.6227766016837961, -8.071800142134975431 ) ) ;
#2909=ORIENTED_EDGE ( 'NONE', *, *, #10335, .T. ) ;
#2911=CARTESIAN_POINT ( 'NONE',  ( -75.97730433202670497, 192.1516832787069688, -28.34894355864045679 ) ) ;
#2912=EDGE_CURVE ( 'NONE', #16523, #16282, #290, .T. ) ;
#2913=DIRECTION ( 'NONE',  ( 0.000000000000000000, 0.000000000000000000, 1.000000000000000000 ) ) ;
#2915=CARTESIAN_POINT ( 'NONE',  ( -77.50000000000002842, 146.6227766016838245, 1.387778780781445676E-14 ) ) ;
#2916=CARTESIAN_POINT ( 'NONE',  ( -18.25212770525996930, 32.30769230769230660, -15.00000000000000000 ) ) ;
#2917=DIRECTION ( 'NONE',  ( -1.156482317317868274E-16, 1.000000000000000000, 0.000000000000000000 ) ) ;
#2918=CARTESIAN_POINT ( 'NONE',  ( 12.11856678106299512, 143.7750213247282431, -17.70723251555758537 ) ) ;
#2919=FACE_BOUND ( 'NONE', #8659, .T. ) ;
#2921=CARTESIAN_POINT ( 'NONE',  ( -9.825395436088792067, 30.54854208321445341, -14.75250191942001088 ) ) ;
#2922=VERTEX_POINT ( 'NONE', #5385 ) ;
#2927=DIRECTION ( 'NONE',  ( -1.000000000000000000, -0.000000000000000000, -0.000000000000000000 ) ) ;
#2929=CARTESIAN_POINT ( 'NONE',  ( -27.99999999999998224, 10.00000000000000000, -16.00000000000000000 ) ) ;
#2931=ORIENTED_EDGE ( 'NONE', *, *, #15097, .T. ) ;
#2933=FACE_OUTER_BOUND ( 'NONE', #7986, .T. ) ;
#2935=VERTEX_POINT ( 'NONE', #10853 ) ;
#2944=LINE ( 'NONE', #6856, #4981 ) ;
#2948=CYLINDRICAL_SURFACE ( 'NONE', #14577, 20.00000000000000355 ) ;
#2949=CIRCLE ( 'NONE', #4652, 20.00000000000000355 ) ;
#2956=CARTESIAN_POINT ( 'NONE',  ( 21.29916379186985154, 29.87370047437059384, -9.875089623381150261 ) ) ;
#2959=EDGE_CURVE ( 'NONE', #4527, #13322, #15568, .T. ) ;
#2963=AXIS2_PLACEMENT_3D ( 'NONE', #975, #7444, #6375 ) ;
#2967=VERTEX_POINT ( 'NONE', #12198 ) ;
#2971=ORIENTED_EDGE ( 'NONE', *, *, #281, .T. ) ;
#2976=AXIS2_PLACEMENT_3D ( 'NONE', #6722, #6814, #12207 ) ;
#2980=CARTESIAN_POINT ( 'NONE',  ( 37.20996884815642147, 144.4916047800714978, -18.80562413441371206 ) ) ;
#2982=CARTESIAN_POINT ( 'NONE',  ( -23.00000000000002842, 120.0000000000000284, -4.999999999999999112 ) ) ;
#2985=FACE_OUTER_BOUND ( 'NONE', #3988, .T. ) ;
#2988=CARTESIAN_POINT ( 'NONE',  ( 13.66217116581496249, 130.1207327347060527, -12.31521373833130717 ) ) ;
#2997=DIRECTION ( 'NONE',  ( -1.000000000000000000, -6.938893903907228378E-16, -0.000000000000000000 ) ) ;
#2998=AXIS2_PLACEMENT_3D ( 'NONE', #8861, #13038, #11524 ) ;
#3000=CIRCLE ( 'NONE', #1012, 7.499999999999996447 ) ;
#3001=DIRECTION ( 'NONE',  ( 0.000000000000000000, -1.000000000000000000, 0.000000000000000000 ) ) ;
#3006=B_SPLINE_CURVE_WITH_KNOTS ( 'NONE', 3,
 ( #12809, #16719, #12463, #13967, #1829, #1920, #2980, #9965, #679, #8377 ),
 .UNSPECIFIED., .F., .F.,
 ( 4, 2, 2, 2, 4 ),
 ( 2.030441771438897272E-17, 0.002588446031580681969, 0.005176892063161337917, 0.007765338094741995600, 0.01035378412632265502 ),
 .UNSPECIFIED. ) ;
#3007=ORIENTED_EDGE ( 'NONE', *, *, #10791, .T. ) ;
#3011=CARTESIAN_POINT ( 'NONE',  ( -86.00000000000001421, 196.6227766016838245, -35.00000000000000000 ) ) ;
#3012=AXIS2_PLACEMENT_3D ( 'NONE', #7082, #10872, #13816 ) ;
#3017=VERTEX_POINT ( 'NONE', #8374 ) ;
#3018=CARTESIAN_POINT ( 'NONE',  ( 22.50000000000001421, 146.6227766016838245, -21.54065922853802562 ) ) ;
#3020=DIRECTION ( 'NONE',  ( -1.000000000000000000, -0.000000000000000000, 0.000000000000000000 ) ) ;
#3023=CIRCLE ( 'NONE', #12926, 6.000000000000005329 ) ;
#3026=DIRECTION ( 'NONE',  ( 1.000000000000000000, 0.000000000000000000, -0.000000000000000000 ) ) ;
#3029=VERTEX_POINT ( 'NONE', #328 ) ;
#3030=EDGE_CURVE ( 'NONE', #10869, #102, #13593, .T. ) ;
#3031=DIRECTION ( 'NONE',  ( -0.000000000000000000, -0.000000000000000000, 1.000000000000000000 ) ) ;
#3032=DIRECTION ( 'NONE',  ( 0.000000000000000000, 1.000000000000000000, 0.000000000000000000 ) ) ;
#3036=CARTESIAN_POINT ( 'NONE',  ( 30.49999999999998224, 9.999999999999998224, -16.00000000000000000 ) ) ;
#3038=CARTESIAN_POINT ( 'NONE',  ( 196.0000000000000000, 167.6227766016838814, -19.42820660268601074 ) ) ;
#3039=CARTESIAN_POINT ( 'NONE',  ( 27.44407568426053246, 138.8271129316868837, -3.666666666666671404 ) ) ;
#3043=DIRECTION ( 'NONE',  ( -1.000000000000000000, 0.000000000000000000, 0.000000000000000000 ) ) ;
#3044=CARTESIAN_POINT ( 'NONE',  ( 22.66773460012013430, 29.84724857135450193, -7.067878044979525320 ) ) ;
#3048=ORIENTED_EDGE ( 'NONE', *, *, #8512, .F. ) ;
#3053=ADVANCED_FACE ( 'NONE', ( #5728 ), #11117, .T. ) ;
#3056=CARTESIAN_POINT ( 'NONE',  ( -70.00000000000000000, 206.6227766016838245, 2.143131898507868248E-15 ) ) ;
#3058=ORIENTED_EDGE ( 'NONE', *, *, #12376, .T. ) ;
#3059=EDGE_CURVE ( 'NONE', #15769, #11112, #12464, .T. ) ;
#3060=CARTESIAN_POINT ( 'NONE',  ( -27.98221281347037959, 30.00000000000000000, -15.00000000000000000 ) ) ;
#3063=FILL_AREA_STYLE ('',( #3238 ) ) ;
#3064=EDGE_CURVE ( 'NONE', #14627, #9221, #18, .T. ) ;
#3065=VERTEX_POINT ( 'NONE', #12724 ) ;
#3066=( NAMED_UNIT ( * ) SI_UNIT ( $, .STERADIAN. ) SOLID_ANGLE_UNIT ( ) );
#3068=CARTESIAN_POINT ( 'NONE',  ( 0.000000000000000000, 0.000000000000000000, 0.000000000000000000 ) ) ;
#3069=CIRCLE ( 'NONE', #15222, 2.500000000000000000 ) ;
#3072=B_SPLINE_CURVE_WITH_KNOTS ( 'NONE', 3,
 ( #13837, #1701, #7098, #363, #16572, #8509, #12934, #14343, #9996, #8688 ),
 .UNSPECIFIED., .F., .F.,
 ( 4, 2, 2, 2, 4 ),
 ( 0.03775390620236029199, 0.04033669301524710205, 0.04291947982813391210, 0.04550226664102072216, 0.04808505345390753222 ),
 .UNSPECIFIED. ) ;
#3074=CARTESIAN_POINT ( 'NONE',  ( 32.90650748920769075, 18.00000000000000000, -13.87185692903161360 ) ) ;
#3081=AXIS2_PLACEMENT_3D ( 'NONE', #13874, #14044, #3327 ) ;
#3085=FACE_OUTER_BOUND ( 'NONE', #11269, .T. ) ;
#3088=DIRECTION ( 'NONE',  ( 1.000000000000000000, 0.000000000000000000, 0.000000000000000000 ) ) ;
#3089=DIRECTION ( 'NONE',  ( 0.000000000000000000, 0.000000000000000000, 1.000000000000000000 ) ) ;
#3091=VECTOR ( 'NONE', #3472, 1000.000000000000000 ) ;
#3093=AXIS2_PLACEMENT_3D ( 'NONE', #10503, #11735, #5525 ) ;
#3094=DIRECTION ( 'NONE',  ( 0.000000000000000000, 0.000000000000000000, -1.000000000000000000 ) ) ;
#3096=LINE ( 'NONE', #16557, #7039 ) ;
#3098=EDGE_CURVE ( 'NONE', #4046, #9326, #5995, .T. ) ;
#3099=LINE ( 'NONE', #15392, #1981 ) ;
#3101=FACE_BOUND ( 'NONE', #11966, .T. ) ;
#3102=ORIENTED_EDGE ( 'NONE', *, *, #2022, .F. ) ;
#3104=CARTESIAN_POINT ( 'NONE',  ( 34.80444759362561058, 19.99999999999999645, -7.621511755370173447 ) ) ;
#3105=CYLINDRICAL_SURFACE ( 'NONE', #5843, 12.00000000000000000 ) ;
#3108=VECTOR ( 'NONE', #2997, 1000.000000000000000 ) ;
#3115=VECTOR ( 'NONE', #1352, 1000.000000000000000 ) ;
#3118=EDGE_CURVE ( 'NONE', #14929, #4566, #3339, .T. ) ;
#3119=CARTESIAN_POINT ( 'NONE',  ( 24.72505082391213804, 141.2912748254776147, -13.00000000000000000 ) ) ;
#3121=EDGE_CURVE ( 'NONE', #453, #7418, #7700, .T. ) ;
#3122=DIRECTION ( 'NONE',  ( -1.156482317317868274E-16, 1.000000000000000000, 0.000000000000000000 ) ) ;
#3127=CARTESIAN_POINT ( 'NONE',  ( -7.379000772445021283, 30.00000000000000000, -13.00000000000000000 ) ) ;
#3128=EDGE_LOOP ( 'NONE', ( #16767, #4880, #6389 ) ) ;
#3132=LINE ( 'NONE', #16591, #4516 ) ;
#3135=ORIENTED_EDGE ( 'NONE', *, *, #11106, .F. ) ;
#3139=CARTESIAN_POINT ( 'NONE',  ( -3.000000000000000888, 154.3022685259950038, -9.999999999999900524 ) ) ;
#3145=ORIENTED_EDGE ( 'NONE', *, *, #4525, .F. ) ;
#3146=LINE ( 'NONE', #8623, #12378 ) ;
#3147=VECTOR ( 'NONE', #14915, 1000.000000000000000 ) ;
#3148=CARTESIAN_POINT ( 'NONE',  ( -3.000000000000000888, 171.6227766016838245, -20.00000000000000355 ) ) ;
#3149=LINE ( 'NONE', #228, #15108 ) ;
#3150=CARTESIAN_POINT ( 'NONE',  ( 32.50000000000000000, 196.6227766016838245, 1.387778780781445676E-14 ) ) ;
#3151=CARTESIAN_POINT ( 'NONE',  ( 15.00000000000000000, 154.3022685259950038, -9.999999999999900524 ) ) ;
#3152=ORIENTED_EDGE ( 'NONE', *, *, #11462, .F. ) ;
#3153=ORIENTED_EDGE ( 'NONE', *, *, #13035, .F. ) ;
#3154=ORIENTED_EDGE ( 'NONE', *, *, #11923, .F. ) ;
#3157=( LENGTH_UNIT ( ) NAMED_UNIT ( * ) SI_UNIT ( .MILLI., .METRE. ) );
#3161=CARTESIAN_POINT ( 'NONE',  ( 30.00000000000000355, 196.6227766016838245, -35.00200000000000244 ) ) ;
#3165=DIRECTION ( 'NONE',  ( 0.000000000000000000, -0.8660254037844413721, -0.4999999999999953371 ) ) ;
#3166=ORIENTED_EDGE ( 'NONE', *, *, #8022, .T. ) ;
#3168=ADVANCED_FACE ( 'NONE', ( #6070 ), #11465, .F. ) ;
#3171=EDGE_CURVE ( 'NONE', #2857, #14947, #15625, .T. ) ;
#3174=( BOUNDED_SURFACE ( )  B_SPLINE_SURFACE ( 3, 2, ( 
 ( #7922, #15708, #930 ),
 ( #13328, #2428, #1192 ),
 ( #6597, #11988, #10663 ),
 ( #8980, #16074, #7827 ) ),
 .UNSPECIFIED., .F., .F., .F. ) 
 B_SPLINE_SURFACE_WITH_KNOTS ( ( 4, 4 ),
 ( 3, 3 ),
 ( 0.1516087691302821228, 0.1566150273425061523 ),
 ( 0.000000000000000000, 1.000000000000000000 ),
 .UNSPECIFIED. ) 
 GEOMETRIC_REPRESENTATION_ITEM ( )  RATIONAL_B_SPLINE_SURFACE ( (
 ( 1.000000000000000000, 0.6556320892438535219, 1.000000000000000000),
 ( 1.000000000000000000, 0.6556321914870770762, 1.000000000000000000),
 ( 1.000000000000000000, 0.6556957163104851771, 1.000000000000000000),
 ( 1.000000000000000000, 0.6558243695371216431, 1.000000000000000000) ) ) 
 REPRESENTATION_ITEM ( '' )  SURFACE ( )  );
#3175=CARTESIAN_POINT ( 'NONE',  ( -27.99999999999998224, 10.00000000000000000, -16.00000000000000000 ) ) ;
#3180=DIRECTION ( 'NONE',  ( -0.000000000000000000, -0.000000000000000000, 1.000000000000000000 ) ) ;
#3186=CARTESIAN_POINT ( 'NONE',  ( 30.00000000000000355, 196.6227766016838245, 0.000000000000000000 ) ) ;
#3188=VERTEX_POINT ( 'NONE', #11557 ) ;
#3190=CARTESIAN_POINT ( 'NONE',  ( 23.15530394309853435, 20.00000000000112976, -10.88800651875285297 ) ) ;
#3191=DIRECTION ( 'NONE',  ( -1.000000000000000000, 8.673617379884038430E-16, 0.000000000000000000 ) ) ;
#3193=CYLINDRICAL_SURFACE ( 'NONE', #11218, 7.500000000000003553 ) ;
#3194=DIRECTION ( 'NONE',  ( -0.000000000000000000, -0.000000000000000000, 1.000000000000000000 ) ) ;
#3195=EDGE_LOOP ( 'NONE', ( #5727, #113, #12363, #1294 ) ) ;
#3196=EDGE_CURVE ( 'NONE', #9392, #11298, #2574, .T. ) ;
#3198=CARTESIAN_POINT ( 'NONE',  ( 24.91549491446250286, 152.1614365523548713, -26.65369102675423818 ) ) ;
#3199=DIRECTION ( 'NONE',  ( -0.000000000000000000, -0.000000000000000000, -1.000000000000000000 ) ) ;
#3202=DIRECTION ( 'NONE',  ( -1.000000000000000000, -0.000000000000000000, 0.000000000000000000 ) ) ;
#3203=CARTESIAN_POINT ( 'NONE',  ( -27.99999999999998224, 10.00000000000000000, 1.387778780781445676E-14 ) ) ;
#3204=DIRECTION ( 'NONE',  ( 0.000000000000000000, 0.000000000000000000, 1.000000000000000000 ) ) ;
#3207=EDGE_LOOP ( 'NONE', ( #17376, #7307, #6041, #12589 ) ) ;
#3209=FACE_BOUND ( 'NONE', #5928, .T. ) ;
#3210=VERTEX_POINT ( 'NONE', #16624 ) ;
#3212=ADVANCED_FACE ( 'NONE', ( #4494 ), #9883, .T. ) ;
#3213=ADVANCED_FACE ( 'NONE', ( #9961, #12977 ), #10389, .F. ) ;
#3220=DIRECTION ( 'NONE',  ( -1.000000000000000000, 0.000000000000000000, 0.000000000000000000 ) ) ;
#3221=DIRECTION ( 'NONE',  ( 1.000000000000000000, 0.000000000000000000, 0.000000000000000000 ) ) ;
#3224=CARTESIAN_POINT ( 'NONE',  ( -8.720613081040614389, 18.00000000000000000, -24.99999999951824492 ) ) ;
#3230=DIRECTION ( 'NONE',  ( -1.000000000000000000, -6.938893903907228378E-16, -0.000000000000000000 ) ) ;
#3231=CIRCLE ( 'NONE', #13122, 5.000000000000000888 ) ;
#3232=ORIENTED_EDGE ( 'NONE', *, *, #16711, .F. ) ;
#3235=ORIENTED_EDGE ( 'NONE', *, *, #8316, .F. ) ;
#3237=ORIENTED_EDGE ( 'NONE', *, *, #15267, .F. ) ;
#3238=FILL_AREA_STYLE_COLOUR ( '', #16617 ) ;
#3243=CARTESIAN_POINT ( 'NONE',  ( 39.99999999999998579, 0.000000000000000000, -33.00000000000000711 ) ) ;
#3248=DIRECTION ( 'NONE',  ( 0.000000000000000000, 8.410780489584519664E-16, 1.000000000000000000 ) ) ;
#3250=CARTESIAN_POINT ( 'NONE',  ( -11.67692690462290273, 19.99999999999766587, -12.94410612366815272 ) ) ;
#3252=ADVANCED_FACE ( 'NONE', ( #15974 ), #11809, .F. ) ;
#3257=ORIENTED_EDGE ( 'NONE', *, *, #12388, .F. ) ;
#3259=EDGE_LOOP ( 'NONE', ( #14461, #761, #16369, #4885 ) ) ;
#3261=ADVANCED_FACE ( 'NONE', ( #2528 ), #3174, .T. ) ;
#3262=ORIENTED_EDGE ( 'NONE', *, *, #12035, .F. ) ;
#3263=PLANE ( 'NONE',  #8159 ) ;
#3264=CARTESIAN_POINT ( 'NONE',  ( 17.00000000000000000, 191.6227766016837961, 1.224646799147353454E-15 ) ) ;
#3267=DIRECTION ( 'NONE',  ( 1.000000000000000000, 0.000000000000000000, 0.000000000000000000 ) ) ;
#3268=CARTESIAN_POINT ( 'NONE',  ( 48.00000000000000000, 171.6227766016838245, -12.50000337241049131 ) ) ;
#3270=DIRECTION ( 'NONE',  ( 1.000000000000000000, 0.000000000000000000, 0.000000000000000000 ) ) ;
#3273=( BOUNDED_SURFACE ( )  B_SPLINE_SURFACE ( 3, 2, ( 
 ( #12272, #4138, #13618 ),
 ( #5465, #1486, #8205 ),
 ( #8286, #149, #9525 ),
 ( #5553, #17514, #1661 ) ),
 .UNSPECIFIED., .F., .F., .F. ) 
 B_SPLINE_SURFACE_WITH_KNOTS ( ( 4, 4 ),
 ( 3, 3 ),
 ( 0.1516087691302827056, 0.1566150273425061523 ),
 ( 0.000000000000000000, 1.000000000000000000 ),
 .UNSPECIFIED. ) 
 GEOMETRIC_REPRESENTATION_ITEM ( )  RATIONAL_B_SPLINE_SURFACE ( (
 ( 1.000000000000000000, 0.6556320892438534109, 1.000000000000000000),
 ( 1.000000000000000000, 0.6556321914870764100, 1.000000000000000000),
 ( 1.000000000000000000, 0.6556957163104859543, 1.000000000000000000),
 ( 1.000000000000000000, 0.6558243695371223092, 1.000000000000000000) ) ) 
 REPRESENTATION_ITEM ( '' )  SURFACE ( )  );
#3276=CARTESIAN_POINT ( 'NONE',  ( 30.80964797964808000, 19.99999999999999645, -17.18170494867160514 ) ) ;
#3277=CARTESIAN_POINT ( 'NONE',  ( -74.72505082391214160, 141.2912748254776147, -13.00000000000000000 ) ) ;
#3282=EDGE_LOOP ( 'NONE', ( #10040, #8235, #17339, #15031 ) ) ;
#3283=AXIS2_PLACEMENT_3D ( 'NONE', #14045, #9955, #10291 ) ;
#3292=VECTOR ( 'NONE', #7892, 1000.000000000000000 ) ;
#3293=DIRECTION ( 'NONE',  ( -1.000000000000000000, -0.000000000000000000, 0.000000000000000000 ) ) ;
#3295=ORIENTED_EDGE ( 'NONE', *, *, #6965, .T. ) ;
#3296=CARTESIAN_POINT ( 'NONE',  ( 27.41872110558518116, 136.9783011792879392, -5.130391642808777242 ) ) ;
#3299=VERTEX_POINT ( 'NONE', #2791 ) ;
#3300=CARTESIAN_POINT ( 'NONE',  ( -48.00000000000000000, 154.3022685259950038, -9.999999999999900524 ) ) ;
#3302=CARTESIAN_POINT ( 'NONE',  ( -27.98221281347037959, 18.00000000000000355, -4.999999999999999112 ) ) ;
#3309=EDGE_LOOP ( 'NONE', ( #23, #15054 ) ) ;
#3313=( GEOMETRIC_REPRESENTATION_CONTEXT ( 3 ) GLOBAL_UNCERTAINTY_ASSIGNED_CONTEXT ( ( #6115 ) ) GLOBAL_UNIT_ASSIGNED_CONTEXT ( ( #1398, #13617, #3066 ) ) REPRESENTATION_CONTEXT ( 'NONE', 'WORKASPACE' ) );
#3314=DIRECTION ( 'NONE',  ( 1.000000000000000000, 0.000000000000000000, 0.000000000000000000 ) ) ;
#3321=CARTESIAN_POINT ( 'NONE',  ( -75.20964951580667446, 200.2528945340145015, -20.13811431823771159 ) ) ;
#3324=LINE ( 'NONE', #8721, #16718 ) ;
#3325=EDGE_CURVE ( 'NONE', #11049, #16267, #1711, .T. ) ;
#3327=DIRECTION ( 'NONE',  ( 0.000000000000000000, 1.000000000000000000, 0.000000000000000000 ) ) ;
#3328=FACE_OUTER_BOUND ( 'NONE', #11942, .T. ) ;
#3331=ORIENTED_EDGE ( 'NONE', *, *, #3059, .F. ) ;
#3335=ORIENTED_EDGE ( 'NONE', *, *, #6614, .T. ) ;
#3339=LINE ( 'NONE', #11385, #590 ) ;
#3342=AXIS2_PLACEMENT_3D ( 'NONE', #10122, #16781, #390 ) ;
#3346=FACE_OUTER_BOUND ( 'NONE', #5110, .T. ) ;
#3348=CARTESIAN_POINT ( 'NONE',  ( 22.50000000000000000, 196.6227766016838245, -13.00000000000000000 ) ) ;
#3349=CARTESIAN_POINT ( 'NONE',  ( -7.379000772444995526, 30.00000000000000000, -15.00000000000000355 ) ) ;
#3358=CARTESIAN_POINT ( 'NONE',  ( 32.99999999999998579, 9.999999999999998224, -35.00200000000000244 ) ) ;
#3366=VECTOR ( 'NONE', #15734, 1000.000000000000000 ) ;
#3367=CARTESIAN_POINT ( 'NONE',  ( 30.93864055801722657, 202.5503328113395014, -16.38559373769485461 ) ) ;
#3370=CARTESIAN_POINT ( 'NONE',  ( 27.13959012325755538, 19.99999999999999645, -20.89788123228700556 ) ) ;
#3372=EDGE_LOOP ( 'NONE', ( #6101, #11259 ) ) ;
#3375=DIRECTION ( 'NONE',  ( -1.000000000000000000, 0.000000000000000000, 0.000000000000000000 ) ) ;
#3379=CIRCLE ( 'NONE', #2808, 2.499999999999998668 ) ;
#3380=ADVANCED_FACE ( 'NONE', ( #9502 ), #6782, .F. ) ;
#3381=CYLINDRICAL_SURFACE ( 'NONE', #4941, 6.000000000000001776 ) ;
#3384=CARTESIAN_POINT ( 'NONE',  ( -48.00000000000000000, 171.6227766016838245, 0.000000000000000000 ) ) ;
#3386=CARTESIAN_POINT ( 'NONE',  ( 17.00000000000000000, 154.3022685259950038, -9.999999999999900524 ) ) ;
#3387=CIRCLE ( 'NONE', #9873, 5.000000000000000888 ) ;
#3389=B_SPLINE_CURVE_WITH_KNOTS ( 'NONE', 3,
 ( #16697, #12527, #1733, #15352 ),
 .UNSPECIFIED., .F., .F.,
 ( 4, 4 ),
 ( 0.000000000000000000, 0.003672568685860802366 ),
 .UNSPECIFIED. ) ;
#3390=ORIENTED_EDGE ( 'NONE', *, *, #14733, .F. ) ;
#3394=EDGE_CURVE ( 'NONE', #2136, #9101, #14996, .T. ) ;
#3396=ORIENTED_EDGE ( 'NONE', *, *, #1958, .T. ) ;
#3397=CYLINDRICAL_SURFACE ( 'NONE', #698, 10.00000000000000000 ) ;
#3398=CARTESIAN_POINT ( 'NONE',  ( -74.40238044657790795, 201.6350306476045091, -13.74486639216964079 ) ) ;
#3400=AXIS2_PLACEMENT_3D ( 'NONE', #13612, #12192, #9431 ) ;
#3401=VECTOR ( 'NONE', #13375, 1000.000000000000000 ) ;
#3402=ORIENTED_EDGE ( 'NONE', *, *, #16848, .F. ) ;
#3406=CARTESIAN_POINT ( 'NONE',  ( -11.99846793330598693, 31.02137248309377071, -14.08482506821421509 ) ) ;
#3409=ORIENTED_EDGE ( 'NONE', *, *, #8607, .T. ) ;
#3410=CARTESIAN_POINT ( 'NONE',  ( 30.00000000000000355, 196.6227766016838245, -13.00000000000000000 ) ) ;
#3411=CARTESIAN_POINT ( 'NONE',  ( -27.98221281347037959, 20.00000000000000000, -4.999999999999999112 ) ) ;
#3416=VERTEX_POINT ( 'NONE', #5447 ) ;
#3417=ORIENTED_EDGE ( 'NONE', *, *, #6319, .T. ) ;
#3418=AXIS2_PLACEMENT_3D ( 'NONE', #1376, #218, #13410 ) ;
#3419=VERTEX_POINT ( 'NONE', #1637 ) ;
#3420=DIRECTION ( 'NONE',  ( 1.000000000000000000, 0.000000000000000000, 0.000000000000000000 ) ) ;
#3424=DIRECTION ( 'NONE',  ( 0.000000000000000000, 0.000000000000000000, 1.000000000000000000 ) ) ;
#3425=DIRECTION ( 'NONE',  ( 0.000000000000000000, 0.000000000000000000, -1.000000000000000000 ) ) ;
#3428=DIRECTION ( 'NONE',  ( 0.000000000000000000, 0.000000000000000000, 1.000000000000000000 ) ) ;
#3429=ORIENTED_EDGE ( 'NONE', *, *, #2022, .T. ) ;
#3433=CARTESIAN_POINT ( 'NONE',  ( -14.51002702888200702, 31.55035369552022928, -12.57309263104575869 ) ) ;
#3434=CARTESIAN_POINT ( 'NONE',  ( 27.99999999999998224, 9.999999999999998224, -12.99999999999999822 ) ) ;
#3436=DIRECTION ( 'NONE',  ( -1.000000000000000000, 0.000000000000000000, 0.000000000000000000 ) ) ;
#3440=EDGE_CURVE ( 'NONE', #15255, #3416, #7650, .T. ) ;
#3444=EDGE_CURVE ( 'NONE', #7056, #1055, #3996, .T. ) ;
#3446=CARTESIAN_POINT ( 'NONE',  ( 27.99999999999998224, 9.999999999999998224, 0.000000000000000000 ) ) ;
#3447=CARTESIAN_POINT ( 'NONE',  ( 6.134011831684049731, 134.2062027339443944, -13.00000000000000000 ) ) ;
#3448=ORIENTED_EDGE ( 'NONE', *, *, #4810, .F. ) ;
#3452=CARTESIAN_POINT ( 'NONE',  ( 24.26110014372655144, 198.4077499201236776, -22.53509453904542070 ) ) ;
#3454=VERTEX_POINT ( 'NONE', #10758 ) ;
#3455=CARTESIAN_POINT ( 'NONE',  ( 28.14717441101472772, 19.99999999999999645, -20.07001214883818108 ) ) ;
#3456=DIRECTION ( 'NONE',  ( 1.000000000000000000, 0.000000000000000000, 0.000000000000000000 ) ) ;
#3458=ADVANCED_FACE ( 'NONE', ( #6049 ), #4378, .F. ) ;
#3462=DIRECTION ( 'NONE',  ( 1.000000000000000000, 0.000000000000000000, -0.000000000000000000 ) ) ;
#3463=UNCERTAINTY_MEASURE_WITH_UNIT (LENGTH_MEASURE( 1.000000000000000082E-05 ), #1037, 'distance_accuracy_value', 'NONE');
#3465=DIRECTION ( 'NONE',  ( 1.000000000000000000, 0.000000000000000000, 0.000000000000000000 ) ) ;
#3467=DIRECTION ( 'NONE',  ( 0.000000000000000000, 0.000000000000000000, 1.000000000000000000 ) ) ;
#3468=CYLINDRICAL_SURFACE ( 'NONE', #14273, 5.999999999999998224 ) ;
#3470=CARTESIAN_POINT ( 'NONE',  ( 6.134011831684053284, 142.5209969267753820, -19.44444444444444642 ) ) ;
#3472=DIRECTION ( 'NONE',  ( -0.000000000000000000, -0.000000000000000000, 1.000000000000000000 ) ) ;
#3474=ADVANCED_FACE ( 'NONE', ( #5973 ), #7199, .F. ) ;
#3483=EDGE_CURVE ( 'NONE', #11751, #10197, #9915, .T. ) ;
#3485=CARTESIAN_POINT ( 'NONE',  ( -14.33532356861720380, 31.51408589783374126, -12.70909354450696149 ) ) ;
#3486=LINE ( 'NONE', #10621, #5572 ) ;
#3489=DIRECTION ( 'NONE',  ( 1.000000000000000000, 0.000000000000000000, 0.000000000000000000 ) ) ;
#3491=EDGE_LOOP ( 'NONE', ( #4673, #7484, #5566, #8858, #5429, #6779, #9966 ) ) ;
#3492=CARTESIAN_POINT ( 'NONE',  ( 25.97411924848963594, 192.1541050315147459, -28.34722919022666332 ) ) ;
#3493=FACE_BOUND ( 'NONE', #6892, .T. ) ;
#3495=ORIENTED_EDGE ( 'NONE', *, *, #5514, .F. ) ;
#3496=EDGE_LOOP ( 'NONE', ( #8699, #3235, #10892, #16646, #7400, #1142, #6745, #10375, #12379, #5360 ) ) ;
#3497=ORIENTED_EDGE ( 'NONE', *, *, #3823, .T. ) ;
#3498=CARTESIAN_POINT ( 'NONE',  ( -87.49298393897305459, 147.0010062438373950, -21.97388680505723002 ) ) ;
#3501=DIRECTION ( 'NONE',  ( 8.673617379884037937E-17, 0.000000000000000000, 1.000000000000000000 ) ) ;
#3503=EDGE_CURVE ( 'NONE', #11327, #8547, #13862, .T. ) ;
#3510=CARTESIAN_POINT ( 'NONE',  ( -27.99999999999998224, 10.00000000000000000, -13.00000000000000000 ) ) ;
#3511=CARTESIAN_POINT ( 'NONE',  ( 49.99999999999998579, 151.6227766016839098, -3.071800142134974099 ) ) ;
#3520=ORIENTED_EDGE ( 'NONE', *, *, #10861, .F. ) ;
#3529=CARTESIAN_POINT ( 'NONE',  ( 34.07337191958318101, 201.0442424278814428, -18.96251499051322753 ) ) ;
#3532=EDGE_CURVE ( 'NONE', #4990, #6914, #15292, .T. ) ;
#3533=ADVANCED_FACE ( 'NONE', ( #13102 ), #15757, .F. ) ;
#3534=CIRCLE ( 'NONE', #4099, 2.500000000000002220 ) ;
#3536=ORIENTED_EDGE ( 'NONE', *, *, #3394, .F. ) ;
#3537=CARTESIAN_POINT ( 'NONE',  ( 19.35452547490215736, 29.94096051140668280, -13.97567760708249551 ) ) ;
#3539=EDGE_CURVE ( 'NONE', #6279, #209, #7013, .T. ) ;
#3547=CIRCLE ( 'NONE', #2407, 6.000000000000005329 ) ;
#3548=CARTESIAN_POINT ( 'NONE',  ( -40.00000000000000000, 20.00000000000000000, 0.000000000000000000 ) ) ;
#3549=CARTESIAN_POINT ( 'NONE',  ( -95.00000000000000000, 143.9321776784423150, 5.086680500673126297E-15 ) ) ;
#3552=DIRECTION ( 'NONE',  ( 0.000000000000000000, 1.040834085586084059E-15, -1.000000000000000000 ) ) ;
#3555=ORIENTED_EDGE ( 'NONE', *, *, #6625, .T. ) ;
#3559=CARTESIAN_POINT ( 'NONE',  ( -100.0000000000000000, 171.6227766016838245, 0.000000000000000000 ) ) ;
#3561=EDGE_LOOP ( 'NONE', ( #966, #7996, #9790, #1341 ) ) ;
#3565=DIRECTION ( 'NONE',  ( 0.000000000000000000, 0.000000000000000000, 1.000000000000000000 ) ) ;
#3566=AXIS2_PLACEMENT_3D ( 'NONE', #7634, #16053, #17105 ) ;
#3567=CARTESIAN_POINT ( 'NONE',  ( 23.52759457847468383, 192.8264746069455100, -25.28784208911849518 ) ) ;
#3568=CARTESIAN_POINT ( 'NONE',  ( -16.66926302330761800, 31.99181794709938487, -10.22419352058821396 ) ) ;
#3570=CARTESIAN_POINT ( 'NONE',  ( -9.245637070518823109, 17.99999999999769074, -12.12237611798427572 ) ) ;
#3574=CARTESIAN_POINT ( 'NONE',  ( -26.89314795393037016, 19.99999999999999289, -11.55702759004480207 ) ) ;
#3575=ORIENTED_EDGE ( 'NONE', *, *, #4203, .F. ) ;
#3576=CARTESIAN_POINT ( 'NONE',  ( -22.93725393319379791, 120.0000000000000284, -6.000000000000001776 ) ) ;
#3580=EDGE_LOOP ( 'NONE', ( #10134, #10364, #5963, #94 ) ) ;
#3583=AXIS2_PLACEMENT_3D ( 'NONE', #5482, #6893, #8222 ) ;
#3584=CARTESIAN_POINT ( 'NONE',  ( -77.99239453806532651, 153.8546784850604183, -27.80828541846620539 ) ) ;
#3590=CARTESIAN_POINT ( 'NONE',  ( 27.18872211705360087, 151.9278302392748685, -28.93306197017448866 ) ) ;
#3592=DIRECTION ( 'NONE',  ( 0.000000000000000000, 1.000000000000000000, 0.000000000000000000 ) ) ;
#3593=EDGE_CURVE ( 'NONE', #13962, #6224, #14439, .T. ) ;
#3599=CARTESIAN_POINT ( 'NONE',  ( -27.30244652380281778, 19.99999999999999645, -10.27378278477019080 ) ) ;
#3600=EDGE_LOOP ( 'NONE', ( #5876, #108, #270, #2076, #17078, #12969, #15156, #1622, #10911, #3632, #10206, #13256, #7640, #16853, #15534, #14751, #17072, #1127, #2160, #16582, #4030, #16067, #12740, #15190, #14548, #13523, #13112, #16327, #15322, #9084, #8366, #16483, #1114, #13916, #11093, #10413, #17185, #1539, #16241, #14464, #5400, #11636, #10826, #13850, #3048, #3145, #12610, #913, #1568, #12722, #5229, #6318, #12758, #5147, #17153 ) ) ;
#3607=ORIENTED_EDGE ( 'NONE', *, *, #11009, .T. ) ;
#3608=FACE_OUTER_BOUND ( 'NONE', #4104, .T. ) ;
#3609=DIRECTION ( 'NONE',  ( 0.000000000000000000, -1.000000000000000000, 0.000000000000000000 ) ) ;
#3613=CIRCLE ( 'NONE', #16354, 6.000000000000001776 ) ;
#3614=CARTESIAN_POINT ( 'NONE',  ( 17.00458606767794834, 29.95830270928036398, -12.72829919683579902 ) ) ;
#3616=EDGE_CURVE ( 'NONE', #4595, #9313, #8986, .T. ) ;
#3617=CARTESIAN_POINT ( 'NONE',  ( 9.186438336152177087, 132.7758989760081931, -12.51111164240594675 ) ) ;
#3618=ORIENTED_EDGE ( 'NONE', *, *, #12145, .T. ) ;
#3622=CARTESIAN_POINT ( 'NONE',  ( 24.65540802277405064, 199.3716779298525239, -21.33657927093678452 ) ) ;
#3624=ORIENTED_EDGE ( 'NONE', *, *, #16804, .T. ) ;
#3625=CARTESIAN_POINT ( 'NONE',  ( 15.58467296311467898, 20.00000000001131895, -15.00881168888636807 ) ) ;
#3628=CARTESIAN_POINT ( 'NONE',  ( 10.98422133653362920, 132.2143956889292724, -13.95899527751216240 ) ) ;
#3630=DIRECTION ( 'NONE',  ( 1.000000000000000000, 0.000000000000000000, 0.000000000000000000 ) ) ;
#3631=CARTESIAN_POINT ( 'NONE',  ( 13.54862175821475034, 128.4555333983033734, -9.713103375557215813 ) ) ;
#3632=ORIENTED_EDGE ( 'NONE', *, *, #16739, .F. ) ;
#3635=EDGE_CURVE ( 'NONE', #11591, #13399, #17474, .T. ) ;
#3638=EDGE_CURVE ( 'NONE', #6756, #5589, #5219, .T. ) ;
#3644=CARTESIAN_POINT ( 'NONE',  ( 14.93242934743711992, 30.00000000000000000, -25.00000000000000000 ) ) ;
#3648=DIRECTION ( 'NONE',  ( 1.000000000000000000, 0.000000000000000000, 0.000000000000000000 ) ) ;
#3649=AXIS2_PLACEMENT_3D ( 'NONE', #955, #6350, #11745 ) ;
#3651=AXIS2_PLACEMENT_3D ( 'NONE', #10106, #8603, #12684 ) ;
#3656=CARTESIAN_POINT ( 'NONE',  ( -73.57895800238922845, 200.5259344270104691, -15.94638436093396372 ) ) ;
#3660=CARTESIAN_POINT ( 'NONE',  ( -725.0000000000000000, 19.99999999999995737, -4.999999999999999112 ) ) ;
#3663=VECTOR ( 'NONE', #7410, 1000.000000000000000 ) ;
#3664=DIRECTION ( 'NONE',  ( 1.000000000000000000, 0.000000000000000000, -0.000000000000000000 ) ) ;
#3665=VECTOR ( 'NONE', #5233, 1000.000000000000000 ) ;
#3666=CARTESIAN_POINT ( 'NONE',  ( -12.80328004466210601, 18.00000000000000000, -4.999999999999999112 ) ) ;
#3669=LINE ( 'NONE', #9057, #16907 ) ;
#3671=CARTESIAN_POINT ( 'NONE',  ( 25.29931031416560927, 192.8887977548965011, -27.79913727548661129 ) ) ;
#3672=DIRECTION ( 'NONE',  ( -1.000000000000000000, -0.000000000000000000, -0.000000000000000000 ) ) ;
#3674=ORIENTED_EDGE ( 'NONE', *, *, #15055, .T. ) ;
#3678=EDGE_CURVE ( 'NONE', #6832, #14506, #17348, .T. ) ;
#3679=CARTESIAN_POINT ( 'NONE',  ( -86.80495063319472138, 149.8103701614163015, -24.76910924193870045 ) ) ;
#3683=CARTESIAN_POINT ( 'NONE',  ( 35.40819381912344710, 149.2475623141791061, -26.91697313366099920 ) ) ;
#3686=ORIENTED_EDGE ( 'NONE', *, *, #10335, .F. ) ;
#3688=CARTESIAN_POINT ( 'NONE',  ( 24.87028194210262910, 29.86925052300016858, -6.309743549972420595 ) ) ;
#3690=DIRECTION ( 'NONE',  ( 1.000000000000000000, 0.000000000000000000, 0.000000000000000000 ) ) ;
#3692=CARTESIAN_POINT ( 'NONE',  ( -17.68452897573239824, 32.19524659542067013, -8.268362122121875046 ) ) ;
#3694=DIRECTION ( 'NONE',  ( 0.000000000000000000, 0.000000000000000000, -1.000000000000000000 ) ) ;
#3696=EDGE_LOOP ( 'NONE', ( #14809, #2667, #9669, #11653 ) ) ;
#3697=ADVANCED_FACE ( 'NONE', ( #10615 ), #13545, .F. ) ;
#3698=CYLINDRICAL_SURFACE ( 'NONE', #16338, 2.499999999999998668 ) ;
#3699=DIRECTION ( 'NONE',  ( -2.674902700537819740E-31, 2.312964634635742267E-15, -1.000000000000000000 ) ) ;
#3704=CARTESIAN_POINT ( 'NONE',  ( -81.98700384596276081, 140.9569246592376714, -16.87109569490920435 ) ) ;
#3706=DIRECTION ( 'NONE',  ( 0.000000000000000000, 0.000000000000000000, 1.000000000000000000 ) ) ;
#3707=EDGE_CURVE ( 'NONE', #7553, #399, #5892, .T. ) ;
#3710=PLANE ( 'NONE',  #3949 ) ;
#3713=CARTESIAN_POINT ( 'NONE',  ( 28.96355834781382654, 202.5339273643436400, -16.41656018636075487 ) ) ;
#3720=CARTESIAN_POINT ( 'NONE',  ( -82.21997260166017440, 152.2013812635045156, -29.11730325185374113 ) ) ;
#3721=CARTESIAN_POINT ( 'NONE',  ( 18.30724418481818461, 142.5286147297794344, -15.57621362570774437 ) ) ;
#3726=CARTESIAN_POINT ( 'NONE',  ( 48.00000000000000711, 175.6227766016838530, -19.42820660268601074 ) ) ;
#3728=CARTESIAN_POINT ( 'NONE',  ( 24.00000000000000355, 146.6227766016838245, -35.00000000000000000 ) ) ;
#3729=FACE_OUTER_BOUND ( 'NONE', #5733, .T. ) ;
#3732=CARTESIAN_POINT ( 'NONE',  ( 48.00000000000000000, 171.6227766016838245, -10.00000337241048953 ) ) ;
#3735=VERTEX_POINT ( 'NONE', #1421 ) ;
#3736=DIRECTION ( 'NONE',  ( -1.000000000000000000, 0.000000000000000000, 0.000000000000000000 ) ) ;
#3737=LINE ( 'NONE', #14526, #3292 ) ;
#3739=ORIENTED_EDGE ( 'NONE', *, *, #11134, .F. ) ;
#3742=LINE ( 'NONE', #14533, #15543 ) ;
#3743=ORIENTED_EDGE ( 'NONE', *, *, #460, .T. ) ;
#3745=CARTESIAN_POINT ( 'NONE',  ( 25.11153254487453879, 190.9286879163519188, -26.76420670456568729 ) ) ;
#3746=FACE_OUTER_BOUND ( 'NONE', #6834, .T. ) ;
#3747=CARTESIAN_POINT ( 'NONE',  ( -12.63209758636618396, 17.99999999999999289, -7.167151760391626603 ) ) ;
#3748=VERTEX_POINT ( 'NONE', #7778 ) ;
#3749=DIRECTION ( 'NONE',  ( -1.000000000000000000, 0.000000000000000000, 0.000000000000000000 ) ) ;
#3751=CARTESIAN_POINT ( 'NONE',  ( 35.54773459694453663, 194.3303362407250461, -26.63481108765544647 ) ) ;
#3755=ADVANCED_FACE ( 'NONE', ( #5485 ), #15033, .T. ) ;
#3758=VERTEX_POINT ( 'NONE', #11229 ) ;
#3759=DIRECTION ( 'NONE',  ( -1.000000000000000000, -0.000000000000000000, 0.000000000000000000 ) ) ;
#3760=ORIENTED_EDGE ( 'NONE', *, *, #13785, .F. ) ;
#3763=LINE ( 'NONE', #9153, #4505 ) ;
#3765=CARTESIAN_POINT ( 'NONE',  ( -86.00000000000002842, 146.6227766016838245, -24.49489742783179480 ) ) ;
#3766=ORIENTED_EDGE ( 'NONE', *, *, #9520, .F. ) ;
#3769=CARTESIAN_POINT ( 'NONE',  ( 37.99999999999999289, 2.000000000000000000, 0.000000000000000000 ) ) ;
#3771=CARTESIAN_POINT ( 'NONE',  ( -27.99999999999998224, 10.00000000000000000, 0.000000000000000000 ) ) ;
#3773=LINE ( 'NONE', #9259, #11466 ) ;
#3779=SURFACE_STYLE_FILL_AREA ( #14580 ) ;
#3781=CARTESIAN_POINT ( 'NONE',  ( -85.49442651926489134, 144.1870492754457302, -21.73814637783849690 ) ) ;
#3782=B_SPLINE_CURVE_WITH_KNOTS ( 'NONE', 3,
 ( #12505, #3296, #8333, #8521, #14012, #372, #10996, #13929, #1791, #16419, #13748, #16583, #14105, #4457, #7021, #4282, #12420, #9843, #12588, #4713, #14447, #3470 ),
 .UNSPECIFIED., .F., .F.,
 ( 4, 2, 2, 2, 2, 2, 2, 2, 2, 2, 4 ),
 ( 0.000000000000000000, 0.003698315653799323904, 0.007396631307598647807, 0.01109494696139797128, 0.01479326261519729561, 0.01664242044209697166, 0.01849157826899665291, 0.02218989392279601541, 0.02403905174969570360, 0.02588820957659539179, 0.02958652523039474735 ),
 .UNSPECIFIED. ) ;
#3788=DIRECTION ( 'NONE',  ( -1.000000000000000000, -0.000000000000000000, 0.000000000000000000 ) ) ;
#3791=CARTESIAN_POINT ( 'NONE',  ( 35.49808778828385414, 199.0501964078081016, -21.74862058155258282 ) ) ;
#3792=EDGE_LOOP ( 'NONE', ( #11666, #12149, #1078 ) ) ;
#3793=VERTEX_POINT ( 'NONE', #1587 ) ;
#3794=CARTESIAN_POINT ( 'NONE',  ( 7.559396570614633326, 133.9010074147453508, -14.92908841323498770 ) ) ;
#3795=VECTOR ( 'NONE', #7709, 1000.000000000000000 ) ;
#3797=CARTESIAN_POINT ( 'NONE',  ( -86.00000000000001421, 146.9394831494155937, -24.81813469455733667 ) ) ;
#3798=EDGE_CURVE ( 'NONE', #8505, #1185, #8301, .T. ) ;
#3799=CARTESIAN_POINT ( 'NONE',  ( 8.997728150919979129, 132.8900016178789372, -12.55705910147062099 ) ) ;
#3802=CARTESIAN_POINT ( 'NONE',  ( 196.0000000000000000, 183.6227766016837961, -5.571800142134975431 ) ) ;
#3804=CARTESIAN_POINT ( 'NONE',  ( 24.72505082391212028, 201.9542783778900059, -13.00000000000000000 ) ) ;
#3807=AXIS2_PLACEMENT_3D ( 'NONE', #10623, #3912, #10267 ) ;
#3809=CARTESIAN_POINT ( 'NONE',  ( 23.09107716925733911, 18.00000000000000355, -5.000000000000003553 ) ) ;
#3811=CARTESIAN_POINT ( 'NONE',  ( -80.00000000000002842, 146.6227766016838245, -35.00200000000000244 ) ) ;
#3815=CARTESIAN_POINT ( 'NONE',  ( 24.16536605930837212, 145.1786002333612089, -22.93437194230014242 ) ) ;
#3820=EDGE_CURVE ( 'NONE', #6443, #10551, #16911, .T. ) ;
#3821=CARTESIAN_POINT ( 'NONE',  ( -20.85266279178582138, 18.00000000000000000, -20.15433268689461954 ) ) ;
#3823=EDGE_CURVE ( 'NONE', #9326, #730, #1649, .T. ) ;
#3824=CARTESIAN_POINT ( 'NONE',  ( -68.00000000000000000, 171.6227766016838245, -20.00000000000000355 ) ) ;
#3831=CIRCLE ( 'NONE', #2124, 8.000000000000000000 ) ;
#3832=AXIS2_PLACEMENT_3D ( 'NONE', #5185, #15987, #16179 ) ;
#3835=CARTESIAN_POINT ( 'NONE',  ( 22.50000000000000711, 196.2479045481293269, -21.97573418327509742 ) ) ;
#3836=FACE_OUTER_BOUND ( 'NONE', #3580, .T. ) ;
#3838=CARTESIAN_POINT ( 'NONE',  ( -11.31385407355777950, 31.26810920821015216, -12.21116371260378308 ) ) ;
#3844=CARTESIAN_POINT ( 'NONE',  ( 24.10475933960641370, 195.4942584061381865, -25.59693137756977421 ) ) ;
#3846=B_SPLINE_CURVE_WITH_KNOTS ( 'NONE', 3,
 ( #9511, #1647, #13776, #8275, #5718, #11107, #16518, #4390, #7130, #12529, #395, #11190, #1813, #14922, #5796, #2800, #16609, #483, #10845, #8193, #1476, #12264, #137, #10928, #16351 ),
 .UNSPECIFIED., .F., .F.,
 ( 4, 2, 2, 1, 2, 2, 2, 2, 2, 2, 2, 2, 4 ),
 ( 0.000000000000000000, 0.003937549356687076833, 0.005906324035030613949, 0.007875098713374151932, 0.009843873391717689048, 0.01181264807006122616, 0.01575019742674830733, 0.01771897210509184445, 0.01968774678343538503, 0.02362529614012245927, 0.02559407081846599985, 0.02756284549680953697, 0.03150039485349661467 ),
 .UNSPECIFIED. ) ;
#3848=ORIENTED_EDGE ( 'NONE', *, *, #13272, .T. ) ;
#3854=CIRCLE ( 'NONE', #12326, 30.00000000000000000 ) ;
#3855=EDGE_LOOP ( 'NONE', ( #3153, #2014, #10255, #1909 ) ) ;
#3857=VECTOR ( 'NONE', #3672, 1000.000000000000000 ) ;
#3859=CARTESIAN_POINT ( 'NONE',  ( 25.17791007590961172, 150.1982800653300387, -27.67726561134454144 ) ) ;
#3860=ADVANCED_FACE ( 'NONE', ( #16470 ), #12215, .F. ) ;
#3865=ORIENTED_EDGE ( 'NONE', *, *, #2879, .F. ) ;
#3869=CARTESIAN_POINT ( 'NONE',  ( -100.0000000000000000, 120.0000000000000284, -6.000000000000001776 ) ) ;
#3871=VERTEX_POINT ( 'NONE', #12477 ) ;
#3878=CARTESIAN_POINT ( 'NONE',  ( -40.00000000000000000, 20.00000000000000000, -28.00000000000000355 ) ) ;
#3883=CARTESIAN_POINT ( 'NONE',  ( -100.0000000000000000, 143.0439382767972347, -16.49999999999984368 ) ) ;
#3891=CARTESIAN_POINT ( 'NONE',  ( 35.49999999999998579, 9.999999999999998224, -35.00200000000000244 ) ) ;
#3893=ORIENTED_EDGE ( 'NONE', *, *, #3030, .F. ) ;
#3896=ORIENTED_EDGE ( 'NONE', *, *, #15638, .T. ) ;
#3898=FACE_BOUND ( 'NONE', #16396, .T. ) ;
#3900=CARTESIAN_POINT ( 'NONE',  ( 13.35668486245713282, 128.6964509245273405, -9.918424562684259982 ) ) ;
#3901=ORIENTED_EDGE ( 'NONE', *, *, #12113, .F. ) ;
#3903=CARTESIAN_POINT ( 'NONE',  ( 25.49999999999998579, 9.999999999999998224, -16.00000000000000000 ) ) ;
#3905=CARTESIAN_POINT ( 'NONE',  ( 22.56345771982927317, 197.7288430733995312, -20.20458554073936241 ) ) ;
#3907=DIRECTION ( 'NONE',  ( 0.000000000000000000, 0.000000000000000000, 1.000000000000000000 ) ) ;
#3908=CARTESIAN_POINT ( 'NONE',  ( 17.75267852353177034, 29.94338869414745830, -12.49131726690029254 ) ) ;
#3910=CARTESIAN_POINT ( 'NONE',  ( -100.0000000000000000, 141.6227766016838245, 0.000000000000000000 ) ) ;
#3912=DIRECTION ( 'NONE',  ( -0.000000000000000000, -0.000000000000000000, 1.000000000000000000 ) ) ;
#3916=CARTESIAN_POINT ( 'NONE',  ( 11.07991637643875116, 132.1496266960828336, -13.91448104906911709 ) ) ;
#3918=CARTESIAN_POINT ( 'NONE',  ( -80.00000000000001421, 196.6227766016838245, 1.387778780781445676E-14 ) ) ;
#3920=ADVANCED_FACE ( 'NONE', ( #12558 ), #12650, .F. ) ;
#3921=ORIENTED_EDGE ( 'NONE', *, *, #458, .F. ) ;
#3930=EDGE_CURVE ( 'NONE', #9467, #4581, #11658, .T. ) ;
#3931=DIRECTION ( 'NONE',  ( 1.000000000000000000, 0.000000000000000000, 0.000000000000000000 ) ) ;
#3932=FACE_OUTER_BOUND ( 'NONE', #9451, .T. ) ;
#3934=CARTESIAN_POINT ( 'NONE',  ( -15.37626115774789248, 32.49812920269235406, -8.581855491731886332 ) ) ;
#3935=EDGE_CURVE ( 'NONE', #11848, #12781, #13002, .T. ) ;
#3936=EDGE_CURVE ( 'NONE', #11405, #7894, #9852, .T. ) ;
#3937=ORIENTED_EDGE ( 'NONE', *, *, #10878, .F. ) ;
#3939=AXIS2_PLACEMENT_3D ( 'NONE', #15039, #1770, #2834 ) ;
#3941=ORIENTED_EDGE ( 'NONE', *, *, #10282, .F. ) ;
#3942=CARTESIAN_POINT ( 'NONE',  ( -87.47214505283551489, 195.8611292878214272, -22.40167687543583952 ) ) ;
#3949=AXIS2_PLACEMENT_3D ( 'NONE', #14501, #17335, #9441 ) ;
#3952=CIRCLE ( 'NONE', #4794, 9.999999999999998224 ) ;
#3954=AXIS2_PLACEMENT_3D ( 'NONE', #11673, #2121, #17006 ) ;
#3956=DIRECTION ( 'NONE',  ( 2.312964634635742464E-16, 0.000000000000000000, 1.000000000000000000 ) ) ;
#3961=CARTESIAN_POINT ( 'NONE',  ( 19.94005785806629660, 29.93324777864367192, -13.66280195656096907 ) ) ;
#3962=DIRECTION ( 'NONE',  ( -1.000000000000000000, -0.000000000000000000, -0.000000000000000000 ) ) ;
#3966=CARTESIAN_POINT ( 'NONE',  ( -85.59761955342212048, 141.6105225557631115, -13.74486639216964612 ) ) ;
#3967=AXIS2_PLACEMENT_3D ( 'NONE', #8293, #14939, #8031 ) ;
#3969=CARTESIAN_POINT ( 'NONE',  ( 49.99999999999998579, 175.6227766016838530, -19.42820660268601074 ) ) ;
#3977=CARTESIAN_POINT ( 'NONE',  ( 16.62686111071178630, 17.99999999999942801, -12.85442640772723344 ) ) ;
#3979=CARTESIAN_POINT ( 'NONE',  ( -84.06337902274010787, 142.1921853732337979, -18.94830881272694256 ) ) ;
#3980=CIRCLE ( 'NONE', #11317, 2.499999999999998668 ) ;
#3983=ORIENTED_EDGE ( 'NONE', *, *, #17160, .F. ) ;
#3986=DIRECTION ( 'NONE',  ( -1.000000000000000000, 0.000000000000000000, 0.000000000000000000 ) ) ;
#3988=EDGE_LOOP ( 'NONE', ( #1715, #11625, #16732, #16116 ) ) ;
#3990=CARTESIAN_POINT ( 'NONE',  ( 9.647168043681871197, 132.9898913927504225, -14.44632387683999575 ) ) ;
#3992=EDGE_CURVE ( 'NONE', #453, #14270, #12822, .T. ) ;
#3994=EDGE_LOOP ( 'NONE', ( #6545, #7729, #7726, #11711 ) ) ;
#3996=CIRCLE ( 'NONE', #4556, 5.000000000000000888 ) ;
#3997=CARTESIAN_POINT ( 'NONE',  ( 23.14977753070779087, 141.0007991078602743, -12.30735618844933832 ) ) ;
#3998=ORIENTED_EDGE ( 'NONE', *, *, #10405, .T. ) ;
#4002=DIRECTION ( 'NONE',  ( -1.000000000000000000, -0.000000000000000000, -0.000000000000000000 ) ) ;
#4003=CARTESIAN_POINT ( 'NONE',  ( 49.99999999999998579, 151.6227766016839098, -5.571800142134973655 ) ) ;
#4004=CARTESIAN_POINT ( 'NONE',  ( 21.99569976772868074, 17.99999999999999645, -9.076888812463767664 ) ) ;
#4007=DIRECTION ( 'NONE',  ( -1.000000000000000000, 0.000000000000000000, 0.000000000000000000 ) ) ;
#4009=DIRECTION ( 'NONE',  ( 1.000000000000000000, 0.000000000000000000, 0.000000000000000000 ) ) ;
#4010=ORIENTED_EDGE ( 'NONE', *, *, #1057, .T. ) ;
#4011=CARTESIAN_POINT ( 'NONE',  ( 16.69631138515844171, 126.9345490261019904, -8.565329098038530375 ) ) ;
#4016=ORIENTED_EDGE ( 'NONE', *, *, #8405, .F. ) ;
#4024=DIRECTION ( 'NONE',  ( -1.000000000000000000, -0.000000000000000000, 0.000000000000000000 ) ) ;
#4026=B_SPLINE_CURVE_WITH_KNOTS ( 'NONE', 3,
 ( #4979, #3835, #11790, #1177, #9315, #17195, #5070, #3567, #15875, #10548, #10470, #11694, #6488, #14538, #3745, #7806, #10371, #10646, #17107, #9132, #9225, #15782, #15956, #14634, #7902, #6581, #5243, #16055, #7549, #8962, #14373, #13483, #9484, #13393, #15056, #6917, #16231, #4189, #5341, #11077, #1615, #7015, #6762, #1357, #2683, #8071 ),
 .UNSPECIFIED., .F., .F.,
 ( 4, 2, 2, 2, 2, 2, 2, 2, 2, 2, 2, 2, 2, 2, 2, 2, 2, 2, 2, 2, 2, 2, 4 ),
 ( 0.01035378412632265502, 0.01206629175607490910, 0.01377879938582716318, 0.01549130701557941726, 0.01634756083045556946, 0.01720381464533172339, 0.01806006846020787732, 0.01891632227508402778, 0.02062882990483638768, 0.02148508371971258324, 0.02234133753458877880, 0.02319759134946497436, 0.02405384516434117687, 0.02576635279409356799, 0.02747886042384597299, 0.02833511423872216509, 0.02919136805359836065, 0.03090387568335074484, 0.03261638331310313943, 0.03432889094285552362, 0.03604139857260790780, 0.03689765238748410336, 0.03775390620236029199 ),
 .UNSPECIFIED. ) ;
#4029=EDGE_CURVE ( 'NONE', #4990, #13903, #10247, .T. ) ;
#4030=ORIENTED_EDGE ( 'NONE', *, *, #3638, .F. ) ;
#4031=ADVANCED_FACE ( 'NONE', ( #6092 ), #3263, .F. ) ;
#4033=LINE ( 'NONE', #10379, #3857 ) ;
#4034=ORIENTED_EDGE ( 'NONE', *, *, #3483, .F. ) ;
#4038=EDGE_CURVE ( 'NONE', #1489, #8410, #14077, .T. ) ;
#4039=ADVANCED_FACE ( 'NONE', ( #1938 ), #7339, .F. ) ;
#4042=CARTESIAN_POINT ( 'NONE',  ( 30.00000000000000355, 196.6227766016838245, -16.00000000000000000 ) ) ;
#4046=VERTEX_POINT ( 'NONE', #10163 ) ;
#4052=DIRECTION ( 'NONE',  ( 0.000000000000000000, 0.000000000000000000, 1.000000000000000000 ) ) ;
#4053=FACE_OUTER_BOUND ( 'NONE', #7266, .T. ) ;
#4056=EDGE_CURVE ( 'NONE', #8410, #5512, #9279, .T. ) ;
#4058=DIRECTION ( 'NONE',  ( 1.000000000000000000, 0.000000000000000000, 0.000000000000000000 ) ) ;
#4059=CARTESIAN_POINT ( 'NONE',  ( 17.00000000000000000, 154.3022685259950038, -9.999999999999900524 ) ) ;
#4060=CARTESIAN_POINT ( 'NONE',  ( -85.83463394069167407, 145.1786002333612089, -22.93437194230014242 ) ) ;
#4068=CARTESIAN_POINT ( 'NONE',  ( 26.57417986947462651, 137.5626638350942699, -8.060801806284990434 ) ) ;
#4073=CARTESIAN_POINT ( 'NONE',  ( 40.00000000000000711, 138.6227766016838245, -6.062001655779397722E-15 ) ) ;
#4074=CARTESIAN_POINT ( 'NONE',  ( -74.09940879757193954, 195.3277913626825466, -25.76530748039454721 ) ) ;
#4077=CARTESIAN_POINT ( 'NONE',  ( 28.15871609335591685, 18.00000000000000000, -20.05978710182010971 ) ) ;
#4078=CARTESIAN_POINT ( 'NONE',  ( 21.38389869590601933, 18.00000000000114753, -9.948751090973035005 ) ) ;
#4079=PLANE ( 'NONE',  #10369 ) ;
#4080=DIRECTION ( 'NONE',  ( 1.000000000000000000, 0.000000000000000000, 0.000000000000000000 ) ) ;
#4082=EDGE_CURVE ( 'NONE', #11435, #4527, #9271, .T. ) ;
#4088=CIRCLE ( 'NONE', #17371, 5.000000000000018652 ) ;
#4092=ORIENTED_EDGE ( 'NONE', *, *, #8714, .T. ) ;
#4093=DIRECTION ( 'NONE',  ( 1.000000000000000000, 0.000000000000000000, -0.000000000000000000 ) ) ;
#4098=ORIENTED_EDGE ( 'NONE', *, *, #9339, .T. ) ;
#4099=AXIS2_PLACEMENT_3D ( 'NONE', #16761, #1966, #1621 ) ;
#4101=CARTESIAN_POINT ( 'NONE',  ( -40.00000000000000000, 4.000000000000000000, -33.00000000000000711 ) ) ;
#4104=EDGE_LOOP ( 'NONE', ( #16302, #4921, #7544, #8832 ) ) ;
#4109=AXIS2_PLACEMENT_3D ( 'NONE', #1786, #9925, #16755 ) ;
#4124=CARTESIAN_POINT ( 'NONE',  ( -78.56757686808167307, 202.4505251070389704, -16.57269434321681345 ) ) ;
#4128=CARTESIAN_POINT ( 'NONE',  ( -32.99999999999998579, 10.00000000000000000, -35.00200000000000244 ) ) ;
#4132=CARTESIAN_POINT ( 'NONE',  ( 37.99999999999998579, 20.00000000000000000, -28.00000000000001066 ) ) ;
#4133=CIRCLE ( 'NONE', #13177, 248.0000000000000000 ) ;
#4135=CARTESIAN_POINT ( 'NONE',  ( 49.99999999999998579, 159.6227766016838814, -3.071800142134975431 ) ) ;
#4136=ORIENTED_EDGE ( 'NONE', *, *, #9547, .F. ) ;
#4138=CARTESIAN_POINT ( 'NONE',  ( 15.96677753504215858, 136.6227766016837961, -4.434194661153730915E-13 ) ) ;
#4139=EDGE_CURVE ( 'NONE', #6006, #16523, #2365, .T. ) ;
#4140=DIRECTION ( 'NONE',  ( -1.000000000000000000, -0.000000000000000000, -0.000000000000000000 ) ) ;
#4141=DIRECTION ( 'NONE',  ( 1.000000000000000000, 0.000000000000000000, 0.000000000000000000 ) ) ;
#4142=EDGE_CURVE ( 'NONE', #12705, #15849, #13301, .T. ) ;
#4143=VECTOR ( 'NONE', #2844, 1000.000000000000000 ) ;
#4144=VECTOR ( 'NONE', #1064, 1000.000000000000000 ) ;
#4146=FACE_OUTER_BOUND ( 'NONE', #12831, .T. ) ;
#4147=EDGE_CURVE ( 'NONE', #13207, #8108, #3069, .T. ) ;
#4151=FACE_OUTER_BOUND ( 'NONE', #3309, .T. ) ;
#4153=CARTESIAN_POINT ( 'NONE',  ( 14.43747245749253416, 129.4010981426196736, -11.63709869316310908 ) ) ;
#4156=CARTESIAN_POINT ( 'NONE',  ( 15.54198151645489645, 125.3641151175237667, -5.547502007357641318 ) ) ;
#4160=CARTESIAN_POINT ( 'NONE',  ( -81.12708499979228804, 190.7253031951458127, -29.32741221247050589 ) ) ;
#4162=CIRCLE ( 'NONE', #16875, 10.00000000000000000 ) ;
#4165=CARTESIAN_POINT ( 'NONE',  ( 27.99999999999998224, 9.999999999999998224, -16.00000000000000000 ) ) ;
#4166=CARTESIAN_POINT ( 'NONE',  ( 17.50698843878764777, 29.94827730614627725, -12.57924512168886011 ) ) ;
#4170=CARTESIAN_POINT ( 'NONE',  ( 26.52113164449903948, 141.7198527106616268, -18.19376952932830349 ) ) ;
#4172=CARTESIAN_POINT ( 'NONE',  ( 9.103003883573421717, 133.2684780490642709, -14.60854014130129030 ) ) ;
#4174=EDGE_LOOP ( 'NONE', ( #7685, #14413 ) ) ;
#4179=CARTESIAN_POINT ( 'NONE',  ( 49.99999999999998579, 183.6227766016837961, -5.571800142134975431 ) ) ;
#4181=ORIENTED_EDGE ( 'NONE', *, *, #6754, .T. ) ;
#4182=EDGE_CURVE ( 'NONE', #10541, #3188, #1096, .T. ) ;
#4184=CARTESIAN_POINT ( 'NONE',  ( 28.86500048027878051, 154.0589040539455823, -27.93804624201380804 ) ) ;
#4187=CIRCLE ( 'NONE', #14351, 35.00000000000000000 ) ;
#4188=DIRECTION ( 'NONE',  ( 1.000000000000000000, 0.000000000000000000, 0.000000000000000000 ) ) ;
#4189=CARTESIAN_POINT ( 'NONE',  ( 36.80495063319472138, 193.4351830419513476, -24.76910924193870400 ) ) ;
#4191=EDGE_LOOP ( 'NONE', ( #12028, #9079, #5805 ) ) ;
#4192=FACE_OUTER_BOUND ( 'NONE', #12058, .T. ) ;
#4198=CARTESIAN_POINT ( 'NONE',  ( -15.96992528024541613, 32.67167891243749978, -7.259156848219323166 ) ) ;
#4199=VECTOR ( 'NONE', #1550, 1000.000000000000000 ) ;
#4200=ORIENTED_EDGE ( 'NONE', *, *, #10540, .F. ) ;
#4203=EDGE_CURVE ( 'NONE', #3029, #15883, #5906, .T. ) ;
#4210=FACE_OUTER_BOUND ( 'NONE', #6693, .T. ) ;
#4212=DIRECTION ( 'NONE',  ( 0.000000000000000000, 0.000000000000000000, 1.000000000000000000 ) ) ;
#4213=CARTESIAN_POINT ( 'NONE',  ( 17.00000000000000000, 154.3022685259950038, -9.999999999999900524 ) ) ;
#4214=AXIS2_PLACEMENT_3D ( 'NONE', #9078, #6257, #10678 ) ;
#4216=VERTEX_POINT ( 'NONE', #2724 ) ;
#4219=DIRECTION ( 'NONE',  ( -0.000000000000000000, -0.000000000000000000, -1.000000000000000000 ) ) ;
#4220=DIRECTION ( 'NONE',  ( 1.000000000000000000, 0.000000000000000000, 0.000000000000000000 ) ) ;
#4226=VECTOR ( 'NONE', #2777, 1000.000000000000000 ) ;
#4228=DIRECTION ( 'NONE',  ( 1.000000000000000000, 0.000000000000000000, 0.000000000000000000 ) ) ;
#4229=AXIS2_PLACEMENT_3D ( 'NONE', #9572, #6667, #14891 ) ;
#4234=VERTEX_POINT ( 'NONE', #13696 ) ;
#4235=FACE_OUTER_BOUND ( 'NONE', #17188, .T. ) ;
#4237=LINE ( 'NONE', #6973, #2544 ) ;
#4242=CARTESIAN_POINT ( 'NONE',  ( 16.17648631192976794, 127.5693673001539992, -9.524520547909567370 ) ) ;
#4250=EDGE_CURVE ( 'NONE', #6671, #17520, #17498, .T. ) ;
#4251=CIRCLE ( 'NONE', #13300, 2.499999999999998668 ) ;
#4255=DIRECTION ( 'NONE',  ( -0.000000000000000000, -0.000000000000000000, -1.000000000000000000 ) ) ;
#4258=CARTESIAN_POINT ( 'NONE',  ( 37.99999999999998579, 18.00000000000000355, -28.00000000000001066 ) ) ;
#4259=CARTESIAN_POINT ( 'NONE',  ( 13.57836111649853450, 143.5532840108684525, -17.35359164609418059 ) ) ;
#4260=DIRECTION ( 'NONE',  ( 0.000000000000000000, 0.000000000000000000, -1.000000000000000000 ) ) ;
#4261=ORIENTED_EDGE ( 'NONE', *, *, #4986, .F. ) ;
#4262=CARTESIAN_POINT ( 'NONE',  ( -14.90344812367259131, 20.00000000000343192, -8.058388986520416353 ) ) ;
#4265=CARTESIAN_POINT ( 'NONE',  ( 24.29786737972285238, 29.87659578631513568, -8.527395788633878482 ) ) ;
#4270=CARTESIAN_POINT ( 'NONE',  ( 15.00000000000000000, 171.6227766016838245, -20.00000000000000355 ) ) ;
#4271=ORIENTED_EDGE ( 'NONE', *, *, #4400, .T. ) ;
#4272=CARTESIAN_POINT ( 'NONE',  ( 36.98037184620995532, 149.3990418665993047, -24.40116746791568758 ) ) ;
#4273=EDGE_CURVE ( 'NONE', #793, #1279, #7586, .T. ) ;
#4274=CIRCLE ( 'NONE', #16985, 5.000000000000004441 ) ;
#4277=DIRECTION ( 'NONE',  ( 1.000000000000000000, 0.000000000000000000, -0.000000000000000000 ) ) ;
#4278=CARTESIAN_POINT ( 'NONE',  ( -725.0000000000001137, 129.9999999999995453, -4.999999999999999112 ) ) ;
#4279=ORIENTED_EDGE ( 'NONE', *, *, #16848, .T. ) ;
#4282=CARTESIAN_POINT ( 'NONE',  ( 12.82244027866276426, 141.9777490571136696, -18.60671400555900235 ) ) ;
#4283=EDGE_CURVE ( 'NONE', #3210, #7915, #6759, .T. ) ;
#4284=VERTEX_POINT ( 'NONE', #11037 ) ;
#4285=CARTESIAN_POINT ( 'NONE',  ( -76.21324911630662768, 190.1432158455537262, -27.31345131271291038 ) ) ;
#4291=LINE ( 'NONE', #1720, #9202 ) ;
#4292=B_SPLINE_CURVE_WITH_KNOTS ( 'NONE', 3,
 ( #12147, #12400, #4344, #16401 ),
 .UNSPECIFIED., .F., .F.,
 ( 4, 4 ),
 ( 0.000000000000000000, 0.001170341053039947524 ),
 .UNSPECIFIED. ) ;
#4293=CARTESIAN_POINT ( 'NONE',  ( -72.78662571002521986, 198.7412861714591088, -18.82352572523460310 ) ) ;
#4295=VERTEX_POINT ( 'NONE', #12461 ) ;
#4301=ORIENTED_EDGE ( 'NONE', *, *, #1958, .F. ) ;
#4305=DIRECTION ( 'NONE',  ( -1.000000000000000000, -0.000000000000000000, 0.000000000000000000 ) ) ;
#4308=DIRECTION ( 'NONE',  ( -6.938893903907228378E-16, 1.000000000000000000, 0.000000000000000000 ) ) ;
#4312=EDGE_LOOP ( 'NONE', ( #5379, #62, #14990, #11609 ) ) ;
#4313=DIRECTION ( 'NONE',  ( -0.000000000000000000, -0.000000000000000000, 1.000000000000000000 ) ) ;
#4314=ORIENTED_EDGE ( 'NONE', *, *, #1484, .T. ) ;
#4316=ORIENTED_EDGE ( 'NONE', *, *, #6851, .T. ) ;
#4319=DIRECTION ( 'NONE',  ( -1.000000000000000000, 0.000000000000000000, 0.000000000000000000 ) ) ;
#4326=CARTESIAN_POINT ( 'NONE',  ( 15.95013150516294154, 137.1612117474554111, -8.111885438162047990 ) ) ;
#4327=VERTEX_POINT ( 'NONE', #15627 ) ;
#4329=CARTESIAN_POINT ( 'NONE',  ( 13.90347339350139677, 138.7488974902626069, -3.510692536283880116 ) ) ;
#4330=VERTEX_POINT ( 'NONE', #7320 ) ;
#4331=CARTESIAN_POINT ( 'NONE',  ( -84.70068968583443336, 192.8887977548965296, -27.79913727548661839 ) ) ;
#4333=EDGE_CURVE ( 'NONE', #7814, #3299, #17204, .T. ) ;
#4335=EDGE_CURVE ( 'NONE', #17412, #14332, #1945, .T. ) ;
#4336=DIRECTION ( 'NONE',  ( -1.000000000000000000, 0.000000000000000000, 0.000000000000000000 ) ) ;
#4338=FACE_OUTER_BOUND ( 'NONE', #10292, .T. ) ;
#4339=CARTESIAN_POINT ( 'NONE',  ( 9.156206820864191798, 144.1010407228830559, -18.21082046960973599 ) ) ;
#4344=CARTESIAN_POINT ( 'NONE',  ( 15.39006516123636281, 143.0404737187717785, -16.50200026350847793 ) ) ;
#4348=VERTEX_POINT ( 'NONE', #3243 ) ;
#4349=CARTESIAN_POINT ( 'NONE',  ( 22.74938895237542624, 148.5880153409832189, -23.63707964515040061 ) ) ;
#4351=CIRCLE ( 'NONE', #5653, 7.499999999999996447 ) ;
#4355=CARTESIAN_POINT ( 'NONE',  ( -5.000000000000000888, 191.6227766016837961, 1.224646799147353454E-15 ) ) ;
#4356=DIRECTION ( 'NONE',  ( -0.000000000000000000, -0.000000000000000000, 1.000000000000000000 ) ) ;
#4357=B_SPLINE_CURVE_WITH_KNOTS ( 'NONE', 3,
 ( #16408, #5506, #9831, #5685, #5853, #4272, #12314, #6912, #191, #15053, #16489, #4537, #11151, #12233, #15323, #12578, #9655, #8320, #8246, #7176, #2851, #10894, #11247, #13736, #1611, #16313, #4184, #16667, #4446, #9568, #7010, #8418, #12408, #3198, #5764, #12497, #14974, #13652, #8590, #4349, #9921, #1443, #6842, #9738, #15138, #3018 ),
 .UNSPECIFIED., .F., .F.,
 ( 4, 2, 2, 2, 2, 2, 2, 2, 2, 2, 2, 2, 2, 2, 2, 2, 2, 2, 2, 2, 2, 2, 4 ),
 ( 0.01035378412632265502, 0.01206629175607499757, 0.01377879938582734186, 0.01549130701557968615, 0.01634756083045588171, 0.01720381464533208074, 0.01806006846020827977, 0.01891632227508447534, 0.02062882990483680748, 0.02148508371971298223, 0.02234133753458915697, 0.02319759134946533172, 0.02405384516434150993, 0.02576635279409385942, 0.02747886042384620545, 0.02833511423872238019, 0.02919136805359855841, 0.03090387568335089402, 0.03261638331310323657, 0.03432889094285557913, 0.03604139857260792168, 0.03689765238748408949, 0.03775390620236026423 ),
 .UNSPECIFIED. ) ;
#4359=DIRECTION ( 'NONE',  ( -1.000000000000000000, -0.000000000000000000, -0.000000000000000000 ) ) ;
#4360=ORIENTED_EDGE ( 'NONE', *, *, #9371, .T. ) ;
#4366=DIRECTION ( 'NONE',  ( 1.000000000000000000, 0.000000000000000000, -0.000000000000000000 ) ) ;
#4369=EDGE_LOOP ( 'NONE', ( #12572, #14160, #7511, #11246, #755, #6063 ) ) ;
#4370=VERTEX_POINT ( 'NONE', #7480 ) ;
#4372=CIRCLE ( 'NONE', #5767, 7.500000000000000000 ) ;
#4373=AXIS2_PLACEMENT_3D ( 'NONE', #14656, #6601, #11265 ) ;
#4378=CYLINDRICAL_SURFACE ( 'NONE', #28, 2.499999999999998668 ) ;
#4380=DIRECTION ( 'NONE',  ( 0.000000000000000000, 0.000000000000000000, 1.000000000000000000 ) ) ;
#4384=CARTESIAN_POINT ( 'NONE',  ( 37.99999999999999289, 18.00000000000000355, -8.789265611615818404E-15 ) ) ;
#4385=AXIS2_PLACEMENT_3D ( 'NONE', #15592, #3467, #8854 ) ;
#4386=EDGE_LOOP ( 'NONE', ( #16515, #15678, #7445, #11296 ) ) ;
#4388=AXIS2_PLACEMENT_3D ( 'NONE', #11350, #3026, #4628 ) ;
#4389=CYLINDRICAL_SURFACE ( 'NONE', #14442, 2.500000000000000444 ) ;
#4390=CARTESIAN_POINT ( 'NONE',  ( 23.79315516583586643, 19.99999999999999645, -22.94240041036162836 ) ) ;
#4391=CARTESIAN_POINT ( 'NONE',  ( 36.00000000000000711, 196.6227766016838245, -16.00000000000000000 ) ) ;
#4392=CARTESIAN_POINT ( 'NONE',  ( 30.00000000000001066, 146.6227766016838245, -13.00000000000000000 ) ) ;
#4394=ORIENTED_EDGE ( 'NONE', *, *, #5331, .F. ) ;
#4395=FACE_OUTER_BOUND ( 'NONE', #7602, .T. ) ;
#4400=EDGE_CURVE ( 'NONE', #8669, #17476, #7878, .T. ) ;
#4406=VECTOR ( 'NONE', #5909, 1000.000000000000000 ) ;
#4409=CARTESIAN_POINT ( 'NONE',  ( -85.27494917608791525, 201.9542783778900059, -13.00000000000000000 ) ) ;
#4414=CARTESIAN_POINT ( 'NONE',  ( 37.99999999999999289, 18.00000000000000355, 0.000000000000000000 ) ) ;
#4416=VECTOR ( 'NONE', #10930, 1000.000000000000000 ) ;
#4418=CARTESIAN_POINT ( 'NONE',  ( -95.00000000000000000, 141.6227766016838245, 5.510910596163088767E-15 ) ) ;
#4419=VERTEX_POINT ( 'NONE', #17045 ) ;
#4428=DIRECTION ( 'NONE',  ( 1.000000000000000000, 0.000000000000000000, 0.000000000000000000 ) ) ;
#4429=CARTESIAN_POINT ( 'NONE',  ( 22.99999999999997868, 9.999999999999998224, -35.00200000000000244 ) ) ;
#4430=LINE ( 'NONE', #2916, #16036 ) ;
#4438=VECTOR ( 'NONE', #9203, 1000.000000000000000 ) ;
#4439=DIRECTION ( 'NONE',  ( 1.000000000000000000, 0.000000000000000000, 0.000000000000000000 ) ) ;
#4444=FACE_OUTER_BOUND ( 'NONE', #9576, .T. ) ;
#4446=CARTESIAN_POINT ( 'NONE',  ( 27.20631483639104076, 153.6052450214444889, -27.64877209012308512 ) ) ;
#4451=TOROIDAL_SURFACE ( 'NONE', #2460, 740.0000000000000000, 8.000000000000000000 ) ;
#4453=MECHANICAL_DESIGN_GEOMETRIC_PRESENTATION_REPRESENTATION('',(#10112),#3313);
#4457=CARTESIAN_POINT ( 'NONE',  ( 15.72080254704531477, 141.4281235329943343, -17.70852598599439176 ) ) ;
#4458=ORIENTED_EDGE ( 'NONE', *, *, #6526, .T. ) ;
#4459=LINE ( 'NONE', #3300, #12407 ) ;
#4461=ORIENTED_EDGE ( 'NONE', *, *, #3539, .T. ) ;
#4470=CARTESIAN_POINT ( 'NONE',  ( -34.99999999999999289, 130.0000000000000000, 0.000000000000000000 ) ) ;
#4471=EDGE_CURVE ( 'NONE', #12970, #4801, #2261, .T. ) ;
#4472=CARTESIAN_POINT ( 'NONE',  ( -96.00000000000001421, 171.6227766016838245, 0.000000000000000000 ) ) ;
#4480=CARTESIAN_POINT ( 'NONE',  ( -74.16379527187788767, 198.0598900292995097, -22.94241666008129243 ) ) ;
#4481=CARTESIAN_POINT ( 'NONE',  ( -86.00000000000001421, 196.6227766016838245, -16.00000000000000000 ) ) ;
#4485=CARTESIAN_POINT ( 'NONE',  ( -80.00000000000001421, 196.6227766016838245, -35.00200000000000244 ) ) ;
#4486=ORIENTED_EDGE ( 'NONE', *, *, #3930, .T. ) ;
#4489=VERTEX_POINT ( 'NONE', #2343 ) ;
#4490=FACE_OUTER_BOUND ( 'NONE', #15698, .T. ) ;
#4492=ORIENTED_EDGE ( 'NONE', *, *, #15369, .F. ) ;
#4494=FACE_OUTER_BOUND ( 'NONE', #8956, .T. ) ;
#4497=FACE_OUTER_BOUND ( 'NONE', #9359, .T. ) ;
#4499=CARTESIAN_POINT ( 'NONE',  ( 196.0000000000000000, 167.6227766016838814, -21.92820660268601074 ) ) ;
#4500=DIRECTION ( 'NONE',  ( 0.000000000000000000, 0.000000000000000000, 1.000000000000000000 ) ) ;
#4504=EDGE_CURVE ( 'NONE', #16539, #11464, #6554, .T. ) ;
#4505=VECTOR ( 'NONE', #5178, 1000.000000000000000 ) ;
#4512=CARTESIAN_POINT ( 'NONE',  ( 30.00000000000001066, 146.6227766016838245, -16.00000000000000000 ) ) ;
#4513=CIRCLE ( 'NONE', #12714, 33.00000000000000000 ) ;
#4515=CARTESIAN_POINT ( 'NONE',  ( -68.00000000000000000, 171.6227766016838245, 0.000000000000000000 ) ) ;
#4516=VECTOR ( 'NONE', #8440, 1000.000000000000000 ) ;
#4517=LINE ( 'NONE', #4429, #9999 ) ;
#4521=DIRECTION ( 'NONE',  ( 0.000000000000000000, 0.000000000000000000, 1.000000000000000000 ) ) ;
#4523=( BOUNDED_SURFACE ( )  B_SPLINE_SURFACE ( 3, 2, ( 
 ( #479, #16695, #4564 ),
 ( #14035, #9949, #3224 ),
 ( #4644, #15439, #11974 ),
 ( #17029, #3570, #15877 ),
 ( #918, #2326, #993 ),
 ( #8964, #16057, #2509 ),
 ( #7718, #6491, #13128 ),
 ( #3838, #10550, #2244 ),
 ( #6669, #7905, #6305 ),
 ( #6397, #11697, #17109 ),
 ( #5073, #14636, #9318 ),
 ( #11792, #4982, #9228 ),
 ( #1089, #2604, #10285 ),
 ( #14541, #7810, #11885 ),
 ( #9134, #17197, #10472 ),
 ( #15686, #1179, #4894 ),
 ( #5164, #17294, #13048 ),
 ( #3934, #3747, #14730 ),
 ( #10650, #7990, #13396 ),
 ( #13314, #2412, #10373 ),
 ( #14460, #5245, #13220 ),
 ( #15958, #1264, #14375 ),
 ( #6583, #15784, #17375 ),
 ( #7637, #3666, #9055 ) ),
 .UNSPECIFIED., .F., .F., .F. ) 
 B_SPLINE_SURFACE_WITH_KNOTS ( ( 4, 2, 2, 2, 2, 2, 2, 2, 2, 2, 2, 4 ),
 ( 3, 3 ),
 ( 0.01427588378380421734, 0.01824401167166928364, 0.02022807561560181766, 0.02221213955953435168, 0.02618026744739941625, 0.02816433139133195027, 0.03014839533526448428, 0.03411652322312955232, 0.03610058716706208287, 0.03808465111099461342, 0.04205277899885968146, 0.04602090688672474950 ),
 ( 0.000000000000000000, 1.000000000000000000 ),
 .UNSPECIFIED. ) 
 GEOMETRIC_REPRESENTATION_ITEM ( )  RATIONAL_B_SPLINE_SURFACE ( (
 ( 1.000000000000000000, 0.7071067811865476838, 1.000000000000000000),
 ( 1.000000000000000000, 0.7013659285812973154, 1.000000000000000000),
 ( 1.000000000000000000, 0.6957352470445186121, 1.000000000000000000),
 ( 1.000000000000000000, 0.6874449304734518984, 1.000000000000000000),
 ( 1.000000000000000000, 0.6847075230360146758, 1.000000000000000000),
 ( 1.000000000000000000, 0.6792848743381181276, 1.000000000000000000),
 ( 1.000000000000000000, 0.6765866164120997173, 1.000000000000000000),
 ( 1.000000000000000000, 0.6687223666255138754, 1.000000000000000000),
 ( 1.000000000000000000, 0.6637534122519734847, 1.000000000000000000),
 ( 1.000000000000000000, 0.6567012635109988894, 1.000000000000000000),
 ( 1.000000000000000000, 0.6544178910916050862, 1.000000000000000000),
 ( 1.000000000000000000, 0.6499901663948596253, 1.000000000000000000),
 ( 1.000000000000000000, 0.6478648508490586488, 1.000000000000000000),
 ( 1.000000000000000000, 0.6418284244075036504, 1.000000000000000000),
 ( 1.000000000000000000, 0.6382188548936987837, 1.000000000000000000),
 ( 1.000000000000000000, 0.6334349500989925330, 1.000000000000000000),
 ( 1.000000000000000000, 0.6319385063093012622, 1.000000000000000000),
 ( 1.000000000000000000, 0.6292162870120669993, 1.000000000000000000),
 ( 1.000000000000000000, 0.6279881568153810045, 1.000000000000000000),
 ( 1.000000000000000000, 0.6246939197237914021, 1.000000000000000000),
 ( 1.000000000000000000, 0.6230139244306683866, 1.000000000000000000),
 ( 1.000000000000000000, 0.6207349535630238835, 1.000000000000000000),
 ( 1.000000000000000000, 0.6201739322038456459, 1.000000000000000000),
 ( 1.000000000000000000, 0.6201736729460424202, 1.000000000000000000) ) ) 
 REPRESENTATION_ITEM ( '' )  SURFACE ( )  );
#4524=EDGE_CURVE ( 'NONE', #6195, #14777, #3379, .T. ) ;
#4525=EDGE_CURVE ( 'NONE', #4801, #4546, #3763, .T. ) ;
#4527=VERTEX_POINT ( 'NONE', #50 ) ;
#4528=CARTESIAN_POINT ( 'NONE',  ( 34.93420767853318409, 19.99999999999999645, -5.000000000000010658 ) ) ;
#4531=CARTESIAN_POINT ( 'NONE',  ( 26.66247177481912800, 139.4607352144954007, -7.398570892697257761 ) ) ;
#4532=ORIENTED_EDGE ( 'NONE', *, *, #5052, .T. ) ;
#4533=CARTESIAN_POINT ( 'NONE',  ( 196.0000000000000000, 159.6227766016838814, -5.571800142134975431 ) ) ;
#4536=ORIENTED_EDGE ( 'NONE', *, *, #16829, .T. ) ;
#4537=CARTESIAN_POINT ( 'NONE',  ( 35.62055130997416796, 151.5947363889490589, -26.22852547856964378 ) ) ;
#4539=DIRECTION ( 'NONE',  ( 0.000000000000000000, 0.000000000000000000, 1.000000000000000000 ) ) ;
#4545=CARTESIAN_POINT ( 'NONE',  ( -74.10793207926305115, 141.9594008680238062, -14.48313018527311868 ) ) ;
#4546=VERTEX_POINT ( 'NONE', #16438 ) ;
#4548=ORIENTED_EDGE ( 'NONE', *, *, #10556, .T. ) ;
#4549=PLANE ( 'NONE',  #3651 ) ;
#4552=DIRECTION ( 'NONE',  ( -1.000000000000000000, -0.000000000000000000, 0.000000000000000000 ) ) ;
#4553=AXIS2_PLACEMENT_3D ( 'NONE', #7129, #12528, #393 ) ;
#4556=AXIS2_PLACEMENT_3D ( 'NONE', #17489, #2872, #8267 ) ;
#4559=LINE ( 'NONE', #11274, #441 ) ;
#4560=CARTESIAN_POINT ( 'NONE',  ( 30.00000000000001066, 146.6227766016838245, -35.00000000000000000 ) ) ;
#4561=CARTESIAN_POINT ( 'NONE',  ( -3.000000000000000888, 171.6227766016838245, -20.00000000000000355 ) ) ;
#4564=CARTESIAN_POINT ( 'NONE',  ( -7.379000772444995526, 18.00000000000000000, -25.00000000000000000 ) ) ;
#4565=EDGE_CURVE ( 'NONE', #6476, #16806, #9012, .T. ) ;
#4566=VERTEX_POINT ( 'NONE', #16343 ) ;
#4568=AXIS2_PLACEMENT_3D ( 'NONE', #13657, #2508, #14807 ) ;
#4569=DIRECTION ( 'NONE',  ( 0.000000000000000000, -1.000000000000000000, -6.123233995736762338E-17 ) ) ;
#4572=CARTESIAN_POINT ( 'NONE',  ( 50.00000000000000000, 171.6227766016838245, 0.000000000000000000 ) ) ;
#4576=EDGE_CURVE ( 'NONE', #4327, #12781, #14914, .T. ) ;
#4578=ORIENTED_EDGE ( 'NONE', *, *, #12564, .T. ) ;
#4579=CARTESIAN_POINT ( 'NONE',  ( -68.00000000000000000, 171.6227766016838245, 0.000000000000000000 ) ) ;
#4581=VERTEX_POINT ( 'NONE', #5366 ) ;
#4582=DIRECTION ( 'NONE',  ( -1.000000000000000000, 0.000000000000000000, 0.000000000000000000 ) ) ;
#4585=LINE ( 'NONE', #2013, #11175 ) ;
#4588=DIRECTION ( 'NONE',  ( -0.01578383822436034076, 0.1110972697184772484, -0.9936841888205766304 ) ) ;
#4590=CARTESIAN_POINT ( 'NONE',  ( -12.77984573873758656, 20.00000000000345679, -11.87289823213939854 ) ) ;
#4592=EDGE_CURVE ( 'NONE', #16329, #2257, #7793, .T. ) ;
#4595=VERTEX_POINT ( 'NONE', #2874 ) ;
#4597=ORIENTED_EDGE ( 'NONE', *, *, #9264, .F. ) ;
#4599=CARTESIAN_POINT ( 'NONE',  ( -86.00000000000001421, 196.6227766016838245, -24.49489742783178770 ) ) ;
#4601=CARTESIAN_POINT ( 'NONE',  ( 49.99999999999998579, 155.6227766016839098, -12.50000337241049309 ) ) ;
#4602=ADVANCED_FACE ( 'NONE', ( #9769 ), #1378, .T. ) ;
#4605=LINE ( 'NONE', #10076, #10933 ) ;
#4608=FACE_BOUND ( 'NONE', #11129, .T. ) ;
#4611=CARTESIAN_POINT ( 'NONE',  ( 24.87018239537452757, 29.86925179676151032, -6.310755877675157777 ) ) ;
#4612=CARTESIAN_POINT ( 'NONE',  ( 20.85969470496125666, 141.7883037112096929, -14.11015612222007398 ) ) ;
#4618=DIRECTION ( 'NONE',  ( 1.000000000000000000, 0.000000000000000000, -0.000000000000000000 ) ) ;
#4622=ADVANCED_FACE ( 'NONE', ( #4730 ), #5975, .F. ) ;
#4623=CARTESIAN_POINT ( 'NONE',  ( -15.00000000000001421, 90.00000000000000000, -13.00000000000000000 ) ) ;
#4628=DIRECTION ( 'NONE',  ( 0.000000000000000000, 1.000000000000000000, 0.000000000000000000 ) ) ;
#4630=DIRECTION ( 'NONE',  ( -1.000000000000000000, -0.000000000000000000, -0.000000000000000000 ) ) ;
#4632=LINE ( 'NONE', #16499, #16937 ) ;
#4633=DIRECTION ( 'NONE',  ( -0.000000000000000000, -0.000000000000000000, -1.000000000000000000 ) ) ;
#4634=ORIENTED_EDGE ( 'NONE', *, *, #17098, .T. ) ;
#4639=DIRECTION ( 'NONE',  ( 0.000000000000000000, 0.000000000000000000, 1.000000000000000000 ) ) ;
#4640=CARTESIAN_POINT ( 'NONE',  ( -82.50000000000001421, 196.6227766016838245, -16.00000000000000000 ) ) ;
#4641=DIRECTION ( 'NONE',  ( -0.000000000000000000, -0.000000000000000000, 1.000000000000000000 ) ) ;
#4644=CARTESIAN_POINT ( 'NONE',  ( -8.542481054582452771, 30.38359229753140767, -12.94984885967198451 ) ) ;
#4646=CARTESIAN_POINT ( 'NONE',  ( -74.25794599717355027, 198.3976433773785004, -22.54711430683564544 ) ) ;
#4648=ORIENTED_EDGE ( 'NONE', *, *, #2590, .T. ) ;
#4650=FACE_BOUND ( 'NONE', #13800, .T. ) ;
#4651=EDGE_LOOP ( 'NONE', ( #2649, #6486, #79, #3402 ) ) ;
#4652=AXIS2_PLACEMENT_3D ( 'NONE', #17409, #13935, #6610 ) ;
#4654=DIRECTION ( 'NONE',  ( -0.000000000000000000, 1.000000000000000000, -0.000000000000000000 ) ) ;
#4655=ORIENTED_EDGE ( 'NONE', *, *, #17198, .T. ) ;
#4656=ADVANCED_FACE ( 'NONE', ( #15522 ), #15346, .F. ) ;
#4659=CARTESIAN_POINT ( 'NONE',  ( 23.57895800238926043, 142.7196187763571231, -15.94638436093396727 ) ) ;
#4663=CIRCLE ( 'NONE', #17088, 10.00000000000000178 ) ;
#4668=CARTESIAN_POINT ( 'NONE',  ( -20.86241502029082184, 19.99999999999999645, -20.14618526196967352 ) ) ;
#4669=DIRECTION ( 'NONE',  ( -0.000000000000000000, -0.000000000000000000, -1.000000000000000000 ) ) ;
#4672=AXIS2_PLACEMENT_3D ( 'NONE', #5839, #1690, #352 ) ;
#4673=ORIENTED_EDGE ( 'NONE', *, *, #2680, .T. ) ;
#4674=ADVANCED_FACE ( 'NONE', ( #12605 ), #5786, .F. ) ;
#4675=CARTESIAN_POINT ( 'NONE',  ( 27.48361012698968864, 136.6227766016838245, 0.000000000000000000 ) ) ;
#4677=ORIENTED_EDGE ( 'NONE', *, *, #9264, .T. ) ;
#4684=CARTESIAN_POINT ( 'NONE',  ( -16.30611068361787019, 32.76923076923078781, -15.00000000000000000 ) ) ;
#4686=EDGE_LOOP ( 'NONE', ( #6452, #4784, #13062, #15127 ) ) ;
#4687=CARTESIAN_POINT ( 'NONE',  ( 48.00000000000000711, 183.6227766016837961, -8.071800142134975431 ) ) ;
#4691=AXIS2_PLACEMENT_3D ( 'NONE', #12596, #463, #8528 ) ;
#4693=EDGE_LOOP ( 'NONE', ( #13855, #16264, #6802, #17400 ) ) ;
#4695=DIRECTION ( 'NONE',  ( -0.000000000000000000, -0.000000000000000000, 1.000000000000000000 ) ) ;
#4697=EDGE_LOOP ( 'NONE', ( #848, #12301 ) ) ;
#4698=CYLINDRICAL_SURFACE ( 'NONE', #1330, 2.500000000000000444 ) ;
#4699=CARTESIAN_POINT ( 'NONE',  ( 8.904477399773945479, 144.1137579919043787, -18.22932967255391290 ) ) ;
#4701=VERTEX_POINT ( 'NONE', #2410 ) ;
#4705=DIRECTION ( 'NONE',  ( 0.000000000000000000, 0.000000000000000000, 1.000000000000000000 ) ) ;
#4706=DIRECTION ( 'NONE',  ( -0.000000000000000000, -0.000000000000000000, 1.000000000000000000 ) ) ;
#4709=AXIS2_PLACEMENT_3D ( 'NONE', #15230, #11067, #14967 ) ;
#4710=DIRECTION ( 'NONE',  ( -0.000000000000000000, -0.000000000000000000, -1.000000000000000000 ) ) ;
#4713=CARTESIAN_POINT ( 'NONE',  ( 8.602893093599609742, 142.4623620169580818, -19.35743923737696903 ) ) ;
#4714=VECTOR ( 'NONE', #2657, 1000.000000000000000 ) ;
#4717=EDGE_CURVE ( 'NONE', #8095, #6914, #7715, .T. ) ;
#4718=CARTESIAN_POINT ( 'NONE',  ( -27.94760966554430937, 18.00000000000000355, -6.338314452217974626 ) ) ;
#4723=DIRECTION ( 'NONE',  ( -1.000000000000000000, -0.000000000000000000, 0.000000000000000000 ) ) ;
#4729=VECTOR ( 'NONE', #11399, 1000.000000000000000 ) ;
#4730=FACE_OUTER_BOUND ( 'NONE', #10993, .T. ) ;
#4731=CARTESIAN_POINT ( 'NONE',  ( -8.058782516633090864, 30.15486961025272450, -15.00000000000000178 ) ) ;
#4745=ORIENTED_EDGE ( 'NONE', *, *, #13936, .T. ) ;
#4746=ADVANCED_FACE ( 'NONE', ( #3932 ), #6394, .T. ) ;
#4747=AXIS2_PLACEMENT_3D ( 'NONE', #15284, #10041, #3420 ) ;
#4756=AXIS2_PLACEMENT_3D ( 'NONE', #12601, #969, #4639 ) ;
#4762=EDGE_CURVE ( 'NONE', #13399, #14544, #4026, .T. ) ;
#4763=CARTESIAN_POINT ( 'NONE',  ( -13.98869899561406882, 20.00000000000231637, -10.23150106588177621 ) ) ;
#4766=LINE ( 'NONE', #10156, #2266 ) ;
#4770=VECTOR ( 'NONE', #6346, 1000.000000000000000 ) ;
#4774=DIRECTION ( 'NONE',  ( 0.000000000000000000, 0.000000000000000000, 1.000000000000000000 ) ) ;
#4775=CARTESIAN_POINT ( 'NONE',  ( 196.0000000000000000, 163.6227766016838530, -10.00000337241049309 ) ) ;
#4777=DIRECTION ( 'NONE',  ( 0.000000000000000000, 0.000000000000000000, 1.000000000000000000 ) ) ;
#4781=FACE_OUTER_BOUND ( 'NONE', #9942, .T. ) ;
#4782=ADVANCED_FACE ( 'NONE', ( #12320 ), #5689, .F. ) ;
#4784=ORIENTED_EDGE ( 'NONE', *, *, #7869, .F. ) ;
#4785=CARTESIAN_POINT ( 'NONE',  ( 19.96520957614361436, 19.99999999999885603, -13.72477420846906249 ) ) ;
#4786=CARTESIAN_POINT ( 'NONE',  ( -100.0000000000000000, 199.3133755249253056, -1.695560166891042033E-15 ) ) ;
#4789=DIRECTION ( 'NONE',  ( 1.000000000000000000, 0.000000000000000000, 0.000000000000000000 ) ) ;
#4790=ADVANCED_FACE ( 'NONE', ( #2933 ), #5431, .F. ) ;
#4792=AXIS2_PLACEMENT_3D ( 'NONE', #8898, #4588, #14306 ) ;
#4794=AXIS2_PLACEMENT_3D ( 'NONE', #15862, #11522, #3736 ) ;
#4795=DIRECTION ( 'NONE',  ( 0.000000000000000000, 0.000000000000000000, 1.000000000000000000 ) ) ;
#4796=DIRECTION ( 'NONE',  ( 0.000000000000000000, 1.000000000000000000, 0.000000000000000000 ) ) ;
#4797=DIRECTION ( 'NONE',  ( -1.000000000000000000, 0.000000000000000000, 0.000000000000000000 ) ) ;
#4799=CYLINDRICAL_SURFACE ( 'NONE', #4385, 7.500000000000000000 ) ;
#4800=CARTESIAN_POINT ( 'NONE',  ( 31.99336486990593542, 140.9591509882843070, -16.87514788462641491 ) ) ;
#4801=VERTEX_POINT ( 'NONE', #16492 ) ;
#4803=AXIS2_PLACEMENT_3D ( 'NONE', #16132, #10, #16215 ) ;
#4807=DIRECTION ( 'NONE',  ( -1.000000000000000000, 0.000000000000000000, 0.000000000000000000 ) ) ;
#4808=VERTEX_POINT ( 'NONE', #1447 ) ;
#4810=EDGE_CURVE ( 'NONE', #14615, #8170, #10820, .T. ) ;
#4812=VECTOR ( 'NONE', #12642, 1000.000000000000000 ) ;
#4814=VERTEX_POINT ( 'NONE', #12157 ) ;
#4817=CARTESIAN_POINT ( 'NONE',  ( 48.00000000000000711, 167.6227766016838814, -19.42820660268601074 ) ) ;
#4819=CARTESIAN_POINT ( 'NONE',  ( -7.379000772444994638, 30.00000000000000000, -15.00000000000000000 ) ) ;
#4822=FACE_OUTER_BOUND ( 'NONE', #8261, .T. ) ;
#4823=ORIENTED_EDGE ( 'NONE', *, *, #1794, .T. ) ;
#4824=LINE ( 'NONE', #11701, #17191 ) ;
#4825=CARTESIAN_POINT ( 'NONE',  ( -27.81025873171733664, 19.99999999999999289, -7.666431193274479305 ) ) ;
#4826=ORIENTED_EDGE ( 'NONE', *, *, #15766, .F. ) ;
#4827=CARTESIAN_POINT ( 'NONE',  ( 34.82914105512134029, 193.0398713882428012, -27.68487141596273915 ) ) ;
#4828=DIRECTION ( 'NONE',  ( -0.000000000000000000, -0.000000000000000000, -1.000000000000000000 ) ) ;
#4831=ORIENTED_EDGE ( 'NONE', *, *, #7115, .F. ) ;
#4832=ORIENTED_EDGE ( 'NONE', *, *, #1599, .T. ) ;
#4835=CARTESIAN_POINT ( 'NONE',  ( -72.74907522843312790, 148.5867852293671092, -23.63587233142069621 ) ) ;
#4837=CARTESIAN_POINT ( 'NONE',  ( 22.78662571002525183, 144.5042670319084266, -18.82352572523457113 ) ) ;
#4838=DIRECTION ( 'NONE',  ( -0.000000000000000000, -0.000000000000000000, -1.000000000000000000 ) ) ;
#4839=DIRECTION ( 'NONE',  ( 1.000000000000000000, 0.000000000000000000, 0.000000000000000000 ) ) ;
#4840=AXIS2_PLACEMENT_3D ( 'NONE', #16608, #8625, #15008 ) ;
#4841=EDGE_CURVE ( 'NONE', #7936, #2922, #8656, .T. ) ;
#4849=CARTESIAN_POINT ( 'NONE',  ( -14.66060021943728486, 20.00000000000115818, -8.782938007015319570 ) ) ;
#4850=CARTESIAN_POINT ( 'NONE',  ( -74.00000000000001421, 196.6227766016838245, -16.00000000000000000 ) ) ;
#4851=AXIS2_PLACEMENT_3D ( 'NONE', #1640, #12786, #12698 ) ;
#4853=VERTEX_POINT ( 'NONE', #9402 ) ;
#4857=CARTESIAN_POINT ( 'NONE',  ( -147.9615242270661213, 171.6227766016838245, 0.000000000000000000 ) ) ;
#4858=CARTESIAN_POINT ( 'NONE',  ( 10.21857696054809317, 131.9747203951183110, -12.11181647197579636 ) ) ;
#4860=DIRECTION ( 'NONE',  ( 1.000000000000000000, 6.938893903907228378E-16, 0.000000000000000000 ) ) ;
#4861=CARTESIAN_POINT ( 'NONE',  ( -725.0000000000000000, 30.00000000000000000, -15.00000000000000000 ) ) ;
#4863=CARTESIAN_POINT ( 'NONE',  ( 33.47930603387190018, 201.5149201033276825, -18.20725769141082040 ) ) ;
#4866=CARTESIAN_POINT ( 'NONE',  ( 20.25331481973466907, 19.99999999999999289, -13.55662431013403868 ) ) ;
#4869=DIRECTION ( 'NONE',  ( 0.000000000000000000, 0.000000000000000000, -1.000000000000000000 ) ) ;
#4871=VERTEX_POINT ( 'NONE', #4355 ) ;
#4872=FACE_OUTER_BOUND ( 'NONE', #16479, .T. ) ;
#4873=ADVANCED_FACE ( 'NONE', ( #16320 ), #13656, .T. ) ;
#4874=CARTESIAN_POINT ( 'NONE',  ( 48.00000000000000711, 155.6227766016839098, -12.50000337241049309 ) ) ;
#4879=CARTESIAN_POINT ( 'NONE',  ( 36.00000000000002132, 145.8714137932802828, -23.72804097270956447 ) ) ;
#4880=ORIENTED_EDGE ( 'NONE', *, *, #2145, .T. ) ;
#4885=ORIENTED_EDGE ( 'NONE', *, *, #3635, .F. ) ;
#4886=DIRECTION ( 'NONE',  ( 1.000000000000000000, 0.000000000000000000, 0.000000000000000000 ) ) ;
#4889=EDGE_LOOP ( 'NONE', ( #11611, #4010 ) ) ;
#4893=DIRECTION ( 'NONE',  ( -1.000000000000000000, -0.000000000000000000, 0.000000000000000000 ) ) ;
#4894=CARTESIAN_POINT ( 'NONE',  ( -24.81085081034726869, 18.00000000000000000, -15.69149817755460496 ) ) ;
#4895=EDGE_CURVE ( 'NONE', #12240, #8170, #6031, .T. ) ;
#4899=CARTESIAN_POINT ( 'NONE',  ( -11.98734322101357641, 20.00000000000000000, -24.50584837321703802 ) ) ;
#4901=CARTESIAN_POINT ( 'NONE',  ( 30.91081357902854521, 190.6879887351488776, -29.35163774059939712 ) ) ;
#4903=EDGE_LOOP ( 'NONE', ( #1660, #1394, #9400, #7819, #14356, #15989 ) ) ;
#4905=ORIENTED_EDGE ( 'NONE', *, *, #17266, .T. ) ;
#4907=CARTESIAN_POINT ( 'NONE',  ( -72.50000000000002842, 146.9976486552383506, -21.97573418327509742 ) ) ;
#4911=CARTESIAN_POINT ( 'NONE',  ( -40.00000000000000000, 4.000000000000000000, -30.00000000000000711 ) ) ;
#4912=CARTESIAN_POINT ( 'NONE',  ( 35.04302060506833527, 149.8947795965756598, -27.44208088385415678 ) ) ;
#4916=ORIENTED_EDGE ( 'NONE', *, *, #5599, .T. ) ;
#4918=DIRECTION ( 'NONE',  ( -1.000000000000000000, -0.000000000000000000, -0.000000000000000000 ) ) ;
#4919=LINE ( 'NONE', #17133, #6517 ) ;
#4921=ORIENTED_EDGE ( 'NONE', *, *, #10708, .T. ) ;
#4924=EDGE_CURVE ( 'NONE', #8768, #8531, #1837, .T. ) ;
#4928=LINE ( 'NONE', #17324, #14686 ) ;
#4930=VERTEX_POINT ( 'NONE', #15242 ) ;
#4934=CARTESIAN_POINT ( 'NONE',  ( -45.00000000000000000, 140.0000000000000000, 0.000000000000000000 ) ) ;
#4941=AXIS2_PLACEMENT_3D ( 'NONE', #2048, #4706, #7441 ) ;
#4945=CARTESIAN_POINT ( 'NONE',  ( 21.54097706593338302, 29.91227807600463606, -12.53500607440986236 ) ) ;
#4946=CARTESIAN_POINT ( 'NONE',  ( 13.53786153804125725, 141.8544345782132439, -18.40805394434863018 ) ) ;
#4947=EDGE_CURVE ( 'NONE', #6224, #13521, #11716, .T. ) ;
#4948=ADVANCED_FACE ( 'NONE', ( #15142, #8516 ), #7271, .T. ) ;
#4951=CARTESIAN_POINT ( 'NONE',  ( 14.50951369217283826, 138.6207054667691523, -6.378636156063609342 ) ) ;
#4953=CARTESIAN_POINT ( 'NONE',  ( -25.49999999999998579, 10.00000000000000000, -16.00000000000000000 ) ) ;
#4955=AXIS2_PLACEMENT_3D ( 'NONE', #17451, #9299, #4009 ) ;
#4961=CARTESIAN_POINT ( 'NONE',  ( 35.49675130541458401, 144.1922489206527302, -21.74472059540656943 ) ) ;
#4963=FACE_OUTER_BOUND ( 'NONE', #11374, .T. ) ;
#4964=ORIENTED_EDGE ( 'NONE', *, *, #5442, .F. ) ;
#4966=CARTESIAN_POINT ( 'NONE',  ( 14.93242934743711992, 30.00000000000000000, -15.00000000000000000 ) ) ;
#4968=CARTESIAN_POINT ( 'NONE',  ( -14.54670497998689171, 17.99999999999999645, -23.76610458325318831 ) ) ;
#4971=DIRECTION ( 'NONE',  ( -1.000000000000000000, 1.040834085586084059E-15, 0.000000000000000000 ) ) ;
#4978=VECTOR ( 'NONE', #12059, 1000.000000000000000 ) ;
#4979=CARTESIAN_POINT ( 'NONE',  ( 22.50000000000000000, 196.6227766016838245, -21.54065922853802562 ) ) ;
#4980=CARTESIAN_POINT ( 'NONE',  ( 40.00000000000000711, 196.6227766016838245, 0.000000000000000000 ) ) ;
#4981=VECTOR ( 'NONE', #3032, 1000.000000000000000 ) ;
#4982=CARTESIAN_POINT ( 'NONE',  ( -11.84409501751983207, 18.00000000000232703, -9.388895791866135099 ) ) ;
#4983=ORIENTED_EDGE ( 'NONE', *, *, #7249, .T. ) ;
#4984=DIRECTION ( 'NONE',  ( -1.156482317317868274E-16, 1.000000000000000000, 0.000000000000000000 ) ) ;
#4985=EDGE_LOOP ( 'NONE', ( #9864, #1940, #9850 ) ) ;
#4986=EDGE_CURVE ( 'NONE', #10807, #11033, #11152, .T. ) ;
#4987=CARTESIAN_POINT ( 'NONE',  ( 196.0000000000000000, 175.6227766016838245, -5.571800142134975431 ) ) ;
#4990=VERTEX_POINT ( 'NONE', #16834 ) ;
#4994=ADVANCED_FACE ( 'NONE', ( #12676 ), #3381, .F. ) ;
#4997=CARTESIAN_POINT ( 'NONE',  ( -84.24679270737827608, 152.8105824767975491, -27.11332964807919410 ) ) ;
#4998=ADVANCED_FACE ( 'NONE', ( #3729 ), #11603, .F. ) ;
#5000=EDGE_LOOP ( 'NONE', ( #17114, #13613, #15672, #16771, #15755, #7909, #14019 ) ) ;
#5004=CARTESIAN_POINT ( 'NONE',  ( 25.96989122963463004, 151.0873486859325112, -28.34424093584478399 ) ) ;
#5007=VERTEX_POINT ( 'NONE', #17269 ) ;
#5013=ORIENTED_EDGE ( 'NONE', *, *, #15921, .T. ) ;
#5026=CARTESIAN_POINT ( 'NONE',  ( 11.61330907248435018, 130.6704317944142986, -11.35602788888950698 ) ) ;
#5027=EDGE_LOOP ( 'NONE', ( #2867, #17235 ) ) ;
#5031=CARTESIAN_POINT ( 'NONE',  ( -27.99999999999998224, 10.00000000000000000, -30.00000000000000355 ) ) ;
#5033=EDGE_LOOP ( 'NONE', ( #10481, #12932 ) ) ;
#5034=VECTOR ( 'NONE', #997, 1000.000000000000000 ) ;
#5038=CARTESIAN_POINT ( 'NONE',  ( 16.61152767523946139, 141.2200844281568379, -17.35152312112458972 ) ) ;
#5041=CARTESIAN_POINT ( 'NONE',  ( 10.03770976535549586, 140.0890479961802839, -11.85997561143352996 ) ) ;
#5042=ORIENTED_EDGE ( 'NONE', *, *, #12324, .F. ) ;
#5043=DIRECTION ( 'NONE',  ( -1.156482317317868274E-16, 1.000000000000000000, 0.000000000000000000 ) ) ;
#5046=CIRCLE ( 'NONE', #13822, 2.500000000000000000 ) ;
#5052=EDGE_CURVE ( 'NONE', #3299, #7814, #14838, .T. ) ;
#5053=FACE_OUTER_BOUND ( 'NONE', #358, .T. ) ;
#5060=AXIS2_PLACEMENT_3D ( 'NONE', #12138, #6829, #9 ) ;
#5061=CARTESIAN_POINT ( 'NONE',  ( -16.40540729975244716, 18.00000000000000000, -23.03124090058167184 ) ) ;
#5069=FACE_OUTER_BOUND ( 'NONE', #681, .T. ) ;
#5070=CARTESIAN_POINT ( 'NONE',  ( 23.19385591260824597, 193.4380998888852901, -24.76648413410753591 ) ) ;
#5071=CIRCLE ( 'NONE', #10164, 7.500000000000000000 ) ;
#5073=CARTESIAN_POINT ( 'NONE',  ( -12.78422937319141184, 31.72181100014091726, -11.38907491820491913 ) ) ;
#5076=DIRECTION ( 'NONE',  ( -0.000000000000000000, -0.000000000000000000, 1.000000000000000000 ) ) ;
#5078=DIRECTION ( 'NONE',  ( -1.000000000000000000, -0.000000000000000000, 0.000000000000000000 ) ) ;
#5079=CARTESIAN_POINT ( 'NONE',  ( 49.99999999999998579, 167.6227766016838530, -3.071800142134975431 ) ) ;
#5082=ORIENTED_EDGE ( 'NONE', *, *, #12575, .T. ) ;
#5087=VECTOR ( 'NONE', #17327, 1000.000000000000000 ) ;
#5088=ORIENTED_EDGE ( 'NONE', *, *, #114, .T. ) ;
#5094=CARTESIAN_POINT ( 'NONE',  ( 35.90034259984014398, 147.9183216992699386, -25.76577836882855266 ) ) ;
#5097=VERTEX_POINT ( 'NONE', #3549 ) ;
#5101=CARTESIAN_POINT ( 'NONE',  ( 22.87571619445694182, 29.89494019521412582, -11.08657135066705379 ) ) ;
#5102=CARTESIAN_POINT ( 'NONE',  ( 30.49999999999998224, 9.999999999999998224, 1.387778780781445676E-14 ) ) ;
#5103=FACE_OUTER_BOUND ( 'NONE', #3561, .T. ) ;
#5105=CARTESIAN_POINT ( 'NONE',  ( -18.25212770525992667, 32.30769230769230660, -4.999999999999998224 ) ) ;
#5110=EDGE_LOOP ( 'NONE', ( #16478, #16227 ) ) ;
#5112=LINE ( 'NONE', #7750, #13569 ) ;
#5115=FILL_AREA_STYLE_COLOUR ( '', #11215 ) ;
#5119=FACE_OUTER_BOUND ( 'NONE', #5307, .T. ) ;
#5125=CARTESIAN_POINT ( 'NONE',  ( 27.99999999999997513, 4.000000000000000000, -30.00000000000000711 ) ) ;
#5129=CIRCLE ( 'NONE', #16726, 20.00000000000000355 ) ;
#5132=CARTESIAN_POINT ( 'NONE',  ( 6.134011831684059501, 134.2062027339443944, -14.99999999999999822 ) ) ;
#5134=LINE ( 'NONE', #7690, #16326 ) ;
#5135=CARTESIAN_POINT ( 'NONE',  ( 8.856485326996372365, 132.9846638168478137, -12.59946789408625456 ) ) ;
#5136=ORIENTED_EDGE ( 'NONE', *, *, #13166, .F. ) ;
#5140=DIRECTION ( 'NONE',  ( 0.000000000000000000, 1.000000000000000000, 0.000000000000000000 ) ) ;
#5142=LINE ( 'NONE', #11512, #4438 ) ;
#5143=CARTESIAN_POINT ( 'NONE',  ( 34.93420767782698988, 18.00000000000000000, -6.321724734778991106 ) ) ;
#5147=ORIENTED_EDGE ( 'NONE', *, *, #720, .T. ) ;
#5150=CARTESIAN_POINT ( 'NONE',  ( -80.00000000000002842, 146.6227766016838245, -12.99999999999999822 ) ) ;
#5153=DIRECTION ( 'NONE',  ( 0.000000000000000000, 1.000000000000000000, 0.000000000000000000 ) ) ;
#5155=ADVANCED_FACE ( 'NONE', ( #14441 ), #898, .T. ) ;
#5157=EDGE_CURVE ( 'NONE', #152, #10357, #1560, .T. ) ;
#5160=ORIENTED_EDGE ( 'NONE', *, *, #9048, .F. ) ;
#5161=DIRECTION ( 'NONE',  ( 0.000000000000000000, 1.000000000000000000, 0.000000000000000000 ) ) ;
#5164=CARTESIAN_POINT ( 'NONE',  ( -15.09627865792072576, 32.41573384469808161, -9.048329374498470301 ) ) ;
#5165=ORIENTED_EDGE ( 'NONE', *, *, #5384, .F. ) ;
#5166=DIRECTION ( 'NONE',  ( 0.000000000000000000, 0.000000000000000000, 1.000000000000000000 ) ) ;
#5167=ORIENTED_EDGE ( 'NONE', *, *, #987, .F. ) ;
#5168=CARTESIAN_POINT ( 'NONE',  ( 29.78045647795447692, 190.6224931067073669, -29.39406016266897836 ) ) ;
#5169=CARTESIAN_POINT ( 'NONE',  ( -80.00000000000001421, 196.6227766016838245, -13.00000000000000000 ) ) ;
#5170=ORIENTED_EDGE ( 'NONE', *, *, #7736, .F. ) ;
#5172=ORIENTED_EDGE ( 'NONE', *, *, #16829, .F. ) ;
#5174=CARTESIAN_POINT ( 'NONE',  ( -72.52785494716455617, 147.3844239155462503, -22.40167687543583952 ) ) ;
#5175=ORIENTED_EDGE ( 'NONE', *, *, #11335, .T. ) ;
#5178=DIRECTION ( 'NONE',  ( 0.000000000000000000, -1.000000000000000000, 0.000000000000000000 ) ) ;
#5185=CARTESIAN_POINT ( 'NONE',  ( 40.00000000000000711, 171.6227766016838245, 0.000000000000000000 ) ) ;
#5186=CARTESIAN_POINT ( 'NONE',  ( -26.11264420168842904, 19.99999999999999645, -13.35921939055851482 ) ) ;
#5187=ORIENTED_EDGE ( 'NONE', *, *, #7943, .T. ) ;
#5189=EDGE_CURVE ( 'NONE', #14597, #8505, #13718, .T. ) ;
#5190=CARTESIAN_POINT ( 'NONE',  ( 27.99999999999998224, 9.999999999999998224, -35.00000000000000000 ) ) ;
#5192=FACE_OUTER_BOUND ( 'NONE', #4697, .T. ) ;
#5193=DIRECTION ( 'NONE',  ( -1.000000000000000000, 0.000000000000000000, 0.000000000000000000 ) ) ;
#5196=CARTESIAN_POINT ( 'NONE',  ( 30.00000000000001066, 146.6227766016838245, -16.00000000000000000 ) ) ;
#5197=CARTESIAN_POINT ( 'NONE',  ( -79.86026353984452442, 140.6228917578588664, -16.24829651775491257 ) ) ;
#5198=DIRECTION ( 'NONE',  ( 1.000000000000000000, 0.000000000000000000, 0.000000000000000000 ) ) ;
#5200=DIRECTION ( 'NONE',  ( 1.000000000000000000, 0.000000000000000000, 0.000000000000000000 ) ) ;
#5201=FACE_BOUND ( 'NONE', #17199, .T. ) ;
#5202=LINE ( 'NONE', #3891, #8197 ) ;
#5205=ORIENTED_EDGE ( 'NONE', *, *, #114, .F. ) ;
#5207=ORIENTED_EDGE ( 'NONE', *, *, #13621, .T. ) ;
#5210=AXIS2_PLACEMENT_3D ( 'NONE', #11782, #4093, #5153 ) ;
#5211=ORIENTED_EDGE ( 'NONE', *, *, #11134, .T. ) ;
#5212=FACE_OUTER_BOUND ( 'NONE', #4889, .T. ) ;
#5213=CARTESIAN_POINT ( 'NONE',  ( 13.82444641086477866, 138.9325364249946517, -8.217559156359119044 ) ) ;
#5217=EDGE_CURVE ( 'NONE', #6709, #12804, #718, .T. ) ;
#5218=EDGE_CURVE ( 'NONE', #13962, #11970, #9832, .T. ) ;
#5219=LINE ( 'NONE', #9454, #15210 ) ;
#5220=LINE ( 'NONE', #10617, #1605 ) ;
#5223=CARTESIAN_POINT ( 'NONE',  ( 18.26135686777330136, 17.99999999999999289, -12.35203162874035065 ) ) ;
#5224=DIRECTION ( 'NONE',  ( 0.000000000000000000, 1.387778780781445676E-14, 1.000000000000000000 ) ) ;
#5225=DIRECTION ( 'NONE',  ( 0.000000000000000000, 0.000000000000000000, -1.000000000000000000 ) ) ;
#5227=CYLINDRICAL_SURFACE ( 'NONE', #3807, 10.00000000000000178 ) ;
#5229=ORIENTED_EDGE ( 'NONE', *, *, #16538, .T. ) ;
#5230=DIRECTION ( 'NONE',  ( 1.000000000000000000, 0.000000000000000000, -0.000000000000000000 ) ) ;
#5233=DIRECTION ( 'NONE',  ( 0.000000000000000000, 1.000000000000000000, 0.000000000000000000 ) ) ;
#5235=ORIENTED_EDGE ( 'NONE', *, *, #9481, .T. ) ;
#5238=ORIENTED_EDGE ( 'NONE', *, *, #6965, .F. ) ;
#5240=AXIS2_PLACEMENT_3D ( 'NONE', #17163, #4695, #8646 ) ;
#5241=VECTOR ( 'NONE', #10795, 1000.000000000000000 ) ;
#5243=CARTESIAN_POINT ( 'NONE',  ( 31.13499951972123014, 189.1866491494220384, -27.93804624201380804 ) ) ;
#5244=CARTESIAN_POINT ( 'NONE',  ( 17.56962100350864375, 125.3109322897003608, -3.333333333333324600 ) ) ;
#5245=CARTESIAN_POINT ( 'NONE',  ( -12.76199592490470636, 18.00000000000464340, -6.193401609026034649 ) ) ;
#5250=AXIS2_PLACEMENT_3D ( 'NONE', #10498, #4052, #1295 ) ;
#5252=CARTESIAN_POINT ( 'NONE',  ( -81.45415618582130435, 189.2596037578064454, -27.89172594985640430 ) ) ;
#5256=VERTEX_POINT ( 'NONE', #2554 ) ;
#5257=ORIENTED_EDGE ( 'NONE', *, *, #4986, .T. ) ;
#5258=CARTESIAN_POINT ( 'NONE',  ( 27.48361012698979522, 126.6227766016837819, -6.072704737864100906E-13 ) ) ;
#5260=VECTOR ( 'NONE', #11788, 1000.000000000000000 ) ;
#5261=ORIENTED_EDGE ( 'NONE', *, *, #4841, .T. ) ;
#5265=CARTESIAN_POINT ( 'NONE',  ( 24.00000000000000355, 146.9394831494156790, -24.81813469455734378 ) ) ;
#5267=DIRECTION ( 'NONE',  ( -1.000000000000000000, -0.000000000000000000, -0.000000000000000000 ) ) ;
#5270=CARTESIAN_POINT ( 'NONE',  ( 24.93507336697353338, 29.86842105263157521, -5.660390792616599498 ) ) ;
#5272=ADVANCED_FACE ( 'NONE', ( #5387 ), #10944, .F. ) ;
#5273=CARTESIAN_POINT ( 'NONE',  ( 15.00000000000903455, 143.2058235767352983, -16.77804593520375676 ) ) ;
#5274=EDGE_CURVE ( 'NONE', #1367, #12793, #7222, .T. ) ;
#5275=PLANE ( 'NONE',  #7752 ) ;
#5277=EDGE_CURVE ( 'NONE', #10995, #11591, #15192, .T. ) ;
#5278=ORIENTED_EDGE ( 'NONE', *, *, #6382, .F. ) ;
#5279=CARTESIAN_POINT ( 'NONE',  ( -85.27494917608791525, 141.2912748254776147, -13.00000000000000000 ) ) ;
#5280=AXIS2_PLACEMENT_3D ( 'NONE', #1776, #1863, #3456 ) ;
#5281=AXIS2_PLACEMENT_3D ( 'NONE', #13290, #11448, #2483 ) ;
#5283=VECTOR ( 'NONE', #9283, 1000.000000000000000 ) ;
#5285=DIRECTION ( 'NONE',  ( 1.156482317317868274E-16, -1.000000000000000000, 0.000000000000000000 ) ) ;
#5286=APPLICATION_CONTEXT ( 'automotive_design' ) ;
#5290=CARTESIAN_POINT ( 'NONE',  ( -100.0000000000000000, 144.1839557653416080, -18.33333333333335702 ) ) ;
#5291=CARTESIAN_POINT ( 'NONE',  ( 16.61976933981454962, 29.96600215813370838, -12.82127072618890118 ) ) ;
#5292=CARTESIAN_POINT ( 'NONE',  ( -48.00000000000000000, 154.3022685259950038, -9.999999999999900524 ) ) ;
#5297=ORIENTED_EDGE ( 'NONE', *, *, #2145, .F. ) ;
#5298=DIRECTION ( 'NONE',  ( 0.000000000000000000, 0.000000000000000000, 1.000000000000000000 ) ) ;
#5303=PRODUCT_DEFINITION_CONTEXT ( 'detailed design', #5286, 'design' ) ;
#5304=ORIENTED_EDGE ( 'NONE', *, *, #15386, .T. ) ;
#5307=EDGE_LOOP ( 'NONE', ( #16447, #15426, #9108, #10380, #617, #10194, #13742, #17512, #16882, #10842, #6434, #15902 ) ) ;
#5308=CARTESIAN_POINT ( 'NONE',  ( -83.53742222559971253, 151.4735692324751994, -28.61877689333859109 ) ) ;
#5310=CARTESIAN_POINT ( 'NONE',  ( 14.28882419134376747, 138.6263508161794675, -3.987386623658401241 ) ) ;
#5320=CARTESIAN_POINT ( 'NONE',  ( 19.87492423018547427, 17.99999999999543121, -11.43634947295695703 ) ) ;
#5325=AXIS2_PLACEMENT_3D ( 'NONE', #1680, #2913, #8570 ) ;
#5331=EDGE_CURVE ( 'NONE', #12122, #15415, #150, .T. ) ;
#5335=CARTESIAN_POINT ( 'NONE',  ( -125.0000000000000000, 206.6227766016838245, 0.000000000000000000 ) ) ;
#5337=DIRECTION ( 'NONE',  ( 0.000000000000000000, 0.000000000000000000, 1.000000000000000000 ) ) ;
#5341=CARTESIAN_POINT ( 'NONE',  ( 36.97967542706143718, 193.8447098639589967, -24.40281628369250555 ) ) ;
#5342=DIRECTION ( 'NONE',  ( 1.000000000000000000, 0.000000000000000000, -0.000000000000000000 ) ) ;
#5343=PLANE ( 'NONE',  #8037 ) ;
#5350=CARTESIAN_POINT ( 'NONE',  ( -87.50000000000004263, 196.2479045481292985, -21.97573418327510808 ) ) ;
#5352=CARTESIAN_POINT ( 'NONE',  ( -90.80384757729339640, 138.6227766016838245, 0.000000000000000000 ) ) ;
#5353=EDGE_CURVE ( 'NONE', #11033, #11867, #329, .T. ) ;
#5354=VERTEX_POINT ( 'NONE', #12460 ) ;
#5357=B_SPLINE_CURVE_WITH_KNOTS ( 'NONE', 3,
 ( #7171, #7514, #16824, #437, #15491, #4531, #14178, #16660, #804, #9916, #2039, #1950, #16747, #8679, #4612, #538, #14089, #7353, #12834, #7433 ),
 .UNSPECIFIED., .F., .F.,
 ( 4, 2, 2, 2, 2, 2, 2, 2, 2, 4 ),
 ( 0.000000000000000000, 0.002318945972243265704, 0.003478418958364892268, 0.004637891944486519265, 0.006956837916729771525, 0.009275783888973026386, 0.01159472986121627865, 0.01391367583345953091, 0.01623262180570278490, 0.01855156777794603890 ),
 .UNSPECIFIED. ) ;
#5360=ORIENTED_EDGE ( 'NONE', *, *, #5423, .F. ) ;
#5364=AXIS2_PLACEMENT_3D ( 'NONE', #7899, #8158, #11784 ) ;
#5365=FACE_OUTER_BOUND ( 'NONE', #752, .T. ) ;
#5366=CARTESIAN_POINT ( 'NONE',  ( -90.80384757729339640, 138.6227766016838245, 0.000000000000000000 ) ) ;
#5367=FACE_BOUND ( 'NONE', #14169, .T. ) ;
#5372=CARTESIAN_POINT ( 'NONE',  ( 49.99999999999998579, 163.6227766016838530, -12.50000337241049309 ) ) ;
#5373=FACE_OUTER_BOUND ( 'NONE', #5961, .T. ) ;
#5379=ORIENTED_EDGE ( 'NONE', *, *, #11054, .T. ) ;
#5382=EDGE_CURVE ( 'NONE', #11298, #9392, #6365, .T. ) ;
#5384=EDGE_CURVE ( 'NONE', #11068, #15082, #11463, .T. ) ;
#5385=CARTESIAN_POINT ( 'NONE',  ( 15.56337975240373872, 125.2134999403456135, -4.999999999999997335 ) ) ;
#5387=FACE_OUTER_BOUND ( 'NONE', #3496, .T. ) ;
#5388=VECTOR ( 'NONE', #5285, 1000.000000000000000 ) ;
#5389=DIRECTION ( 'NONE',  ( 0.000000000000000000, -0.8660254037844413721, -0.4999999999999953371 ) ) ;
#5394=CYLINDRICAL_SURFACE ( 'NONE', #13214, 2.500000000000000444 ) ;
#5399=CARTESIAN_POINT ( 'NONE',  ( 16.12877328687227774, 136.8349817083154676, -4.209125965272636272 ) ) ;
#5400=ORIENTED_EDGE ( 'NONE', *, *, #8514, .F. ) ;
#5402=VECTOR ( 'NONE', #7384, 1000.000000000000000 ) ;
#5403=DIRECTION ( 'NONE',  ( -1.000000000000000000, 0.000000000000000000, 0.000000000000000000 ) ) ;
#5408=CARTESIAN_POINT ( 'NONE',  ( 23.34636706823183872, 200.1176944260899120, -16.66575456205188743 ) ) ;
#5411=CARTESIAN_POINT ( 'NONE',  ( 18.93266870823487125, 29.92002005853035840, -11.93384102663519997 ) ) ;
#5412=CARTESIAN_POINT ( 'NONE',  ( -22.99999999999999289, 100.0000000000000142, 0.000000000000000000 ) ) ;
#5413=CIRCLE ( 'NONE', #4568, 5.999999999999998224 ) ;
#5415=CARTESIAN_POINT ( 'NONE',  ( -50.00000000000000000, 154.3022685259950038, -9.999999999999900524 ) ) ;
#5416=CARTESIAN_POINT ( 'NONE',  ( 27.59653005489939659, 141.1206502181308338, -17.16533225383574290 ) ) ;
#5418=CARTESIAN_POINT ( 'NONE',  ( 8.750829511962136209, 133.4309389808502715, -14.69696305399116198 ) ) ;
#5419=ORIENTED_EDGE ( 'NONE', *, *, #10825, .T. ) ;
#5423=EDGE_CURVE ( 'NONE', #7078, #12240, #12979, .T. ) ;
#5429=ORIENTED_EDGE ( 'NONE', *, *, #12280, .T. ) ;
#5431=PLANE ( 'NONE',  #10027 ) ;
#5432=DIRECTION ( 'NONE',  ( -1.000000000000000000, -0.000000000000000000, 0.000000000000000000 ) ) ;
#5437=CARTESIAN_POINT ( 'NONE',  ( -79.43652167955697507, 189.1215240515805931, -27.97845313684487678 ) ) ;
#5438=LINE ( 'NONE', #11086, #7247 ) ;
#5439=ORIENTED_EDGE ( 'NONE', *, *, #15638, .F. ) ;
#5440=VERTEX_POINT ( 'NONE', #6072 ) ;
#5442=EDGE_CURVE ( 'NONE', #2002, #5792, #12890, .T. ) ;
#5444=B_SPLINE_CURVE_WITH_KNOTS ( 'NONE', 3,
 ( #1116, #5270, #3688, #16084, #7931, #15982, #14753, #1291, #10673, #11722, #5101, #14661, #15898, #16177, #6604, #940, #3961, #9346, #2348, #2625, #9075, #7662, #13337, #13151, #11817 ),
 .UNSPECIFIED., .F., .F.,
 ( 4, 2, 2, 2, 2, 2, 2, 2, 2, 1, 2, 2, 4 ),
 ( 0.000000000000000000, 0.001953037758357041142, 0.002929556637535561930, 0.003906075516714082284, 0.005859113275071132533, 0.006835632154249659392, 0.007812151033428187119, 0.009765188791785242572, 0.01074170767096376509, 0.01171822655014228762, 0.01269474542932080841, 0.01367126430849933093, 0.01562430206685638465 ),
 .UNSPECIFIED. ) ;
#5447=CARTESIAN_POINT ( 'NONE',  ( -30.49999999999998224, 10.00000000000000000, 1.387778780781445676E-14 ) ) ;
#5449=CARTESIAN_POINT ( 'NONE',  ( -27.99999999999998224, 10.00000000000000000, -35.00200000000000244 ) ) ;
#5452=DIRECTION ( 'NONE',  ( 1.000000000000000000, 0.000000000000000000, 0.000000000000000000 ) ) ;
#5454=ORIENTED_EDGE ( 'NONE', *, *, #7249, .F. ) ;
#5455=CARTESIAN_POINT ( 'NONE',  ( -79.06135944198280185, 202.5503328113395298, -16.38559373769483685 ) ) ;
#5457=DIRECTION ( 'NONE',  ( 0.000000000000000000, 0.000000000000000000, -1.000000000000000000 ) ) ;
#5458=DIRECTION ( 'NONE',  ( 1.000000000000000000, 0.000000000000000000, 0.000000000000000000 ) ) ;
#5460=EDGE_CURVE ( 'NONE', #1799, #7907, #8890, .T. ) ;
#5462=ORIENTED_EDGE ( 'NONE', *, *, #10405, .F. ) ;
#5465=CARTESIAN_POINT ( 'NONE',  ( 27.48361012695778882, 136.6227766016838530, -1.300194169143111589 ) ) ;
#5466=CARTESIAN_POINT ( 'NONE',  ( 49.99999999999998579, 179.6227766016838245, -12.50000337241049309 ) ) ;
#5470=CARTESIAN_POINT ( 'NONE',  ( 40.00000000000000711, 146.6227766016838245, 0.000000000000000000 ) ) ;
#5471=CARTESIAN_POINT ( 'NONE',  ( -27.99999999999998224, 10.00000000000000000, -12.99999999999999822 ) ) ;
#5475=EDGE_CURVE ( 'NONE', #7915, #14615, #17044, .T. ) ;
#5476=EDGE_CURVE ( 'NONE', #3210, #7898, #931, .T. ) ;
#5477=CARTESIAN_POINT ( 'NONE',  ( 16.36928288456664049, 136.8619714623083610, -5.700917076122243188 ) ) ;
#5479=CARTESIAN_POINT ( 'NONE',  ( -74.09965740015987024, 147.9183216992699101, -25.76577836882853489 ) ) ;
#5482=CARTESIAN_POINT ( 'NONE',  ( 0.000000000000000000, 0.000000000000000000, 0.000000000000000000 ) ) ;
#5485=FACE_OUTER_BOUND ( 'NONE', #13933, .T. ) ;
#5487=CARTESIAN_POINT ( 'NONE',  ( 33.66231827095856488, 18.00000000000000000, -12.04861179558545636 ) ) ;
#5488=CARTESIAN_POINT ( 'NONE',  ( 20.77386775082738879, 29.88392224133981401, -10.47448535043027462 ) ) ;
#5489=DIRECTION ( 'NONE',  ( 0.000000000000000000, 0.000000000000000000, 1.000000000000000000 ) ) ;
#5495=CARTESIAN_POINT ( 'NONE',  ( 9.788850454972870097, 132.9181049171561995, -14.40474131580982231 ) ) ;
#5496=EDGE_CURVE ( 'NONE', #6195, #13094, #15975, .T. ) ;
#5498=AXIS2_PLACEMENT_3D ( 'NONE', #8953, #10011, #4971 ) ;
#5502=ORIENTED_EDGE ( 'NONE', *, *, #7865, .T. ) ;
#5504=DIRECTION ( 'NONE',  ( 0.000000000000000000, 1.000000000000000000, 0.000000000000000000 ) ) ;
#5506=CARTESIAN_POINT ( 'NONE',  ( 37.50000000000000000, 146.9976486552383790, -21.97573418327510097 ) ) ;
#5509=CARTESIAN_POINT ( 'NONE',  ( -80.00000000000001421, 196.6227766016838245, -12.99999999999999822 ) ) ;
#5511=DIRECTION ( 'NONE',  ( -0.000000000000000000, -0.000000000000000000, 1.000000000000000000 ) ) ;
#5512=VERTEX_POINT ( 'NONE', #7923 ) ;
#5513=FACE_BOUND ( 'NONE', #3372, .T. ) ;
#5514=EDGE_CURVE ( 'NONE', #588, #9872, #17408, .T. ) ;
#5518=ORIENTED_EDGE ( 'NONE', *, *, #3635, .T. ) ;
#5519=CARTESIAN_POINT ( 'NONE',  ( -85.93543503013836471, 192.0313071030111871, -25.93356563065114528 ) ) ;
#5521=CARTESIAN_POINT ( 'NONE',  ( -15.27350142870561811, 32.46802521863179436, -8.792838265516087048 ) ) ;
#5522=ORIENTED_EDGE ( 'NONE', *, *, #3593, .T. ) ;
#5525=DIRECTION ( 'NONE',  ( 0.000000000000000000, 0.000000000000000000, 1.000000000000000000 ) ) ;
#5527=EDGE_LOOP ( 'NONE', ( #12945, #1451, #5502, #15102 ) ) ;
#5530=DIRECTION ( 'NONE',  ( 1.000000000000000000, 0.000000000000000000, 0.000000000000000000 ) ) ;
#5531=CARTESIAN_POINT ( 'NONE',  ( 22.93524650466161674, 29.84210526315774104, -5.528366322421692125 ) ) ;
#5532=DIRECTION ( 'NONE',  ( -1.000000000000000000, -0.000000000000000000, -0.000000000000000000 ) ) ;
#5533=LINE ( 'NONE', #4213, #6933 ) ;
#5536=VECTOR ( 'NONE', #5267, 1000.000000000000000 ) ;
#5538=CARTESIAN_POINT ( 'NONE',  ( -82.39581698594608383, 202.1282835878849369, -17.15932559113869971 ) ) ;
#5539=CARTESIAN_POINT ( 'NONE',  ( 196.0000000000000000, 163.6227766016838530, -12.50000337241049309 ) ) ;
#5542=DIRECTION ( 'NONE',  ( -1.000000000000000000, 0.000000000000000000, 0.000000000000000000 ) ) ;
#5544=EDGE_CURVE ( 'NONE', #16407, #6443, #5711, .T. ) ;
#5548=VECTOR ( 'NONE', #12877, 1000.000000000000000 ) ;
#5549=ORIENTED_EDGE ( 'NONE', *, *, #8124, .F. ) ;
#5550=DIRECTION ( 'NONE',  ( 0.000000000000000000, 0.000000000000000000, 1.000000000000000000 ) ) ;
#5552=ORIENTED_EDGE ( 'NONE', *, *, #5722, .F. ) ;
#5553=CARTESIAN_POINT ( 'NONE',  ( 27.44407568426047206, 136.8394969516870958, -3.888888888888889728 ) ) ;
#5554=DIRECTION ( 'NONE',  ( 1.000000000000000000, 0.000000000000000000, 0.000000000000000000 ) ) ;
#5556=AXIS2_PLACEMENT_3D ( 'NONE', #16936, #6043, #7282 ) ;
#5558=ORIENTED_EDGE ( 'NONE', *, *, #6612, .F. ) ;
#5565=CARTESIAN_POINT ( 'NONE',  ( 16.31902522550215551, 136.8400131045044930, -5.103539400524613967 ) ) ;
#5566=ORIENTED_EDGE ( 'NONE', *, *, #10985, .F. ) ;
#5567=CARTESIAN_POINT ( 'NONE',  ( -85.00000000000002842, 146.6227766016838245, -12.99999999999999822 ) ) ;
#5568=DIRECTION ( 'NONE',  ( 1.000000000000000000, 0.000000000000000000, 0.000000000000000000 ) ) ;
#5572=VECTOR ( 'NONE', #16948, 1000.000000000000000 ) ;
#5573=CARTESIAN_POINT ( 'NONE',  ( -77.00170055202453057, 191.4074798671404949, -28.87243506922800051 ) ) ;
#5575=ADVANCED_FACE ( 'NONE', ( #5365 ), #11097, .T. ) ;
#5577=CARTESIAN_POINT ( 'NONE',  ( 30.81698523721487604, 18.00000000000000000, -17.17210857557096659 ) ) ;
#5578=CARTESIAN_POINT ( 'NONE',  ( -48.00000000000000000, 171.6227766016838245, 0.000000000000000000 ) ) ;
#5580=CARTESIAN_POINT ( 'NONE',  ( -7.379000772444994638, 30.00000000000000000, -25.00000000000000000 ) ) ;
#5584=VECTOR ( 'NONE', #5200, 1000.000000000000000 ) ;
#5588=CARTESIAN_POINT ( 'NONE',  ( 22.50000000000001421, 146.6227766016838245, -21.54065922853802562 ) ) ;
#5589=VERTEX_POINT ( 'NONE', #16437 ) ;
#5594=DIRECTION ( 'NONE',  ( 0.000000000000000000, 0.000000000000000000, 1.000000000000000000 ) ) ;
#5595=VERTEX_POINT ( 'NONE', #14913 ) ;
#5599=EDGE_CURVE ( 'NONE', #7553, #4527, #16510, .T. ) ;
#5603=DIRECTION ( 'NONE',  ( -1.000000000000000000, -0.000000000000000000, 0.000000000000000000 ) ) ;
#5605=ORIENTED_EDGE ( 'NONE', *, *, #17288, .T. ) ;
#5607=ORIENTED_EDGE ( 'NONE', *, *, #14249, .T. ) ;
#5608=DIRECTION ( 'NONE',  ( 1.000000000000000000, 0.000000000000000000, 0.000000000000000000 ) ) ;
#5610=CARTESIAN_POINT ( 'NONE',  ( -85.45105639388464169, 191.4650750923992177, -26.36917907415269724 ) ) ;
#5611=CARTESIAN_POINT ( 'NONE',  ( -100.0000000000000000, 144.1839557653416080, -18.33333333333335702 ) ) ;
#5612=CARTESIAN_POINT ( 'NONE',  ( -16.30611068361787019, 32.76923076923078781, -4.999999999999999112 ) ) ;
#5613=TOROIDAL_SURFACE ( 'NONE', #1092, 240.0000000000000000, 10.00000000000000000 ) ;
#5615=EDGE_LOOP ( 'NONE', ( #2741, #626, #3331, #6297 ) ) ;
#5616=DIRECTION ( 'NONE',  ( -1.000000000000000000, -0.000000000000000000, 0.000000000000000000 ) ) ;
#5619=CARTESIAN_POINT ( 'NONE',  ( 30.00000000000000355, 196.6227766016838245, -16.00000000000000000 ) ) ;
#5620=ORIENTED_EDGE ( 'NONE', *, *, #8168, .F. ) ;
#5622=CARTESIAN_POINT ( 'NONE',  ( -45.00000000000000000, 134.2062027339443944, -25.00000000000000000 ) ) ;
#5630=CARTESIAN_POINT ( 'NONE',  ( -81.40404063475818930, 202.4574374834314483, -16.55982638047048638 ) ) ;
#5633=PLANE ( 'NONE',  #1671 ) ;
#5637=CYLINDRICAL_SURFACE ( 'NONE', #568, 5.999999999999998224 ) ;
#5639=EDGE_LOOP ( 'NONE', ( #4826, #8904 ) ) ;
#5640=EDGE_CURVE ( 'NONE', #15415, #8582, #10057, .T. ) ;
#5646=CARTESIAN_POINT ( 'NONE',  ( 27.99999999999998224, 9.999999999999998224, -30.00000000000001066 ) ) ;
#5650=AXIS2_PLACEMENT_3D ( 'NONE', #5819, #1491, #8292 ) ;
#5653=AXIS2_PLACEMENT_3D ( 'NONE', #1210, #6532, #14317 ) ;
#5654=DIRECTION ( 'NONE',  ( 1.000000000000000000, 0.000000000000000000, -8.673617379884036705E-17 ) ) ;
#5656=ADVANCED_FACE ( 'NONE', ( #9677 ), #16169, .F. ) ;
#5659=CIRCLE ( 'NONE', #16703, 10.00000000000000000 ) ;
#5660=CIRCLE ( 'NONE', #11028, 20.00000000000000355 ) ;
#5663=CARTESIAN_POINT ( 'NONE',  ( -81.56512917543578567, 190.8261496651129221, -29.26147795858665646 ) ) ;
#5668=ADVANCED_FACE ( 'NONE', ( #48 ), #15078, .T. ) ;
#5670=ADVANCED_FACE ( 'NONE', ( #4210 ), #14999, .T. ) ;
#5671=DIRECTION ( 'NONE',  ( 1.000000000000000000, 0.000000000000000000, -0.000000000000000000 ) ) ;
#5673=DIRECTION ( 'NONE',  ( 0.000000000000000000, 0.000000000000000000, 1.000000000000000000 ) ) ;
#5677=CARTESIAN_POINT ( 'NONE',  ( 23.92105171931311958, 29.88144160311327724, -9.435928464502936208 ) ) ;
#5680=ADVANCED_FACE ( 'NONE', ( #15345 ), #16855, .F. ) ;
#5683=DIRECTION ( 'NONE',  ( 1.000000000000000000, 0.000000000000000000, -0.000000000000000000 ) ) ;
#5685=CARTESIAN_POINT ( 'NONE',  ( 37.34717144291667523, 148.1823054118432026, -23.23525722188765741 ) ) ;
#5686=AXIS2_PLACEMENT_3D ( 'NONE', #8874, #14617, #13296 ) ;
#5688=CARTESIAN_POINT ( 'NONE',  ( -27.99999999999998224, 10.00000000000000000, -12.99999999999999822 ) ) ;
#5689=PLANE ( 'NONE',  #4229 ) ;
#5692=CARTESIAN_POINT ( 'NONE',  ( 48.00000000000000711, 163.6227766016838530, -15.00000337241049486 ) ) ;
#5694=DIRECTION ( 'NONE',  ( 0.000000000000000000, 0.000000000000000000, -1.000000000000000000 ) ) ;
#5695=ORIENTED_EDGE ( 'NONE', *, *, #14451, .T. ) ;
#5702=VERTEX_POINT ( 'NONE', #5785 ) ;
#5703=EDGE_CURVE ( 'NONE', #1561, #3210, #1309, .T. ) ;
#5704=EDGE_LOOP ( 'NONE', ( #11413, #4360, #17033, #8237 ) ) ;
#5705=FACE_OUTER_BOUND ( 'NONE', #2355, .T. ) ;
#5708=ORIENTED_EDGE ( 'NONE', *, *, #10104, .F. ) ;
#5711=LINE ( 'NONE', #220, #15687 ) ;
#5712=DIRECTION ( 'NONE',  ( 1.000000000000000000, 0.000000000000000000, 0.000000000000000000 ) ) ;
#5718=CARTESIAN_POINT ( 'NONE',  ( 20.13757169487763576, 19.99999999999999289, -24.32197800972832624 ) ) ;
#5720=FACE_OUTER_BOUND ( 'NONE', #6858, .T. ) ;
#5721=VERTEX_POINT ( 'NONE', #3139 ) ;
#5722=EDGE_CURVE ( 'NONE', #12617, #10091, #16288, .T. ) ;
#5723=EDGE_LOOP ( 'NONE', ( #13097, #15044, #12927, #8614 ) ) ;
#5727=ORIENTED_EDGE ( 'NONE', *, *, #13749, .F. ) ;
#5728=FACE_OUTER_BOUND ( 'NONE', #3600, .T. ) ;
#5731=DIRECTION ( 'NONE',  ( -0.000000000000000000, -0.000000000000000000, -1.000000000000000000 ) ) ;
#5732=DIRECTION ( 'NONE',  ( 0.000000000000000000, 1.734723475976807094E-15, -1.000000000000000000 ) ) ;
#5733=EDGE_LOOP ( 'NONE', ( #7559, #1532, #5982, #2673 ) ) ;
#5737=EDGE_CURVE ( 'NONE', #12705, #1250, #4559, .T. ) ;
#5738=DIRECTION ( 'NONE',  ( -1.000000000000000000, -0.000000000000000000, -0.000000000000000000 ) ) ;
#5740=CARTESIAN_POINT ( 'NONE',  ( 26.13287303778632165, 137.8093815885048627, -9.050576676228219597 ) ) ;
#5744=VERTEX_POINT ( 'NONE', #8711 ) ;
#5745=DIRECTION ( 'NONE',  ( 0.000000000000000000, 0.000000000000000000, 1.000000000000000000 ) ) ;
#5750=CARTESIAN_POINT ( 'NONE',  ( -30.49999999999998224, 10.00000000000000000, -16.00000000000000000 ) ) ;
#5752=EDGE_CURVE ( 'NONE', #9797, #9988, #384, .T. ) ;
#5753=CARTESIAN_POINT ( 'NONE',  ( -24.99999999999999289, 100.0000000000000142, 0.000000000000000000 ) ) ;
#5754=ORIENTED_EDGE ( 'NONE', *, *, #3930, .F. ) ;
#5758=EDGE_LOOP ( 'NONE', ( #6654, #7465, #13604, #14997 ) ) ;
#5764=CARTESIAN_POINT ( 'NONE',  ( 24.54484354042847016, 151.7936747764227619, -26.38258506112509494 ) ) ;
#5765=FACE_OUTER_BOUND ( 'NONE', #70, .T. ) ;
#5766=CARTESIAN_POINT ( 'NONE',  ( 0.000000000000000000, 18.00000000000000355, 0.000000000000000000 ) ) ;
#5767=AXIS2_PLACEMENT_3D ( 'NONE', #12788, #1991, #9862 ) ;
#5770=CARTESIAN_POINT ( 'NONE',  ( 34.93420767853316988, 18.00000000000000355, -4.999999999999999112 ) ) ;
#5772=ORIENTED_EDGE ( 'NONE', *, *, #1485, .F. ) ;
#5776=ORIENTED_EDGE ( 'NONE', *, *, #1656, .F. ) ;
#5778=ORIENTED_EDGE ( 'NONE', *, *, #2820, .F. ) ;
#5779=CARTESIAN_POINT ( 'NONE',  ( 37.99999999999999289, 20.00000000000000000, 0.000000000000000000 ) ) ;
#5784=CARTESIAN_POINT ( 'NONE',  ( 40.00000000000000711, 146.6227766016838245, 0.000000000000000000 ) ) ;
#5785=CARTESIAN_POINT ( 'NONE',  ( 37.50000000000000711, 196.6227766016838245, -13.00000000000000000 ) ) ;
#5786=CYLINDRICAL_SURFACE ( 'NONE', #7043, 8.000000000000000000 ) ;
#5788=EDGE_CURVE ( 'NONE', #16962, #243, #10902, .T. ) ;
#5790=CYLINDRICAL_SURFACE ( 'NONE', #398, 7.499999999999996447 ) ;
#5791=AXIS2_PLACEMENT_3D ( 'NONE', #16411, #4277, #9658 ) ;
#5792=VERTEX_POINT ( 'NONE', #4640 ) ;
#5793=CARTESIAN_POINT ( 'NONE',  ( -80.00000000000001421, 196.6227766016838245, 1.387778780781445676E-14 ) ) ;
#5795=DIRECTION ( 'NONE',  ( -1.000000000000000000, -0.000000000000000000, -0.000000000000000000 ) ) ;
#5796=CARTESIAN_POINT ( 'NONE',  ( 30.81698523721487604, 20.00000000000000355, -17.17210857557096659 ) ) ;
#5798=FACE_BOUND ( 'NONE', #15520, .T. ) ;
#5802=ORIENTED_EDGE ( 'NONE', *, *, #240, .F. ) ;
#5803=DIRECTION ( 'NONE',  ( -1.000000000000000000, 0.000000000000000000, 0.000000000000000000 ) ) ;
#5804=AXIS2_PLACEMENT_3D ( 'NONE', #16366, #11036, #15020 ) ;
#5805=ORIENTED_EDGE ( 'NONE', *, *, #12510, .F. ) ;
#5809=CARTESIAN_POINT ( 'NONE',  ( 196.0000000000000000, 167.6227766016838530, -3.071800142134975431 ) ) ;
#5810=VECTOR ( 'NONE', #3690, 1000.000000000000000 ) ;
#5816=CARTESIAN_POINT ( 'NONE',  ( 24.93034343272520204, 18.00000000000000000, -22.33460256651928333 ) ) ;
#5819=CARTESIAN_POINT ( 'NONE',  ( 15.00000000000000000, 171.6227766016838245, 0.000000000000000000 ) ) ;
#5821=CARTESIAN_POINT ( 'NONE',  ( -40.00000000000000000, 0.000000000000000000, -30.00000000000000355 ) ) ;
#5822=AXIS2_PLACEMENT_3D ( 'NONE', #15264, #16691, #3220 ) ;
#5824=DIRECTION ( 'NONE',  ( 1.000000000000000000, 0.000000000000000000, -0.000000000000000000 ) ) ;
#5826=CARTESIAN_POINT ( 'NONE',  ( -95.00000000000000000, 171.6227766016838245, -27.69059892324149530 ) ) ;
#5829=CARTESIAN_POINT ( 'NONE',  ( -79.08918642097148677, 190.6879887351489060, -29.35163774059940067 ) ) ;
#5832=CARTESIAN_POINT ( 'NONE',  ( 48.00000000000000711, 175.6227766016838245, -5.571800142134975431 ) ) ;
#5834=CARTESIAN_POINT ( 'NONE',  ( -45.00000000000000000, 140.0000000000000000, -15.00000000000000000 ) ) ;
#5839=CARTESIAN_POINT ( 'NONE',  ( -80.00000000000002842, 146.6227766016838245, -13.00000000000000000 ) ) ;
#5841=ORIENTED_EDGE ( 'NONE', *, *, #3394, .T. ) ;
#5842=CARTESIAN_POINT ( 'NONE',  ( 33.66001102075547635, 19.99999999999999645, -12.05479157725600459 ) ) ;
#5843=AXIS2_PLACEMENT_3D ( 'NONE', #16482, #2761, #8504 ) ;
#5844=AXIS2_PLACEMENT_3D ( 'NONE', #5688, #11076, #3931 ) ;
#5846=CIRCLE ( 'NONE', #10649, 33.00000000000000000 ) ;
#5850=CARTESIAN_POINT ( 'NONE',  ( 225.0000000000000000, 89.99999999999997158, -15.00000000000000000 ) ) ;
#5851=ORIENTED_EDGE ( 'NONE', *, *, #7691, .T. ) ;
#5853=CARTESIAN_POINT ( 'NONE',  ( 37.25092477156690762, 148.5867852293671376, -23.63587233142070687 ) ) ;
#5854=EDGE_CURVE ( 'NONE', #9467, #14899, #3854, .T. ) ;
#5858=FACE_OUTER_BOUND ( 'NONE', #770, .T. ) ;
#5860=LINE ( 'NONE', #8781, #15107 ) ;
#5864=DIRECTION ( 'NONE',  ( 1.000000000000000000, 0.000000000000000000, 0.000000000000000000 ) ) ;
#5869=CARTESIAN_POINT ( 'NONE',  ( -14.26174088910747706, 32.16828253888332512, -10.14247415352539683 ) ) ;
#5876=ORIENTED_EDGE ( 'NONE', *, *, #2212, .T. ) ;
#5878=CARTESIAN_POINT ( 'NONE',  ( -80.00000000000002842, 146.6227766016838245, -35.00000000000000000 ) ) ;
#5879=CARTESIAN_POINT ( 'NONE',  ( 34.93420767853316988, 30.00000000000000000, -4.999999999999999112 ) ) ;
#5886=EDGE_LOOP ( 'NONE', ( #5278, #15599, #490, #17097 ) ) ;
#5889=LINE ( 'NONE', #16698, #7380 ) ;
#5892=CIRCLE ( 'NONE', #9835, 33.00000000000000000 ) ;
#5895=ORIENTED_EDGE ( 'NONE', *, *, #2234, .F. ) ;
#5901=DIRECTION ( 'NONE',  ( 0.000000000000000000, 0.000000000000000000, -1.000000000000000000 ) ) ;
#5906=CIRCLE ( 'NONE', #12967, 12.00000000000000000 ) ;
#5909=DIRECTION ( 'NONE',  ( -0.000000000000000000, -0.000000000000000000, -1.000000000000000000 ) ) ;
#5910=ORIENTED_EDGE ( 'NONE', *, *, #4471, .T. ) ;
#5913=CARTESIAN_POINT ( 'NONE',  ( -95.00000000000000000, 171.6227766016838245, 0.000000000000000000 ) ) ;
#5914=CARTESIAN_POINT ( 'NONE',  ( -8.720613081040568204, 20.00000000000000000, -24.99999999951824492 ) ) ;
#5915=DIRECTION ( 'NONE',  ( 0.000000000000000000, 0.000000000000000000, -1.000000000000000000 ) ) ;
#5916=AXIS2_PLACEMENT_3D ( 'NONE', #7346, #12751, #16629 ) ;
#5917=CIRCLE ( 'NONE', #13836, 6.000000000000005329 ) ;
#5919=CYLINDRICAL_SURFACE ( 'NONE', #6502, 2.500000000000000444 ) ;
#5920=EDGE_CURVE ( 'NONE', #9313, #4595, #14865, .T. ) ;
#5928=EDGE_LOOP ( 'NONE', ( #15128, #2448 ) ) ;
#5930=CARTESIAN_POINT ( 'NONE',  ( -43.00000000000000000, 140.0000000000000000, 0.000000000000000000 ) ) ;
#5931=AXIS2_PLACEMENT_3D ( 'NONE', #2901, #8559, #7066 ) ;
#5933=LINE ( 'NONE', #10304, #11213 ) ;
#5939=CARTESIAN_POINT ( 'NONE',  ( 30.00000000000001066, 146.6227766016838245, -12.99999999999999822 ) ) ;
#5940=ORIENTED_EDGE ( 'NONE', *, *, #9845, .F. ) ;
#5941=ORIENTED_EDGE ( 'NONE', *, *, #7843, .F. ) ;
#5942=CARTESIAN_POINT ( 'NONE',  ( 22.95484754400920124, 19.99999999999998934, -11.15425480658508306 ) ) ;
#5943=CIRCLE ( 'NONE', #11316, 239.9999999999999716 ) ;
#5946=VERTEX_POINT ( 'NONE', #17194 ) ;
#5948=AXIS2_PLACEMENT_3D ( 'NONE', #9633, #16286, #15115 ) ;
#5951=CYLINDRICAL_SURFACE ( 'NONE', #6783, 7.500000000000003553 ) ;
#5955=VECTOR ( 'NONE', #15050, 1000.000000000000000 ) ;
#5961=EDGE_LOOP ( 'NONE', ( #8883, #3624, #6841, #7009 ) ) ;
#5962=DIRECTION ( 'NONE',  ( 1.000000000000000000, 0.000000000000000000, 0.000000000000000000 ) ) ;
#5963=ORIENTED_EDGE ( 'NONE', *, *, #12607, .T. ) ;
#5964=EDGE_CURVE ( 'NONE', #8896, #160, #8367, .T. ) ;
#5966=CARTESIAN_POINT ( 'NONE',  ( -25.81010901361623056, 18.00000000000000000, -13.97188021846430139 ) ) ;
#5972=ORIENTED_EDGE ( 'NONE', *, *, #7869, .T. ) ;
#5973=FACE_OUTER_BOUND ( 'NONE', #1810, .T. ) ;
#5974=DIRECTION ( 'NONE',  ( -0.000000000000000000, -0.000000000000000000, -1.000000000000000000 ) ) ;
#5975=CYLINDRICAL_SURFACE ( 'NONE', #7896, 2.500000000000000444 ) ;
#5976=LINE ( 'NONE', #11366, #7657 ) ;
#5981=DIRECTION ( 'NONE',  ( -1.000000000000000000, 0.000000000000000000, 0.000000000000000000 ) ) ;
#5982=ORIENTED_EDGE ( 'NONE', *, *, #9588, .T. ) ;
#5983=EDGE_CURVE ( 'NONE', #15728, #7056, #11621, .T. ) ;
#5986=ORIENTED_EDGE ( 'NONE', *, *, #9161, .F. ) ;
#5987=ORIENTED_EDGE ( 'NONE', *, *, #10951, .T. ) ;
#5988=ADVANCED_FACE ( 'NONE', ( #10281 ), #8960, .T. ) ;
#5992=CARTESIAN_POINT ( 'NONE',  ( 30.00000000000000355, 196.6227766016838245, -12.99999999999999822 ) ) ;
#5993=ADVANCED_FACE ( 'NONE', ( #5069 ), #16581, .T. ) ;
#5995=LINE ( 'NONE', #8733, #9901 ) ;
#5997=DIRECTION ( 'NONE',  ( -1.000000000000000000, -0.000000000000000000, -0.000000000000000000 ) ) ;
#5998=CYLINDRICAL_SURFACE ( 'NONE', #9477, 7.500000000000003553 ) ;
#5999=ORIENTED_EDGE ( 'NONE', *, *, #12413, .T. ) ;
#6002=DIRECTION ( 'NONE',  ( 1.000000000000000000, 0.000000000000000000, 0.000000000000000000 ) ) ;
#6003=CARTESIAN_POINT ( 'NONE',  ( -13.66886994730069560, 31.37497952739824214, -13.17845503416513075 ) ) ;
#6006=VERTEX_POINT ( 'NONE', #7901 ) ;
#6007=CARTESIAN_POINT ( 'NONE',  ( 49.99999999999998579, 187.6227766016837961, -15.00000337241049486 ) ) ;
#6010=CARTESIAN_POINT ( 'NONE',  ( -85.72866685541674769, 194.8302331505971949, -26.20043099198422354 ) ) ;
#6011=CARTESIAN_POINT ( 'NONE',  ( -80.00000000000001421, 196.6227766016838245, -35.00000000000000000 ) ) ;
#6012=LINE ( 'NONE', #4684, #13405 ) ;
#6016=ADVANCED_FACE ( 'NONE', ( #6226 ), #14457, .T. ) ;
#6019=EDGE_CURVE ( 'NONE', #15920, #14931, #13470, .T. ) ;
#6021=ORIENTED_EDGE ( 'NONE', *, *, #6191, .F. ) ;
#6024=ORIENTED_EDGE ( 'NONE', *, *, #2073, .F. ) ;
#6026=LINE ( 'NONE', #10089, #10162 ) ;
#6027=ORIENTED_EDGE ( 'NONE', *, *, #8887, .T. ) ;
#6028=FACE_BOUND ( 'NONE', #9614, .T. ) ;
#6031=LINE ( 'NONE', #10000, #15406 ) ;
#6035=CARTESIAN_POINT ( 'NONE',  ( -77.50000000000002842, 146.6227766016838245, -16.00000000000000000 ) ) ;
#6037=EDGE_CURVE ( 'NONE', #8060, #4330, #8379, .T. ) ;
#6040=PLANE ( 'NONE',  #13243 ) ;
#6041=ORIENTED_EDGE ( 'NONE', *, *, #2079, .F. ) ;
#6043=DIRECTION ( 'NONE',  ( -0.000000000000000000, -0.000000000000000000, 1.000000000000000000 ) ) ;
#6045=DIRECTION ( 'NONE',  ( 0.000000000000000000, 0.000000000000000000, 1.000000000000000000 ) ) ;
#6049=FACE_OUTER_BOUND ( 'NONE', #13049, .T. ) ;
#6050=ADVANCED_FACE ( 'NONE', ( #1446 ), #8161, .T. ) ;
#6055=FACE_OUTER_BOUND ( 'NONE', #11656, .T. ) ;
#6056=ORIENTED_EDGE ( 'NONE', *, *, #17198, .F. ) ;
#6057=DIRECTION ( 'NONE',  ( -0.000000000000000000, -0.000000000000000000, -1.000000000000000000 ) ) ;
#6060=DIRECTION ( 'NONE',  ( 0.000000000000000000, -0.4999999999999952816, 0.8660254037844413721 ) ) ;
#6062=AXIS2_PLACEMENT_3D ( 'NONE', #14280, #15610, #2152 ) ;
#6063=ORIENTED_EDGE ( 'NONE', *, *, #12794, .F. ) ;
#6064=AXIS2_PLACEMENT_3D ( 'NONE', #14759, #12005, #15072 ) ;
#6065=ORIENTED_EDGE ( 'NONE', *, *, #1642, .F. ) ;
#6067=ORIENTED_EDGE ( 'NONE', *, *, #11396, .F. ) ;
#6069=ORIENTED_EDGE ( 'NONE', *, *, #11935, .T. ) ;
#6070=FACE_OUTER_BOUND ( 'NONE', #3696, .T. ) ;
#6071=EDGE_CURVE ( 'NONE', #3416, #9987, #13480, .T. ) ;
#6072=CARTESIAN_POINT ( 'NONE',  ( -75.00000000000000000, 196.6227766016838245, 0.000000000000000000 ) ) ;
#6075=DIRECTION ( 'NONE',  ( 0.000000000000000000, 0.000000000000000000, 1.000000000000000000 ) ) ;
#6079=DIRECTION ( 'NONE',  ( 1.000000000000000000, 0.000000000000000000, 0.000000000000000000 ) ) ;
#6081=CARTESIAN_POINT ( 'NONE',  ( -13.91527097789397160, 19.99999999999999645, -23.98152295253190758 ) ) ;
#6082=DIRECTION ( 'NONE',  ( 0.000000000000000000, 0.000000000000000000, 1.000000000000000000 ) ) ;
#6090=EDGE_LOOP ( 'NONE', ( #14275, #13033, #4314, #2729 ) ) ;
#6092=FACE_OUTER_BOUND ( 'NONE', #13347, .T. ) ;
#6093=CARTESIAN_POINT ( 'NONE',  ( 12.84413890157916782, 129.3215245152910313, -10.42375118840982573 ) ) ;
#6095=VECTOR ( 'NONE', #7828, 1000.000000000000000 ) ;
#6097=LINE ( 'NONE', #4861, #15523 ) ;
#6101=ORIENTED_EDGE ( 'NONE', *, *, #176, .F. ) ;
#6102=CIRCLE ( 'NONE', #737, 10.00000000000000178 ) ;
#6104=CARTESIAN_POINT ( 'NONE',  ( 23.77503517897789465, 19.99999999999999645, -22.95135521423388170 ) ) ;
#6105=CARTESIAN_POINT ( 'NONE',  ( -3.000000000000002665, 142.8100939375178200, -16.63501009223129756 ) ) ;
#6113=VECTOR ( 'NONE', #10748, 1000.000000000000000 ) ;
#6114=FACE_OUTER_BOUND ( 'NONE', #5639, .T. ) ;
#6115=UNCERTAINTY_MEASURE_WITH_UNIT (LENGTH_MEASURE( 1.000000000000000082E-05 ), #1398, 'distance_accuracy_value', 'NONE');
#6121=CARTESIAN_POINT ( 'NONE',  ( -95.00000000000000000, 141.6227766016838245, 5.510910596163088767E-15 ) ) ;
#6123=ORIENTED_EDGE ( 'NONE', *, *, #1226, .T. ) ;
#6126=ORIENTED_EDGE ( 'NONE', *, *, #7865, .F. ) ;
#6127=DIRECTION ( 'NONE',  ( -1.000000000000000000, -0.000000000000000000, 0.000000000000000000 ) ) ;
#6130=ORIENTED_EDGE ( 'NONE', *, *, #10104, .T. ) ;
#6132=EDGE_CURVE ( 'NONE', #16282, #14332, #10897, .T. ) ;
#6133=EDGE_CURVE ( 'NONE', #8547, #6832, #2854, .T. ) ;
#6138=CIRCLE ( 'NONE', #12647, 12.00000000000000000 ) ;
#6141=DIRECTION ( 'NONE',  ( 0.000000000000000000, 0.000000000000000000, 1.000000000000000000 ) ) ;
#6144=CARTESIAN_POINT ( 'NONE',  ( -40.00000000000000000, 20.00000000000000000, 0.000000000000000000 ) ) ;
#6145=VERTEX_POINT ( 'NONE', #13655 ) ;
#6146=DIRECTION ( 'NONE',  ( -1.000000000000000000, 0.000000000000000000, 0.000000000000000000 ) ) ;
#6148=EDGE_LOOP ( 'NONE', ( #16961, #14090, #16502, #6908 ) ) ;
#6149=CARTESIAN_POINT ( 'NONE',  ( 24.02486036880400277, 195.9845216101234939, -25.13379275193915063 ) ) ;
#6150=DIRECTION ( 'NONE',  ( 1.000000000000000000, 0.000000000000000000, -0.000000000000000000 ) ) ;
#6152=ORIENTED_EDGE ( 'NONE', *, *, #7734, .T. ) ;
#6154=ORIENTED_EDGE ( 'NONE', *, *, #12145, .F. ) ;
#6170=CARTESIAN_POINT ( 'NONE',  ( -40.00000000000000000, 20.00000000000000000, -30.00000000000000355 ) ) ;
#6171=CARTESIAN_POINT ( 'NONE',  ( -24.81085081035532269, 19.99999999999999645, -15.69149817756037457 ) ) ;
#6178=VECTOR ( 'NONE', #8753, 1000.000000000000000 ) ;
#6179=ORIENTED_EDGE ( 'NONE', *, *, #1328, .F. ) ;
#6184=LINE ( 'NONE', #11584, #1343 ) ;
#6191=EDGE_CURVE ( 'NONE', #7175, #8522, #1881, .T. ) ;
#6192=CARTESIAN_POINT ( 'NONE',  ( 20.42763382733002686, 19.99999999999999645, -24.23318166603087676 ) ) ;
#6193=B_SPLINE_CURVE_WITH_KNOTS ( 'NONE', 3,
 ( #3302, #14111, #4718, #10107, #15598, #14360, #12685, #562, #5966, #10009, #15512, #11780, #6381, #15946, #3821, #13471, #13381, #14450, #5061, #4968, #9123, #11874, #13116, #11961, #8059, #10539 ),
 .UNSPECIFIED., .F., .F.,
 ( 4, 2, 2, 2, 2, 2, 2, 2, 2, 2, 2, 2, 4 ),
 ( 0.000000000000000000, 0.002002783134349999609, 0.004005566268699999218, 0.008011132537399998435, 0.01001391567174999414, 0.01201669880609998985, 0.01602226507479997952, 0.01802504820914997002, 0.02002783134349995706, 0.02403339761219993806, 0.02603618074654992856, 0.02803896388089991906, 0.03204453014959990353 ),
 .UNSPECIFIED. ) ;
#6195=VERTEX_POINT ( 'NONE', #7987 ) ;
#6197=CARTESIAN_POINT ( 'NONE',  ( 7.010070850707991852, 140.5745599005093709, -12.93128425348633570 ) ) ;
#6199=EDGE_CURVE ( 'NONE', #5097, #793, #13392, .T. ) ;
#6200=ORIENTED_EDGE ( 'NONE', *, *, #2879, .T. ) ;
#6203=ADVANCED_FACE ( 'NONE', ( #9401 ), #14805, .T. ) ;
#6207=CARTESIAN_POINT ( 'NONE',  ( 34.93420767853318409, 18.00000000000000000, -5.000000000000010658 ) ) ;
#6209=CARTESIAN_POINT ( 'NONE',  ( 196.0000000000000000, 187.6227766016837961, -12.50000337241049309 ) ) ;
#6210=FACE_OUTER_BOUND ( 'NONE', #377, .T. ) ;
#6211=EDGE_LOOP ( 'NONE', ( #13976, #2774, #3893, #14071 ) ) ;
#6213=CIRCLE ( 'NONE', #569, 10.00000000000000000 ) ;
#6216=DIRECTION ( 'NONE',  ( -0.000000000000000000, -0.000000000000000000, -1.000000000000000000 ) ) ;
#6218=FACE_BOUND ( 'NONE', #16873, .T. ) ;
#6219=ORIENTED_EDGE ( 'NONE', *, *, #4895, .T. ) ;
#6224=VERTEX_POINT ( 'NONE', #4623 ) ;
#6226=FACE_OUTER_BOUND ( 'NONE', #7354, .T. ) ;
#6228=CARTESIAN_POINT ( 'NONE',  ( -16.47274440071381107, 31.95215739789422571, -10.50982007662407725 ) ) ;
#6231=FACE_OUTER_BOUND ( 'NONE', #1167, .T. ) ;
#6233=EDGE_CURVE ( 'NONE', #17520, #6671, #9499, .T. ) ;
#6235=ADVANCED_FACE ( 'NONE', ( #12499 ), #15141, .F. ) ;
#6236=ORIENTED_EDGE ( 'NONE', *, *, #4056, .F. ) ;
#6237=CARTESIAN_POINT ( 'NONE',  ( 33.36777657078724957, 191.6397216241468300, -28.71272404723382721 ) ) ;
#6239=CONICAL_SURFACE ( 'NONE', #4840, 33.26794919243112503, 0.5235987755983005920 ) ;
#6243=CARTESIAN_POINT ( 'NONE',  ( -74.91436539010484807, 152.1411297330830052, -26.63673872167001377 ) ) ;
#6249=AXIS2_PLACEMENT_3D ( 'NONE', #12606, #1807, #9680 ) ;
#6257=DIRECTION ( 'NONE',  ( -1.000000000000000000, 0.000000000000000000, 2.312964634635742464E-16 ) ) ;
#6260=VECTOR ( 'NONE', #4356, 1000.000000000000000 ) ;
#6264=CARTESIAN_POINT ( 'NONE',  ( -82.50000000000001421, 196.6227766016838245, 1.387778780781445676E-14 ) ) ;
#6266=CARTESIAN_POINT ( 'NONE',  ( -85.97513963119602920, 195.9845216101233802, -25.13379275193914353 ) ) ;
#6269=CARTESIAN_POINT ( 'NONE',  ( 15.41470791700940879, 125.6764093509959963, -6.286214449974339757 ) ) ;
#6271=FACE_OUTER_BOUND ( 'NONE', #8841, .T. ) ;
#6274=CARTESIAN_POINT ( 'NONE',  ( 29.09190978889357737, 202.5550951275239413, -16.37659873159347512 ) ) ;
#6275=VERTEX_POINT ( 'NONE', #8515 ) ;
#6277=CARTESIAN_POINT ( 'NONE',  ( 16.23418548573199516, 29.98246013044581915, -14.93677958672484785 ) ) ;
#6278=CARTESIAN_POINT ( 'NONE',  ( 12.89436750745977278, 141.9634372303913779, -18.58317047499899743 ) ) ;
#6279=VERTEX_POINT ( 'NONE', #12582 ) ;
#6283=PLANE ( 'NONE',  #13852 ) ;
#6289=CARTESIAN_POINT ( 'NONE',  ( 28.70390606474517625, 140.7594520581394022, -16.50672721711050528 ) ) ;
#6290=ORIENTED_EDGE ( 'NONE', *, *, #12388, .T. ) ;
#6292=ORIENTED_EDGE ( 'NONE', *, *, #14162, .T. ) ;
#6293=EDGE_CURVE ( 'NONE', #16965, #17478, #15164, .T. ) ;
#6296=FACE_BOUND ( 'NONE', #2400, .T. ) ;
#6297=ORIENTED_EDGE ( 'NONE', *, *, #8085, .F. ) ;
#6304=FACE_BOUND ( 'NONE', #5027, .T. ) ;
#6305=CARTESIAN_POINT ( 'NONE',  ( -17.59086657693884703, 18.00000000000000000, -22.42595686383721443 ) ) ;
#6307=ORIENTED_EDGE ( 'NONE', *, *, #8799, .T. ) ;
#6310=CARTESIAN_POINT ( 'NONE',  ( 35.39974920818285398, 194.0006876528842668, -26.91236748077486141 ) ) ;
#6312=( BOUNDED_CURVE ( )  B_SPLINE_CURVE ( 3, ( #14352, #14444, #17273, #17355 ),
 .UNSPECIFIED., .F., .F. ) 
 B_SPLINE_CURVE_WITH_KNOTS ( ( 4, 4 ),
 ( 3.141592653589792672, 4.712388980384690562 ),
 .UNSPECIFIED. ) 
 CURVE ( )  GEOMETRIC_REPRESENTATION_ITEM ( )  RATIONAL_B_SPLINE_CURVE ( ( 1.000000000000000000, 0.8047378541243646044, 0.8047378541243646044, 1.000000000000000000 ) ) 
 REPRESENTATION_ITEM ( '' )  );
#6316=CARTESIAN_POINT ( 'NONE',  ( -76.18268817859248543, 153.1022248993911887, -27.31438289289432220 ) ) ;
#6317=B_SPLINE_CURVE_WITH_KNOTS ( 'NONE', 3,
 ( #13342, #14666, #1206, #2630, #14488, #16181, #10403, #6609, #3966, #5279 ),
 .UNSPECIFIED., .F., .F.,
 ( 4, 2, 2, 2, 4 ),
 ( 0.03775390620236027117, 0.04033669301524707429, 0.04291947982813387741, 0.04550226664102068053, 0.04808505345390748364 ),
 .UNSPECIFIED. ) ;
#6318=ORIENTED_EDGE ( 'NONE', *, *, #3483, .T. ) ;
#6319=EDGE_CURVE ( 'NONE', #12075, #7078, #16491, .T. ) ;
#6320=DIRECTION ( 'NONE',  ( 0.000000000000000000, 0.000000000000000000, -1.000000000000000000 ) ) ;
#6322=CARTESIAN_POINT ( 'NONE',  ( 34.30925017698373836, 150.8166157800934570, -28.14689102807276555 ) ) ;
#6325=VECTOR ( 'NONE', #16950, 1000.000000000000000 ) ;
#6327=CYLINDRICAL_SURFACE ( 'NONE', #15207, 5.000000000000000888 ) ;
#6328=CYLINDRICAL_SURFACE ( 'NONE', #418, 33.00000000000000000 ) ;
#6329=CIRCLE ( 'NONE', #5498, 10.00000000000000178 ) ;
#6331=CARTESIAN_POINT ( 'NONE',  ( -26.90043998676167192, 19.99999999999999645, -11.53672424425260878 ) ) ;
#6335=EDGE_LOOP ( 'NONE', ( #13668, #4034, #2899, #7666 ) ) ;
#6336=DIRECTION ( 'NONE',  ( -0.000000000000000000, -0.000000000000000000, -1.000000000000000000 ) ) ;
#6340=EDGE_CURVE ( 'NONE', #16539, #152, #13104, .T. ) ;
#6343=ADVANCED_FACE ( 'NONE', ( #970 ), #11602, .F. ) ;
#6346=DIRECTION ( 'NONE',  ( 1.000000000000000000, 0.000000000000000000, 0.000000000000000000 ) ) ;
#6349=CARTESIAN_POINT ( 'NONE',  ( 22.93524650466158832, 29.84210526315789380, 0.000000000000000000 ) ) ;
#6350=DIRECTION ( 'NONE',  ( 0.000000000000000000, -1.000000000000000000, 0.000000000000000000 ) ) ;
#6351=DIRECTION ( 'NONE',  ( 0.000000000000000000, 0.000000000000000000, 1.000000000000000000 ) ) ;
#6352=CARTESIAN_POINT ( 'NONE',  ( 33.63492343075080271, 201.4000939832746155, -18.39459910103779450 ) ) ;
#6354=ORIENTED_EDGE ( 'NONE', *, *, #4333, .F. ) ;
#6356=ORIENTED_EDGE ( 'NONE', *, *, #3098, .F. ) ;
#6357=FACE_OUTER_BOUND ( 'NONE', #17082, .T. ) ;
#6358=ORIENTED_EDGE ( 'NONE', *, *, #14502, .T. ) ;
#6359=DIRECTION ( 'NONE',  ( -1.000000000000000000, 0.000000000000000000, 0.000000000000000000 ) ) ;
#6360=ORIENTED_EDGE ( 'NONE', *, *, #4592, .F. ) ;
#6361=DIRECTION ( 'NONE',  ( 0.000000000000000000, -0.000000000000000000, 1.000000000000000000 ) ) ;
#6362=CARTESIAN_POINT ( 'NONE',  ( 15.07980489400154056, 126.2730657262978724, -7.274180996386617970 ) ) ;
#6365=CIRCLE ( 'NONE', #12036, 7.500000000000000000 ) ;
#6375=DIRECTION ( 'NONE',  ( 0.000000000000000000, 1.000000000000000000, 0.000000000000000000 ) ) ;
#6376=ORIENTED_EDGE ( 'NONE', *, *, #16047, .T. ) ;
#6378=ORIENTED_EDGE ( 'NONE', *, *, #9107, .T. ) ;
#6381=CARTESIAN_POINT ( 'NONE',  ( -22.79696676584440596, 18.00000000000000711, -18.34105320469107170 ) ) ;
#6382=EDGE_CURVE ( 'NONE', #16806, #588, #5142, .T. ) ;
#6389=ORIENTED_EDGE ( 'NONE', *, *, #12004, .F. ) ;
#6390=DIRECTION ( 'NONE',  ( 1.000000000000000000, 0.000000000000000000, -0.000000000000000000 ) ) ;
#6393=AXIS2_PLACEMENT_3D ( 'NONE', #7613, #10350, #14609 ) ;
#6394=PLANE ( 'NONE',  #1672 ) ;
#6395=DIRECTION ( 'NONE',  ( 0.000000000000000000, 0.9938079899999064937, 0.1111111111111109523 ) ) ;
#6396=AXIS2_PLACEMENT_3D ( 'NONE', #4515, #7248, #858 ) ;
#6397=CARTESIAN_POINT ( 'NONE',  ( -12.54944958582184888, 31.64997543288135873, -11.54276402733058937 ) ) ;
#6400=CARTESIAN_POINT ( 'NONE',  ( -725.0000000000000000, 19.99999999999995737, -15.00000000000000000 ) ) ;
#6401=EDGE_LOOP ( 'NONE', ( #12213, #5941, #15271, #5160, #879 ) ) ;
#6402=CARTESIAN_POINT ( 'NONE',  ( -85.00000000000002842, 146.6227766016838245, 0.000000000000000000 ) ) ;
#6403=CARTESIAN_POINT ( 'NONE',  ( -87.50000000000004263, 196.6227766016838245, -21.54065922853802562 ) ) ;
#6405=ORIENTED_EDGE ( 'NONE', *, *, #10983, .F. ) ;
#6406=ORIENTED_EDGE ( 'NONE', *, *, #9562, .T. ) ;
#6407=VECTOR ( 'NONE', #10257, 1000.000000000000000 ) ;
#6408=AXIS2_PLACEMENT_3D ( 'NONE', #11135, #15480, #13987 ) ;
#6410=CARTESIAN_POINT ( 'NONE',  ( -75.73052444394195959, 152.8115259536291148, -27.11642929875282348 ) ) ;
#6418=CARTESIAN_POINT ( 'NONE',  ( 24.10468692392765533, 147.7508872708765750, -25.59654897292658049 ) ) ;
#6422=DIRECTION ( 'NONE',  ( -1.000000000000000000, -0.000000000000000000, -0.000000000000000000 ) ) ;
#6428=CARTESIAN_POINT ( 'NONE',  ( -27.99999999999998224, 4.000000000000000000, -30.00000000000000711 ) ) ;
#6430=DIRECTION ( 'NONE',  ( -0.000000000000000000, -0.000000000000000000, -1.000000000000000000 ) ) ;
#6431=CIRCLE ( 'NONE', #14340, 6.000000000000005329 ) ;
#6432=EDGE_CURVE ( 'NONE', #6602, #13323, #14601, .T. ) ;
#6434=ORIENTED_EDGE ( 'NONE', *, *, #5703, .T. ) ;
#6441=CARTESIAN_POINT ( 'NONE',  ( -86.00000000000001421, 146.2509476181505477, -24.11540106065089262 ) ) ;
#6443=VERTEX_POINT ( 'NONE', #15589 ) ;
#6447=DIRECTION ( 'NONE',  ( 0.000000000000000000, 0.000000000000000000, 1.000000000000000000 ) ) ;
#6452=ORIENTED_EDGE ( 'NONE', *, *, #4182, .T. ) ;
#6455=FACE_OUTER_BOUND ( 'NONE', #1595, .T. ) ;
#6458=CARTESIAN_POINT ( 'NONE',  ( 11.61604111307750209, 130.6582085322020532, -11.34316963496758390 ) ) ;
#6459=EDGE_LOOP ( 'NONE', ( #8751, #3686, #888, #5772 ) ) ;
#6460=CARTESIAN_POINT ( 'NONE',  ( 30.49999999999998224, 9.999999999999998224, -16.00000000000000000 ) ) ;
#6461=CARTESIAN_POINT ( 'NONE',  ( -3.000000000000000888, 171.6227766016838245, 0.000000000000000000 ) ) ;
#6462=DIRECTION ( 'NONE',  ( 0.000000000000000000, 1.000000000000000000, 0.000000000000000000 ) ) ;
#6466=CARTESIAN_POINT ( 'NONE',  ( 0.000000000000000000, 0.000000000000000000, -33.00000000000000711 ) ) ;
#6468=CARTESIAN_POINT ( 'NONE',  ( -5.000000000000004441, 142.8100939375178200, -16.63501009223129756 ) ) ;
#6469=LINE ( 'NONE', #12043, #821 ) ;
#6471=CARTESIAN_POINT ( 'NONE',  ( 34.99061305271412436, 143.2738031352136545, -20.53261660472919203 ) ) ;
#6473=DIRECTION ( 'NONE',  ( 8.673617379884037937E-17, 0.000000000000000000, 1.000000000000000000 ) ) ;
#6474=ADVANCED_FACE ( 'NONE', ( #14258 ), #10264, .F. ) ;
#6476=VERTEX_POINT ( 'NONE', #2125 ) ;
#6480=AXIS2_PLACEMENT_3D ( 'NONE', #9492, #15066, #13585 ) ;
#6484=ORIENTED_EDGE ( 'NONE', *, *, #1597, .T. ) ;
#6486=ORIENTED_EDGE ( 'NONE', *, *, #7972, .F. ) ;
#6487=CARTESIAN_POINT ( 'NONE',  ( 48.00000000000000711, 171.6227766016838245, 0.000000000000000000 ) ) ;
#6488=CARTESIAN_POINT ( 'NONE',  ( 24.54894360611539028, 191.4650750923992177, -26.36917907415269013 ) ) ;
#6490=CARTESIAN_POINT ( 'NONE',  ( 27.44407568426044008, 126.9014170516880284, -4.999999999999997335 ) ) ;
#6491=CARTESIAN_POINT ( 'NONE',  ( -10.13698291596435119, 17.99999999999999645, -11.46558158188963539 ) ) ;
#6494=ORIENTED_EDGE ( 'NONE', *, *, #15639, .F. ) ;
#6496=EDGE_LOOP ( 'NONE', ( #4655, #3007 ) ) ;
#6497=CARTESIAN_POINT ( 'NONE',  ( 24.27133314458328428, 194.8302331505971665, -26.20043099198421288 ) ) ;
#6498=CARTESIAN_POINT ( 'NONE',  ( -85.27494917608791525, 201.9542783778900059, -13.00000000000000000 ) ) ;
#6500=ORIENTED_EDGE ( 'NONE', *, *, #3936, .F. ) ;
#6501=EDGE_LOOP ( 'NONE', ( #9364, #13451, #16033, #2588 ) ) ;
#6502=AXIS2_PLACEMENT_3D ( 'NONE', #780, #14234, #16891 ) ;
#6503=VECTOR ( 'NONE', #6740, 1000.000000000000000 ) ;
#6506=VECTOR ( 'NONE', #16810, 1000.000000000000000 ) ;
#6507=EDGE_LOOP ( 'NONE', ( #10396, #3232, #6027, #8315 ) ) ;
#6509=DIRECTION ( 'NONE',  ( 1.000000000000000000, 0.000000000000000000, 0.000000000000000000 ) ) ;
#6511=CARTESIAN_POINT ( 'NONE',  ( 24.13838555012902276, 147.9152928535323213, -25.74888847741386044 ) ) ;
#6515=ORIENTED_EDGE ( 'NONE', *, *, #11929, .F. ) ;
#6516=CARTESIAN_POINT ( 'NONE',  ( -100.0000000000000000, 100.0000000000000142, -6.000000000000000000 ) ) ;
#6517=VECTOR ( 'NONE', #11818, 1000.000000000000000 ) ;
#6520=CYLINDRICAL_SURFACE ( 'NONE', #1578, 27.69059892324149530 ) ;
#6521=AXIS2_PLACEMENT_3D ( 'NONE', #11638, #17043, #6320 ) ;
#6522=CARTESIAN_POINT ( 'NONE',  ( -18.18164784767110120, 32.29378831700660157, -6.323624269675778287 ) ) ;
#6526=EDGE_CURVE ( 'NONE', #13081, #4701, #12633, .T. ) ;
#6527=EDGE_CURVE ( 'NONE', #12225, #8437, #13199, .T. ) ;
#6532=DIRECTION ( 'NONE',  ( 0.000000000000000000, 0.000000000000000000, 1.000000000000000000 ) ) ;
#6534=ORIENTED_EDGE ( 'NONE', *, *, #7414, .F. ) ;
#6538=CARTESIAN_POINT ( 'NONE',  ( -79.72426293143250575, 140.6276388071887880, -16.25736180127251629 ) ) ;
#6542=FACE_OUTER_BOUND ( 'NONE', #8787, .T. ) ;
#6545=ORIENTED_EDGE ( 'NONE', *, *, #11421, .F. ) ;
#6547=CARTESIAN_POINT ( 'NONE',  ( 6.851232759387628768, 134.0993825829163200, -14.99999999999999822 ) ) ;
#6548=ORIENTED_EDGE ( 'NONE', *, *, #1794, .F. ) ;
#6549=CARTESIAN_POINT ( 'NONE',  ( -80.92353557482439896, 152.5685199100058753, -29.35899209070758786 ) ) ;
#6550=CARTESIAN_POINT ( 'NONE',  ( 10.76597736162413632, 139.9178931572356532, -11.43282512092270053 ) ) ;
#6554=B_SPLINE_CURVE_WITH_KNOTS ( 'NONE', 3,
 ( #15711, #5265, #9247, #6418, #6511, #7656, #13412, #9340, #17310, #13066, #8005, #3859, #10665, #932, #5004, #14478, #14747, #11903, #3590, #10391, #15805, #7733, #11717, #12085, #13240, #2431, #10303, #8983, #13145, #7829, #1196, #6599, #16076, #1111, #14559, #17216, #6322, #13330, #4912, #3683, #11990, #5094, #10487, #2619 ),
 .UNSPECIFIED., .F., .F.,
 ( 4, 2, 2, 2, 2, 2, 2, 2, 2, 2, 2, 2, 2, 2, 2, 2, 2, 2, 2, 2, 2, 4 ),
 ( 0.02539562174428236160, 0.02674754696500278306, 0.02742350957536299205, 0.02809947218572320105, 0.02945139740644361903, 0.03012736001680382456, 0.03080332262716403008, 0.03215524784788444806, 0.03283121045824467787, 0.03350717306860491462, 0.03418313567896515137, 0.03485909828932538118, 0.03621102351004584774, 0.03688698612040607061, 0.03756294873076629348, 0.03891487395148671147, 0.03959083656184691352, 0.04026679917220711558, 0.04161872439292756132, 0.04297064961364800706, 0.04432257483436844586, 0.04702642527580933041 ),
 .UNSPECIFIED. ) ;
#6555=DIRECTION ( 'NONE',  ( 1.000000000000000000, 0.000000000000000000, -0.000000000000000000 ) ) ;
#6557=ADVANCED_FACE ( 'NONE', ( #13638 ), #13458, .F. ) ;
#6558=CARTESIAN_POINT ( 'NONE',  ( -90.80384757729339640, 171.6227766016838245, 0.000000000000000000 ) ) ;
#6562=DIRECTION ( 'NONE',  ( 0.000000000000000000, 0.000000000000000000, 1.000000000000000000 ) ) ;
#6564=CARTESIAN_POINT ( 'NONE',  ( 28.23642206097335006, 140.8827219813066449, -16.73516917262794479 ) ) ;
#6565=ORIENTED_EDGE ( 'NONE', *, *, #11863, .F. ) ;
#6566=CARTESIAN_POINT ( 'NONE',  ( 12.80996511848405994, 130.8496636614418094, -12.93682947221565804 ) ) ;
#6567=CARTESIAN_POINT ( 'NONE',  ( -13.90980987654335976, 19.99999999999998934, -23.98326992096530219 ) ) ;
#6577=EDGE_CURVE ( 'NONE', #7719, #7374, #11706, .T. ) ;
#6580=DIRECTION ( 'NONE',  ( -0.000000000000000000, -0.000000000000000000, 1.000000000000000000 ) ) ;
#6581=CARTESIAN_POINT ( 'NONE',  ( 30.56347832044301782, 189.1215240515806499, -27.97845313684487678 ) ) ;
#6582=DIRECTION ( 'NONE',  ( -0.000000000000000000, -1.000000000000000000, 0.000000000000000000 ) ) ;
#6583=CARTESIAN_POINT ( 'NONE',  ( -16.30611068361414695, 32.76923076921517008, -5.528684565802741702 ) ) ;
#6586=CARTESIAN_POINT ( 'NONE',  ( 49.99999999999998579, 187.6227766016837961, -12.50000337241049309 ) ) ;
#6588=CARTESIAN_POINT ( 'NONE',  ( -73.91032892519172037, 192.2167777214562250, -25.78994361341036523 ) ) ;
#6590=VERTEX_POINT ( 'NONE', #2915 ) ;
#6594=CARTESIAN_POINT ( 'NONE',  ( -74.06456496986170635, 151.2142461003564335, -25.93356563065114528 ) ) ;
#6597=CARTESIAN_POINT ( 'NONE',  ( 27.47046887122067105, 138.6908793960143669, -2.448156880351273657 ) ) ;
#6599=CARTESIAN_POINT ( 'NONE',  ( 32.79231225559605889, 151.9379092097359205, -28.93992015514735172 ) ) ;
#6600=CARTESIAN_POINT ( 'NONE',  ( -80.00000000000001421, 196.6227766016838245, -16.00000000000000000 ) ) ;
#6601=DIRECTION ( 'NONE',  ( -1.000000000000000000, -0.000000000000000000, 0.000000000000000000 ) ) ;
#6602=VERTEX_POINT ( 'NONE', #17350 ) ;
#6603=CARTESIAN_POINT ( 'NONE',  ( -80.51989362019833152, 202.6059057426778622, -16.28038605903245539 ) ) ;
#6604=CARTESIAN_POINT ( 'NONE',  ( 21.04314855419486108, 29.91877537971376455, -12.94423386069545323 ) ) ;
#6607=CARTESIAN_POINT ( 'NONE',  ( -35.49999999999998579, 10.00000000000000178, -28.00000000000000355 ) ) ;
#6609=CARTESIAN_POINT ( 'NONE',  ( -85.89213624354479748, 141.9593924407984957, -14.48320912595414711 ) ) ;
#6610=DIRECTION ( 'NONE',  ( 0.000000000000000000, 0.000000000000000000, 1.000000000000000000 ) ) ;
#6612=EDGE_CURVE ( 'NONE', #14270, #7418, #17146, .T. ) ;
#6613=ORIENTED_EDGE ( 'NONE', *, *, #5218, .T. ) ;
#6614=EDGE_CURVE ( 'NONE', #2922, #16329, #9514, .T. ) ;
#6615=DIRECTION ( 'NONE',  ( -1.000000000000000000, 0.000000000000000000, 8.673617379884037937E-17 ) ) ;
#6622=CARTESIAN_POINT ( 'NONE',  ( -85.34448289831571799, 143.8733932267928424, -21.33602313251873639 ) ) ;
#6625=EDGE_CURVE ( 'NONE', #15082, #11068, #11771, .T. ) ;
#6627=CARTESIAN_POINT ( 'NONE',  ( 49.99999999999998579, 159.6227766016838814, -5.571800142134975431 ) ) ;
#6629=DIRECTION ( 'NONE',  ( -1.000000000000000000, 0.000000000000000000, 0.000000000000000000 ) ) ;
#6630=PLANE ( 'NONE',  #13148 ) ;
#6632=AXIS2_PLACEMENT_3D ( 'NONE', #16759, #10003, #7183 ) ;
#6636=CARTESIAN_POINT ( 'NONE',  ( -85.86161444987101277, 147.9152928535322928, -25.74888847741385689 ) ) ;
#6637=CARTESIAN_POINT ( 'NONE',  ( 16.61152767523464391, 142.9573811237880534, -16.36000751420521837 ) ) ;
#6641=CARTESIAN_POINT ( 'NONE',  ( -50.00000000000000000, 171.6227766016838245, 0.000000000000000000 ) ) ;
#6642=DIRECTION ( 'NONE',  ( -0.000000000000000000, -0.000000000000000000, -1.000000000000000000 ) ) ;
#6643=DIRECTION ( 'NONE',  ( 0.000000000000000000, 0.000000000000000000, -1.000000000000000000 ) ) ;
#6646=CARTESIAN_POINT ( 'NONE',  ( 22.25017171248248005, 17.99999999999544542, -8.611421531743401303 ) ) ;
#6648=FACE_OUTER_BOUND ( 'NONE', #4985, .T. ) ;
#6650=DIRECTION ( 'NONE',  ( 1.000000000000000000, 0.000000000000000000, 0.000000000000000000 ) ) ;
#6651=CARTESIAN_POINT ( 'NONE',  ( 196.0000000000000000, 187.6227766016837961, -12.50000337241049309 ) ) ;
#6653=CARTESIAN_POINT ( 'NONE',  ( 17.39133856982844506, 125.9242906883583970, -6.521754810248964418 ) ) ;
#6654=ORIENTED_EDGE ( 'NONE', *, *, #1160, .F. ) ;
#6662=VERTEX_POINT ( 'NONE', #11058 ) ;
#6666=CARTESIAN_POINT ( 'NONE',  ( -95.00000000000000000, 143.9321776784423150, 5.086680500673126297E-15 ) ) ;
#6667=DIRECTION ( 'NONE',  ( 0.000000000000000000, 0.000000000000000000, -1.000000000000000000 ) ) ;
#6668=CARTESIAN_POINT ( 'NONE',  ( 196.0000000000000000, 159.6227766016838814, -3.071800142134975431 ) ) ;
#6669=CARTESIAN_POINT ( 'NONE',  ( -11.82448321327245466, 31.42688426858654438, -11.97038274549936254 ) ) ;
#6671=VERTEX_POINT ( 'NONE', #9722 ) ;
#6675=DIRECTION ( 'NONE',  ( 0.000000000000000000, -0.8660254037844413721, -0.4999999999999953371 ) ) ;
#6676=CARTESIAN_POINT ( 'NONE',  ( 39.99999999999998579, 20.00000000000000000, -30.00000000000001066 ) ) ;
#6679=EDGE_CURVE ( 'NONE', #4216, #5512, #4517, .T. ) ;
#6681=ORIENTED_EDGE ( 'NONE', *, *, #13254, .F. ) ;
#6683=ORIENTED_EDGE ( 'NONE', *, *, #3593, .F. ) ;
#6684=AXIS2_PLACEMENT_3D ( 'NONE', #6487, #2323, #3565 ) ;
#6689=DIRECTION ( 'NONE',  ( 1.000000000000000000, 0.000000000000000000, -0.000000000000000000 ) ) ;
#6690=DIRECTION ( 'NONE',  ( -0.000000000000000000, -0.000000000000000000, -1.000000000000000000 ) ) ;
#6693=EDGE_LOOP ( 'NONE', ( #16160, #11336, #8290, #3152 ) ) ;
#6705=DIRECTION ( 'NONE',  ( -0.000000000000000000, -0.000000000000000000, -1.000000000000000000 ) ) ;
#6709=VERTEX_POINT ( 'NONE', #7343 ) ;
#6712=CARTESIAN_POINT ( 'NONE',  ( -78.22549311270449834, 140.8861252344925106, -16.74142298344136393 ) ) ;
#6713=AXIS2_PLACEMENT_3D ( 'NONE', #16993, #8670, #7423 ) ;
#6719=CARTESIAN_POINT ( 'NONE',  ( -72.50000000000000000, 196.6227766016838245, -13.00000000000000000 ) ) ;
#6722=CARTESIAN_POINT ( 'NONE',  ( 225.0000000000000000, 89.99999999999997158, -15.00000000000000000 ) ) ;
#6724=CARTESIAN_POINT ( 'NONE',  ( 16.34705933256690713, 136.9208395216682561, -6.505922558274787271 ) ) ;
#6726=ORIENTED_EDGE ( 'NONE', *, *, #9353, .F. ) ;
#6728=VECTOR ( 'NONE', #4723, 1000.000000000000000 ) ;
#6729=CARTESIAN_POINT ( 'NONE',  ( 14.12560798726494760, 138.8049619564753243, -7.597757983846324947 ) ) ;
#6730=VERTEX_POINT ( 'NONE', #7083 ) ;
#6731=DIRECTION ( 'NONE',  ( 0.000000000000000000, 0.000000000000000000, 1.000000000000000000 ) ) ;
#6734=CARTESIAN_POINT ( 'NONE',  ( 30.00000000000001066, 146.6227766016838245, 1.387778780781445676E-14 ) ) ;
#6735=CARTESIAN_POINT ( 'NONE',  ( 16.25302816831168329, 18.00000000000000000, -25.00000000000000000 ) ) ;
#6736=CARTESIAN_POINT ( 'NONE',  ( 22.51491806150639974, 29.85019096660411364, -7.572044396946283840 ) ) ;
#6737=LINE ( 'NONE', #90, #2757 ) ;
#6740=DIRECTION ( 'NONE',  ( 1.000000000000000000, 0.000000000000000000, 0.000000000000000000 ) ) ;
#6745=ORIENTED_EDGE ( 'NONE', *, *, #305, .T. ) ;
#6746=CARTESIAN_POINT ( 'NONE',  ( 14.34366722128227067, 129.4994645064758174, -11.74322308516846647 ) ) ;
#6750=LINE ( 'NONE', #1604, #4143 ) ;
#6751=ORIENTED_EDGE ( 'NONE', *, *, #8084, .F. ) ;
#6754=EDGE_CURVE ( 'NONE', #16058, #3029, #6012, .T. ) ;
#6756=VERTEX_POINT ( 'NONE', #3264 ) ;
#6757=VECTOR ( 'NONE', #9466, 1000.000000000000000 ) ;
#6758=CARTESIAN_POINT ( 'NONE',  ( 14.93242934743710393, 30.00000000000000000, -13.00000000000000178 ) ) ;
#6759=CIRCLE ( 'NONE', #16655, 6.000000000000005329 ) ;
#6761=DIRECTION ( 'NONE',  ( 1.000000000000000000, 0.000000000000000000, 0.000000000000000000 ) ) ;
#6762=CARTESIAN_POINT ( 'NONE',  ( 37.46328901163953162, 195.8564978660714360, -22.40111672564487222 ) ) ;
#6765=CARTESIAN_POINT ( 'NONE',  ( -22.99999999999999645, 100.0000000000000142, -15.00000000000000000 ) ) ;
#6766=ORIENTED_EDGE ( 'NONE', *, *, #625, .F. ) ;
#6771=CARTESIAN_POINT ( 'NONE',  ( -84.88846745512550740, 190.9286879163519757, -26.76420670456570505 ) ) ;
#6778=CIRCLE ( 'NONE', #16400, 2.500000000000002220 ) ;
#6779=ORIENTED_EDGE ( 'NONE', *, *, #15701, .T. ) ;
#6782=CYLINDRICAL_SURFACE ( 'NONE', #7090, 20.00000000000000355 ) ;
#6783=AXIS2_PLACEMENT_3D ( 'NONE', #17083, #809, #2213 ) ;
#6785=CARTESIAN_POINT ( 'NONE',  ( -80.00000000000001421, 196.6227766016838245, -35.00200000000000244 ) ) ;
#6787=LINE ( 'NONE', #12348, #3147 ) ;
#6792=CARTESIAN_POINT ( 'NONE',  ( -81.03644165218622675, 202.5339273643435547, -16.41656018636075132 ) ) ;
#6799=DIRECTION ( 'NONE',  ( 0.000000000000000000, 0.000000000000000000, -1.000000000000000000 ) ) ;
#6800=ORIENTED_EDGE ( 'NONE', *, *, #10599, .T. ) ;
#6801=DIRECTION ( 'NONE',  ( -1.000000000000000000, -0.000000000000000000, -0.000000000000000000 ) ) ;
#6802=ORIENTED_EDGE ( 'NONE', *, *, #8168, .T. ) ;
#6804=VECTOR ( 'NONE', #16263, 1000.000000000000000 ) ;
#6806=AXIS2_PLACEMENT_3D ( 'NONE', #5372, #5795, #1812 ) ;
#6808=EDGE_CURVE ( 'NONE', #2922, #15641, #8324, .T. ) ;
#6812=DIRECTION ( 'NONE',  ( -0.000000000000000000, -0.000000000000000000, -1.000000000000000000 ) ) ;
#6813=CARTESIAN_POINT ( 'NONE',  ( -3.000000000000000888, 171.6227766016838245, 0.000000000000000000 ) ) ;
#6814=DIRECTION ( 'NONE',  ( -0.000000000000000000, -0.000000000000000000, 1.000000000000000000 ) ) ;
#6815=VECTOR ( 'NONE', #8541, 1000.000000000000000 ) ;
#6816=CARTESIAN_POINT ( 'NONE',  ( 14.18611645313626290, 129.6406627243902676, -11.87032202561248617 ) ) ;
#6818=CARTESIAN_POINT ( 'NONE',  ( -27.99999999999998224, 10.00000000000000000, -30.00000000000000355 ) ) ;
#6820=CARTESIAN_POINT ( 'NONE',  ( 196.0000000000000000, 171.6227766016838245, -15.00000337241049131 ) ) ;
#6822=LINE ( 'NONE', #13634, #3108 ) ;
#6823=EDGE_CURVE ( 'NONE', #11878, #102, #14420, .T. ) ;
#6825=CARTESIAN_POINT ( 'NONE',  ( 32.29638371061065527, 18.00000000000000000, -15.01265034258821096 ) ) ;
#6826=CARTESIAN_POINT ( 'NONE',  ( 30.80964797964692536, 18.00000000000000000, -17.18170494867161224 ) ) ;
#6829=DIRECTION ( 'NONE',  ( -0.000000000000000000, -0.000000000000000000, -1.000000000000000000 ) ) ;
#6830=DIRECTION ( 'NONE',  ( 0.000000000000000000, 0.000000000000000000, 1.000000000000000000 ) ) ;
#6831=CARTESIAN_POINT ( 'NONE',  ( 24.00000000000000711, 146.2509476181506329, -24.11540106065089262 ) ) ;
#6832=VERTEX_POINT ( 'NONE', #11741 ) ;
#6834=EDGE_LOOP ( 'NONE', ( #16175, #10831 ) ) ;
#6836=LINE ( 'NONE', #3011, #1602 ) ;
#6838=CARTESIAN_POINT ( 'NONE',  ( 22.93524650466160963, 29.84210526315773748, -4.999999999999999112 ) ) ;
#6839=DIRECTION ( 'NONE',  ( -0.000000000000000000, -0.000000000000000000, 1.000000000000000000 ) ) ;
#6841=ORIENTED_EDGE ( 'NONE', *, *, #1031, .F. ) ;
#6842=CARTESIAN_POINT ( 'NONE',  ( 22.53671098836050746, 147.3890553372962700, -22.40111672564484024 ) ) ;
#6843=EDGE_CURVE ( 'NONE', #10402, #2789, #11424, .T. ) ;
#6844=ORIENTED_EDGE ( 'NONE', *, *, #10609, .F. ) ;
#6845=CARTESIAN_POINT ( 'NONE',  ( -90.80384757729339640, 204.6227766016838245, 0.000000000000000000 ) ) ;
#6848=VERTEX_POINT ( 'NONE', #2285 ) ;
#6849=LINE ( 'NONE', #6765, #12858 ) ;
#6851=EDGE_CURVE ( 'NONE', #9797, #4327, #15737, .T. ) ;
#6852=ORIENTED_EDGE ( 'NONE', *, *, #2678, .T. ) ;
#6855=CARTESIAN_POINT ( 'NONE',  ( -86.47240542152535170, 192.8264746069454816, -25.28784208911848808 ) ) ;
#6856=CARTESIAN_POINT ( 'NONE',  ( -100.0000000000000000, 171.6227766016838245, 0.000000000000000000 ) ) ;
#6858=EDGE_LOOP ( 'NONE', ( #3396, #6069, #8709, #3848 ) ) ;
#6867=CARTESIAN_POINT ( 'NONE',  ( -75.00000000000002842, 146.6227766016838245, 0.000000000000000000 ) ) ;
#6868=ORIENTED_EDGE ( 'NONE', *, *, #2877, .F. ) ;
#6869=CARTESIAN_POINT ( 'NONE',  ( -77.02080656390279501, 201.8349995435116568, -17.67084604013262350 ) ) ;
#6873=DIRECTION ( 'NONE',  ( -0.000000000000000000, -0.000000000000000000, -1.000000000000000000 ) ) ;
#6876=EDGE_CURVE ( 'NONE', #7826, #12193, #3231, .T. ) ;
#6878=ORIENTED_EDGE ( 'NONE', *, *, #1599, .F. ) ;
#6883=DIRECTION ( 'NONE',  ( 0.000000000000000000, -1.000000000000000000, 0.000000000000000000 ) ) ;
#6886=CARTESIAN_POINT ( 'NONE',  ( 15.80099858973940030, 127.9994182179736413, -10.08996921773076316 ) ) ;
#6887=EDGE_CURVE ( 'NONE', #14780, #539, #14817, .T. ) ;
#6889=ADVANCED_FACE ( 'NONE', ( #5119 ), #2103, .F. ) ;
#6890=ORIENTED_EDGE ( 'NONE', *, *, #7068, .T. ) ;
#6892=EDGE_LOOP ( 'NONE', ( #7050, #8057 ) ) ;
#6893=DIRECTION ( 'NONE',  ( 0.000000000000000000, 0.000000000000000000, 1.000000000000000000 ) ) ;
#6894=DIRECTION ( 'NONE',  ( -1.000000000000000000, -0.000000000000000000, 0.000000000000000000 ) ) ;
#6898=DIRECTION ( 'NONE',  ( -1.000000000000000000, -0.000000000000000000, 0.000000000000000000 ) ) ;
#6900=CARTESIAN_POINT ( 'NONE',  ( 14.93242934743711992, 18.00000000000000355, -25.00000000000000000 ) ) ;
#6903=CARTESIAN_POINT ( 'NONE',  ( -10.04118010627649049, 19.99999999999999645, -24.87462214923097648 ) ) ;
#6907=FACE_OUTER_BOUND ( 'NONE', #2551, .T. ) ;
#6908=ORIENTED_EDGE ( 'NONE', *, *, #16040, .F. ) ;
#6911=ORIENTED_EDGE ( 'NONE', *, *, #14421, .F. ) ;
#6912=CARTESIAN_POINT ( 'NONE',  ( 36.47240542152533749, 150.4190785964221675, -25.28784208911848808 ) ) ;
#6914=VERTEX_POINT ( 'NONE', #8026 ) ;
#6915=CIRCLE ( 'NONE', #2963, 2.500000000000002220 ) ;
#6917=CARTESIAN_POINT ( 'NONE',  ( 36.08967107480828673, 192.2167777214563102, -25.78994361341037944 ) ) ;
#6926=CARTESIAN_POINT ( 'NONE',  ( -87.50000000000004263, 196.6227766016838245, -21.54065922853802562 ) ) ;
#6927=LINE ( 'NONE', #5611, #1872 ) ;
#6929=CARTESIAN_POINT ( 'NONE',  ( -16.28901493728125160, 32.76428253546148284, -5.573780508339472028 ) ) ;
#6933=VECTOR ( 'NONE', #2878, 1000.000000000000114 ) ;
#6934=CARTESIAN_POINT ( 'NONE',  ( -72.50000000000000000, 197.1883573205068103, -20.88424858573643661 ) ) ;
#6937=ORIENTED_EDGE ( 'NONE', *, *, #5722, .T. ) ;
#6940=DIRECTION ( 'NONE',  ( 1.000000000000000000, 0.000000000000000000, 0.000000000000000000 ) ) ;
#6941=VECTOR ( 'NONE', #8982, 1000.000000000000000 ) ;
#6942=CARTESIAN_POINT ( 'NONE',  ( 22.51550247401197069, 29.85017970947654575, -7.570302168957804057 ) ) ;
#6943=CIRCLE ( 'NONE', #10058, 248.0000000000000000 ) ;
#6944=CARTESIAN_POINT ( 'NONE',  ( 27.99999999999998224, 9.999999999999998224, 0.000000000000000000 ) ) ;
#6946=AXIS2_PLACEMENT_3D ( 'NONE', #12469, #5738, #11125 ) ;
#6953=ADVANCED_FACE ( 'NONE', ( #10782 ), #5790, .T. ) ;
#6957=ORIENTED_EDGE ( 'NONE', *, *, #4029, .T. ) ;
#6960=LINE ( 'NONE', #234, #1433 ) ;
#6961=CIRCLE ( 'NONE', #7795, 7.500000000000020428 ) ;
#6965=EDGE_CURVE ( 'NONE', #9959, #11342, #13869, .T. ) ;
#6970=VECTOR ( 'NONE', #4796, 1000.000000000000000 ) ;
#6972=CARTESIAN_POINT ( 'NONE',  ( 22.50000000000000000, 196.6227766016838245, -21.54065922853802562 ) ) ;
#6973=CARTESIAN_POINT ( 'NONE',  ( -50.00000000000000000, 154.3022685259950038, -9.999999999999900524 ) ) ;
#6978=CARTESIAN_POINT ( 'NONE',  ( 26.46962346220079709, 137.6228726052619606, -8.310907492956932430 ) ) ;
#6981=CARTESIAN_POINT ( 'NONE',  ( -725.0000000000000000, 19.99999999999995737, -13.00000000000000000 ) ) ;
#6985=CARTESIAN_POINT ( 'NONE',  ( -80.90398788703467403, 190.6868548533384171, -29.35237411376977334 ) ) ;
#6988=CARTESIAN_POINT ( 'NONE',  ( -725.0000000000001137, 129.9999999999995453, -4.999999999999999112 ) ) ;
#6999=CARTESIAN_POINT ( 'NONE',  ( -15.53366225407947354, 31.76144936975385136, -11.66511309525283835 ) ) ;
#7000=CIRCLE ( 'NONE', #13797, 8.000000000000000000 ) ;
#7001=ORIENTED_EDGE ( 'NONE', *, *, #13635, .F. ) ;
#7003=CARTESIAN_POINT ( 'NONE',  ( 25.06493225369642630, 19.99999999999999645, -5.669446505520304491 ) ) ;
#7004=AXIS2_PLACEMENT_3D ( 'NONE', #14053, #7310, #5803 ) ;
#7006=ORIENTED_EDGE ( 'NONE', *, *, #14421, .T. ) ;
#7008=CARTESIAN_POINT ( 'NONE',  ( 27.48361012698968864, 138.6227766016838245, -1.063447695028166570E-14 ) ) ;
#7009=ORIENTED_EDGE ( 'NONE', *, *, #11335, .F. ) ;
#7010=CARTESIAN_POINT ( 'NONE',  ( 26.21324911630662058, 153.1023373578139513, -27.31345131271288906 ) ) ;
#7013=CIRCLE ( 'NONE', #4756, 20.00000000000000355 ) ;
#7014=DIRECTION ( 'NONE',  ( -1.000000000000000000, 0.000000000000000000, 0.000000000000000000 ) ) ;
#7015=CARTESIAN_POINT ( 'NONE',  ( 37.44048204095823706, 195.6584727333608669, -22.61345334826514275 ) ) ;
#7016=DIRECTION ( 'NONE',  ( -1.000000000000000000, -6.938893903907228378E-16, -0.000000000000000000 ) ) ;
#7017=ADVANCED_FACE ( 'NONE', ( #6055 ), #8871, .F. ) ;
#7018=DIRECTION ( 'NONE',  ( -0.000000000000000000, -0.000000000000000000, 1.000000000000000000 ) ) ;
#7019=CARTESIAN_POINT ( 'NONE',  ( -43.00000000000000000, 134.2062027339443944, -25.00000000000000000 ) ) ;
#7021=CARTESIAN_POINT ( 'NONE',  ( 14.58358448378887928, 141.6717822189192191, -18.11319387340528309 ) ) ;
#7024=CARTESIAN_POINT ( 'NONE',  ( -40.00000000000000000, 20.00000000000000000, -30.00000000000000355 ) ) ;
#7025=CARTESIAN_POINT ( 'NONE',  ( -11.59473107857741425, 31.35552539902487723, -12.08231249604354574 ) ) ;
#7029=LINE ( 'NONE', #1298, #14262 ) ;
#7033=EDGE_LOOP ( 'NONE', ( #7670, #43, #15861, #702 ) ) ;
#7039=VECTOR ( 'NONE', #9818, 1000.000000000000000 ) ;
#7043=AXIS2_PLACEMENT_3D ( 'NONE', #8868, #6141, #8617 ) ;
#7046=DIRECTION ( 'NONE',  ( 1.000000000000000000, 0.000000000000000000, 0.000000000000000000 ) ) ;
#7049=CARTESIAN_POINT ( 'NONE',  ( -80.00000000000001421, 196.6227766016838245, -16.00000000000000000 ) ) ;
#7050=ORIENTED_EDGE ( 'NONE', *, *, #6527, .T. ) ;
#7056=VERTEX_POINT ( 'NONE', #8620 ) ;
#7057=CARTESIAN_POINT ( 'NONE',  ( 48.00000000000000711, 163.6227766016838530, -12.50000337241049309 ) ) ;
#7064=AXIS2_PLACEMENT_3D ( 'NONE', #12044, #8233, #9640 ) ;
#7065=PRODUCT_DEFINITION ( 'UNKNOWN', '', #16052, #5303 ) ;
#7066=DIRECTION ( 'NONE',  ( 0.000000000000000000, 0.000000000000000000, 1.000000000000000000 ) ) ;
#7068=EDGE_CURVE ( 'NONE', #11112, #15769, #4372, .T. ) ;
#7069=CIRCLE ( 'NONE', #7357, 20.00000000000000355 ) ;
#7070=DIRECTION ( 'NONE',  ( -1.000000000000000000, -0.000000000000000000, 0.000000000000000000 ) ) ;
#7072=CARTESIAN_POINT ( 'NONE',  ( 27.44407568426053246, 136.8394969516870958, -3.888888888888893725 ) ) ;
#7073=ORIENTED_EDGE ( 'NONE', *, *, #9529, .F. ) ;
#7075=CARTESIAN_POINT ( 'NONE',  ( 26.85584576128377066, 139.3465472469502231, -6.878002324459898453 ) ) ;
#7078=VERTEX_POINT ( 'NONE', #6144 ) ;
#7079=CARTESIAN_POINT ( 'NONE',  ( -82.99938094214050466, 191.4078883217828491, -28.87216486436161844 ) ) ;
#7082=CARTESIAN_POINT ( 'NONE',  ( -91.33974596215564645, 171.6227766016838245, 0.000000000000000000 ) ) ;
#7083=CARTESIAN_POINT ( 'NONE',  ( 27.48361012698968864, 138.6227766016838245, -1.063447695028166570E-14 ) ) ;
#7088=EDGE_LOOP ( 'NONE', ( #3058, #10316 ) ) ;
#7090=AXIS2_PLACEMENT_3D ( 'NONE', #2700, #14821, #12179 ) ;
#7092=ORIENTED_EDGE ( 'NONE', *, *, #1485, .T. ) ;
#7094=CARTESIAN_POINT ( 'NONE',  ( 49.99999999999998579, 163.6227766016838530, -15.00000337241049486 ) ) ;
#7097=EDGE_CURVE ( 'NONE', #13399, #8346, #7296, .T. ) ;
#7098=CARTESIAN_POINT ( 'NONE',  ( 37.43684327452984206, 197.7246901893026632, -20.20962120078073809 ) ) ;
#7103=CARTESIAN_POINT ( 'NONE',  ( -90.80384757729339640, 204.6227766016838245, 0.000000000000000000 ) ) ;
#7107=VERTEX_POINT ( 'NONE', #579 ) ;
#7109=CIRCLE ( 'NONE', #608, 12.00000000000001421 ) ;
#7110=CARTESIAN_POINT ( 'NONE',  ( -12.31336727611479631, 31.57746213708666971, -11.68681022658133806 ) ) ;
#7111=ORIENTED_EDGE ( 'NONE', *, *, #6843, .F. ) ;
#7112=EDGE_LOOP ( 'NONE', ( #1017, #1463 ) ) ;
#7115=EDGE_CURVE ( 'NONE', #14296, #14117, #15099, .T. ) ;
#7128=CARTESIAN_POINT ( 'NONE',  ( -74.50191221171618849, 199.0501964078081016, -21.74862058155255795 ) ) ;
#7129=CARTESIAN_POINT ( 'NONE',  ( -725.0000000000000000, 19.99999999999995737, -15.00000000000000000 ) ) ;
#7130=CARTESIAN_POINT ( 'NONE',  ( 24.94691999498327206, 20.00000000000000355, -22.32501294936691139 ) ) ;
#7131=DIRECTION ( 'NONE',  ( -1.000000000000000000, 0.000000000000000000, 0.000000000000000000 ) ) ;
#7141=CARTESIAN_POINT ( 'NONE',  ( 22.94847233519770668, 144.0220640066157785, -18.10843944793623805 ) ) ;
#7144=CARTESIAN_POINT ( 'NONE',  ( 30.00000000000000355, 196.6227766016838245, -35.00200000000000244 ) ) ;
#7145=CARTESIAN_POINT ( 'NONE',  ( 22.56235622051156042, 18.00000000000227018, -7.873592366086867855 ) ) ;
#7146=ORIENTED_EDGE ( 'NONE', *, *, #6432, .F. ) ;
#7148=CARTESIAN_POINT ( 'NONE',  ( -100.0000000000000000, 100.0000000000000142, -6.000000000000000000 ) ) ;
#7151=EDGE_CURVE ( 'NONE', #9019, #4348, #14208, .T. ) ;
#7152=PRODUCT_DEFINITION_SHAPE ( 'NONE', 'NONE',  #7065 ) ;
#7153=ADVANCED_FACE ( 'NONE', ( #4822 ), #4523, .T. ) ;
#7154=CARTESIAN_POINT ( 'NONE',  ( -7.379000772445021283, 18.00000000000000000, -25.00000000000000355 ) ) ;
#7155=ORIENTED_EDGE ( 'NONE', *, *, #4525, .T. ) ;
#7159=CARTESIAN_POINT ( 'NONE',  ( -84.02588075151039959, 192.1541050315148595, -28.34722919022667043 ) ) ;
#7164=FACE_OUTER_BOUND ( 'NONE', #4386, .T. ) ;
#7166=CARTESIAN_POINT ( 'NONE',  ( 6.134011831684049731, 144.1839557653416080, -18.33333333333335702 ) ) ;
#7167=FACE_BOUND ( 'NONE', #11236, .T. ) ;
#7168=EDGE_LOOP ( 'NONE', ( #2087, #14212, #11177, #4964 ) ) ;
#7170=CARTESIAN_POINT ( 'NONE',  ( 24.60025152864608700, 29.87271304632927027, -7.586598161752979408 ) ) ;
#7171=CARTESIAN_POINT ( 'NONE',  ( 27.44407568426044008, 138.8271129316868837, -3.666666666666658081 ) ) ;
#7175=VERTEX_POINT ( 'NONE', #1710 ) ;
#7176=CARTESIAN_POINT ( 'NONE',  ( 32.27956779150308364, 153.7735974263994194, -27.75644086540373934 ) ) ;
#7177=ADVANCED_FACE ( 'NONE', ( #2773 ), #8330, .T. ) ;
#7180=AXIS2_PLACEMENT_3D ( 'NONE', #7503, #12913, #7854 ) ;
#7183=DIRECTION ( 'NONE',  ( 0.000000000000000000, 0.000000000000000000, 1.000000000000000000 ) ) ;
#7184=CARTESIAN_POINT ( 'NONE',  ( -74.72505082391214160, 141.2912748254776147, -13.00000000000000000 ) ) ;
#7185=EDGE_LOOP ( 'NONE', ( #201, #14566, #1606, #11825 ) ) ;
#7192=ORIENTED_EDGE ( 'NONE', *, *, #8349, .T. ) ;
#7195=AXIS2_PLACEMENT_3D ( 'NONE', #15246, #8696, #3122 ) ;
#7198=ORIENTED_EDGE ( 'NONE', *, *, #5382, .F. ) ;
#7199=CYLINDRICAL_SURFACE ( 'NONE', #10769, 6.000000000000005329 ) ;
#7205=AXIS2_PLACEMENT_3D ( 'NONE', #10530, #14260, #9031 ) ;
#7207=DIRECTION ( 'NONE',  ( 0.000000000000000000, 1.000000000000000000, 0.000000000000000000 ) ) ;
#7214=DIRECTION ( 'NONE',  ( 0.000000000000000000, 0.8660254037844413721, 0.4999999999999952816 ) ) ;
#7216=ORIENTED_EDGE ( 'NONE', *, *, #9430, .T. ) ;
#7218=ORIENTED_EDGE ( 'NONE', *, *, #15267, .T. ) ;
#7219=CARTESIAN_POINT ( 'NONE',  ( -15.00000000000002132, 90.00000000000000000, -4.999999999999999112 ) ) ;
#7222=CIRCLE ( 'NONE', #15420, 12.00000000000000000 ) ;
#7233=CARTESIAN_POINT ( 'NONE',  ( -5.000000000000004441, 171.6227766016838245, 0.000000000000000000 ) ) ;
#7234=CARTESIAN_POINT ( 'NONE',  ( -70.00000000000000000, 204.6227766016838245, 2.020667218593133100E-15 ) ) ;
#7238=CARTESIAN_POINT ( 'NONE',  ( -23.00000000000000000, 122.0000000000000284, -15.00000000000000000 ) ) ;
#7242=CARTESIAN_POINT ( 'NONE',  ( 0.000000000000000000, 18.00000000000000355, 0.000000000000000000 ) ) ;
#7247=VECTOR ( 'NONE', #8433, 1000.000000000000000 ) ;
#7248=DIRECTION ( 'NONE',  ( -1.000000000000000000, -0.000000000000000000, -0.000000000000000000 ) ) ;
#7249=EDGE_CURVE ( 'NONE', #4808, #12895, #6849, .T. ) ;
#7258=CARTESIAN_POINT ( 'NONE',  ( 31.20232444246483894, 19.99999999999999645, -16.65183244246150451 ) ) ;
#7264=DIRECTION ( 'NONE',  ( 0.000000000000000000, 0.000000000000000000, 1.000000000000000000 ) ) ;
#7266=EDGE_LOOP ( 'NONE', ( #13404, #7192, #905, #7399, #11081 ) ) ;
#7269=ADVANCED_FACE ( 'NONE', ( #16324 ), #289, .T. ) ;
#7270=DIRECTION ( 'NONE',  ( 0.000000000000000000, 0.000000000000000000, -1.000000000000000000 ) ) ;
#7271=PLANE ( 'NONE',  #14004 ) ;
#7272=DIRECTION ( 'NONE',  ( 0.000000000000000000, -1.000000000000000000, 0.000000000000000000 ) ) ;
#7275=CARTESIAN_POINT ( 'NONE',  ( -72.79003115184357853, 144.4916047800714693, -18.80562413441370850 ) ) ;
#7276=ORIENTED_EDGE ( 'NONE', *, *, #14691, .T. ) ;
#7279=ADVANCED_FACE ( 'NONE', ( #5513, #4192 ), #5343, .F. ) ;
#7282=DIRECTION ( 'NONE',  ( 1.000000000000000000, 0.000000000000000000, 0.000000000000000000 ) ) ;
#7283=ORIENTED_EDGE ( 'NONE', *, *, #5752, .F. ) ;
#7287=AXIS2_PLACEMENT_3D ( 'NONE', #5258, #7999, #17486 ) ;
#7292=CARTESIAN_POINT ( 'NONE',  ( 196.0000000000000000, 183.6227766016837961, -5.571800142134975431 ) ) ;
#7296=LINE ( 'NONE', #12701, #10573 ) ;
#7299=AXIS2_PLACEMENT_3D ( 'NONE', #8806, #14210, #6146 ) ;
#7300=PLANE ( 'NONE',  #26 ) ;
#7304=FACE_BOUND ( 'NONE', #5033, .T. ) ;
#7305=EDGE_LOOP ( 'NONE', ( #11526, #1887, #1913, #6548 ) ) ;
#7307=ORIENTED_EDGE ( 'NONE', *, *, #9201, .T. ) ;
#7310=DIRECTION ( 'NONE',  ( -0.000000000000000000, -0.000000000000000000, -1.000000000000000000 ) ) ;
#7320=CARTESIAN_POINT ( 'NONE',  ( -85.00000000000002842, 196.6227766016838245, -12.99999999999999822 ) ) ;
#7325=CARTESIAN_POINT ( 'NONE',  ( -100.0000000000000000, 143.0439382767972347, -16.49999999999984368 ) ) ;
#7326=CARTESIAN_POINT ( 'NONE',  ( -7.379000772444995526, 20.00000000000000000, -25.00000000000000000 ) ) ;
#7330=AXIS2_PLACEMENT_3D ( 'NONE', #16511, #4380, #11098 ) ;
#7331=CARTESIAN_POINT ( 'NONE',  ( -21.99999999999998579, 10.00000000000000000, -16.00000000000000000 ) ) ;
#7332=EDGE_LOOP ( 'NONE', ( #10504, #8442, #2175, #3865, #15750, #12956, #12820, #1797 ) ) ;
#7334=ORIENTED_EDGE ( 'NONE', *, *, #10599, .F. ) ;
#7339=CYLINDRICAL_SURFACE ( 'NONE', #14942, 6.000000000000005329 ) ;
#7342=AXIS2_PLACEMENT_3D ( 'NONE', #13024, #10263, #4618 ) ;
#7343=CARTESIAN_POINT ( 'NONE',  ( -18.25212770525997286, 32.30769230769230660, -4.999999999999999112 ) ) ;
#7346=CARTESIAN_POINT ( 'NONE',  ( 49.99999999999998579, 171.6227766016838245, -12.50000337241049131 ) ) ;
#7349=EDGE_LOOP ( 'NONE', ( #11455, #2568, #8921, #16429 ) ) ;
#7350=ORIENTED_EDGE ( 'NONE', *, *, #7473, .F. ) ;
#7351=DIRECTION ( 'NONE',  ( -1.000000000000000000, 0.000000000000000000, 0.000000000000000000 ) ) ;
#7353=CARTESIAN_POINT ( 'NONE',  ( 17.57170338634705331, 142.7189882356449857, -15.92841986281182187 ) ) ;
#7354=EDGE_LOOP ( 'NONE', ( #7998, #7396, #2720, #11242, #1725 ) ) ;
#7355=EDGE_CURVE ( 'NONE', #668, #12793, #8598, .T. ) ;
#7356=CARTESIAN_POINT ( 'NONE',  ( -70.00000000000000000, 171.6227766016838245, 0.000000000000000000 ) ) ;
#7357=AXIS2_PLACEMENT_3D ( 'NONE', #14605, #17173, #7695 ) ;
#7358=CARTESIAN_POINT ( 'NONE',  ( 6.134011831684059501, 144.1839557653415795, -18.33333333333333215 ) ) ;
#7363=CARTESIAN_POINT ( 'NONE',  ( -34.99999999999999289, 130.0000000000000000, -15.00000000000000000 ) ) ;
#7366=VECTOR ( 'NONE', #16634, 1000.000000000000000 ) ;
#7369=AXIS2_PLACEMENT_3D ( 'NONE', #7478, #498, #10227 ) ;
#7372=FACE_BOUND ( 'NONE', #3259, .T. ) ;
#7373=B_SPLINE_CURVE_WITH_KNOTS ( 'NONE', 3,
 ( #17403, #5273, #13607, #16085 ),
 .UNSPECIFIED., .F., .F.,
 ( 4, 4 ),
 ( 0.000000000000000000, 0.0004807729677303993116 ),
 .UNSPECIFIED. ) ;
#7374=VERTEX_POINT ( 'NONE', #5770 ) ;
#7377=ORIENTED_EDGE ( 'NONE', *, *, #6808, .T. ) ;
#7380=VECTOR ( 'NONE', #4569, 1000.000000000000000 ) ;
#7384=DIRECTION ( 'NONE',  ( 2.312964634635742464E-16, 0.000000000000000000, 1.000000000000000000 ) ) ;
#7391=DIRECTION ( 'NONE',  ( 0.000000000000000000, 0.000000000000000000, 1.000000000000000000 ) ) ;
#7395=CARTESIAN_POINT ( 'NONE',  ( -22.79696676584442017, 19.99999999999999645, -18.34105320469109301 ) ) ;
#7396=ORIENTED_EDGE ( 'NONE', *, *, #16739, .T. ) ;
#7397=DIRECTION ( 'NONE',  ( -0.000000000000000000, -0.000000000000000000, -1.000000000000000000 ) ) ;
#7398=FACE_BOUND ( 'NONE', #11710, .T. ) ;
#7399=ORIENTED_EDGE ( 'NONE', *, *, #8887, .F. ) ;
#7400=ORIENTED_EDGE ( 'NONE', *, *, #1865, .T. ) ;
#7401=ORIENTED_EDGE ( 'NONE', *, *, #8795, .F. ) ;
#7407=CARTESIAN_POINT ( 'NONE',  ( 6.134011831684049731, 134.2062027339443944, -13.00000000000000000 ) ) ;
#7408=VERTEX_POINT ( 'NONE', #726 ) ;
#7410=DIRECTION ( 'NONE',  ( 2.312964634635742464E-16, 0.000000000000000000, 1.000000000000000000 ) ) ;
#7411=CARTESIAN_POINT ( 'NONE',  ( -25.00000000000002132, 120.0000000000000284, -5.000000000000023093 ) ) ;
#7412=CARTESIAN_POINT ( 'NONE',  ( -7.379000772444995526, 20.00000000000000355, -15.00000000000000178 ) ) ;
#7414=EDGE_CURVE ( 'NONE', #3416, #15255, #8610, .T. ) ;
#7418=VERTEX_POINT ( 'NONE', #3119 ) ;
#7421=CARTESIAN_POINT ( 'NONE',  ( 13.21952030233119046, 128.8713892059273860, -10.07325499884888664 ) ) ;
#7423=DIRECTION ( 'NONE',  ( 1.000000000000000000, 0.000000000000000000, 0.000000000000000000 ) ) ;
#7427=ORIENTED_EDGE ( 'NONE', *, *, #4947, .F. ) ;
#7432=CARTESIAN_POINT ( 'NONE',  ( 21.08563699167523353, 19.99999999999999645, -13.01331479026599602 ) ) ;
#7433=CARTESIAN_POINT ( 'NONE',  ( 16.17028938446068764, 143.0439382767918346, -16.49999999999050360 ) ) ;
#7434=ORIENTED_EDGE ( 'NONE', *, *, #680, .F. ) ;
#7435=FACE_OUTER_BOUND ( 'NONE', #3792, .T. ) ;
#7437=ORIENTED_EDGE ( 'NONE', *, *, #10059, .T. ) ;
#7438=PRODUCT ( 'MirrorLeft Housing Shell', 'MirrorLeft Housing Shell', '', ( #14820 ) ) ;
#7441=DIRECTION ( 'NONE',  ( 1.000000000000000000, 0.000000000000000000, 0.000000000000000000 ) ) ;
#7444=DIRECTION ( 'NONE',  ( 1.000000000000000000, 0.000000000000000000, -0.000000000000000000 ) ) ;
#7445=ORIENTED_EDGE ( 'NONE', *, *, #10983, .T. ) ;
#7449=DIRECTION ( 'NONE',  ( 0.000000000000000000, 1.000000000000000000, 0.000000000000000000 ) ) ;
#7461=EDGE_CURVE ( 'NONE', #7719, #2257, #406, .T. ) ;
#7463=DIRECTION ( 'NONE',  ( 0.000000000000000000, 0.000000000000000000, 1.000000000000000000 ) ) ;
#7465=ORIENTED_EDGE ( 'NONE', *, *, #10774, .T. ) ;
#7468=AXIS2_PLACEMENT_3D ( 'NONE', #835, #16862, #13948 ) ;
#7470=VECTOR ( 'NONE', #13856, 1000.000000000000000 ) ;
#7472=VERTEX_POINT ( 'NONE', #6035 ) ;
#7473=EDGE_CURVE ( 'NONE', #13322, #14130, #11428, .T. ) ;
#7474=VERTEX_POINT ( 'NONE', #12585 ) ;
#7475=CARTESIAN_POINT ( 'NONE',  ( 30.00000000000000355, 196.6227766016838245, -35.00000000000000000 ) ) ;
#7476=ORIENTED_EDGE ( 'NONE', *, *, #5920, .T. ) ;
#7478=CARTESIAN_POINT ( 'NONE',  ( 17.00000000000000000, 171.6227766016838245, 0.000000000000000000 ) ) ;
#7480=CARTESIAN_POINT ( 'NONE',  ( 48.00000000000000711, 187.6227766016837961, -10.00000337241049309 ) ) ;
#7482=CIRCLE ( 'NONE', #13135, 5.000000000000000888 ) ;
#7484=ORIENTED_EDGE ( 'NONE', *, *, #15006, .F. ) ;
#7486=DIRECTION ( 'NONE',  ( 0.000000000000000000, 0.000000000000000000, 1.000000000000000000 ) ) ;
#7488=CARTESIAN_POINT ( 'NONE',  ( -23.66837786580496328, 19.99999999999999645, -17.32703391567687135 ) ) ;
#7490=EDGE_CURVE ( 'NONE', #16973, #14936, #5860, .T. ) ;
#7491=ADVANCED_FACE ( 'NONE', ( #16927 ), #4799, .T. ) ;
#7496=CARTESIAN_POINT ( 'NONE',  ( -68.00000000000000000, 206.6227766016838245, 2.143131898507868248E-15 ) ) ;
#7497=AXIS2_PLACEMENT_3D ( 'NONE', #2174, #1016, #3592 ) ;
#7498=ORIENTED_EDGE ( 'NONE', *, *, #4038, .F. ) ;
#7500=CARTESIAN_POINT ( 'NONE',  ( -86.00000000000002842, 146.6227766016838245, -16.00000000000000000 ) ) ;
#7503=CARTESIAN_POINT ( 'NONE',  ( -40.00000000000000000, 20.00000000000000000, -30.00000000000000355 ) ) ;
#7504=VECTOR ( 'NONE', #13238, 1000.000000000000000 ) ;
#7505=ORIENTED_EDGE ( 'NONE', *, *, #2678, .F. ) ;
#7506=DIRECTION ( 'NONE',  ( 0.000000000000000000, 0.000000000000000000, -1.000000000000000000 ) ) ;
#7508=VECTOR ( 'NONE', #13077, 1000.000000000000000 ) ;
#7509=DIRECTION ( 'NONE',  ( 1.000000000000000000, 0.000000000000000000, -0.000000000000000000 ) ) ;
#7510=CARTESIAN_POINT ( 'NONE',  ( 29.74498994719569467, 202.6234830987602038, -16.24672887513766639 ) ) ;
#7511=ORIENTED_EDGE ( 'NONE', *, *, #3064, .T. ) ;
#7513=CARTESIAN_POINT ( 'NONE',  ( 18.45742352454476887, 29.95282391178955095, -14.36414658362611974 ) ) ;
#7514=CARTESIAN_POINT ( 'NONE',  ( 27.42718951882975631, 138.9142741377072525, -4.446260193316556197 ) ) ;
#7515=VERTEX_POINT ( 'NONE', #11864 ) ;
#7519=AXIS2_PLACEMENT_3D ( 'NONE', #9222, #14372, #12957 ) ;
#7522=FACE_BOUND ( 'NONE', #11451, .T. ) ;
#7523=ADVANCED_FACE ( 'NONE', ( #5053 ), #9117, .F. ) ;
#7525=EDGE_CURVE ( 'NONE', #4295, #9729, #6312, .T. ) ;
#7531=LINE ( 'NONE', #11770, #1273 ) ;
#7534=DIRECTION ( 'NONE',  ( 0.000000000000000000, -0.8660254037844413721, -0.4999999999999953371 ) ) ;
#7539=CIRCLE ( 'NONE', #15738, 5.999999999999998224 ) ;
#7542=DIRECTION ( 'NONE',  ( -1.000000000000000000, -0.000000000000000000, -0.000000000000000000 ) ) ;
#7544=ORIENTED_EDGE ( 'NONE', *, *, #8256, .T. ) ;
#7545=EDGE_CURVE ( 'NONE', #919, #6279, #815, .T. ) ;
#7549=CARTESIAN_POINT ( 'NONE',  ( 32.79368516360896280, 189.6403081819231886, -27.64877209012309223 ) ) ;
#7550=CARTESIAN_POINT ( 'NONE',  ( -11.03695849842137910, 30.81357570984703642, -14.42948753805835871 ) ) ;
#7553=VERTEX_POINT ( 'NONE', #13030 ) ;
#7555=CARTESIAN_POINT ( 'NONE',  ( -20.85266279178580362, 19.99999999999999645, -20.15433268689462665 ) ) ;
#7558=DIRECTION ( 'NONE',  ( 1.000000000000000000, 0.000000000000000000, 0.000000000000000000 ) ) ;
#7559=ORIENTED_EDGE ( 'NONE', *, *, #5476, .F. ) ;
#7563=CARTESIAN_POINT ( 'NONE',  ( 16.24385689529520604, 136.8350826111700655, -4.682368943704262598 ) ) ;
#7567=ORIENTED_EDGE ( 'NONE', *, *, #9265, .F. ) ;
#7576=CARTESIAN_POINT ( 'NONE',  ( 49.99999999999998579, 171.6227766016838245, -12.50000337241049131 ) ) ;
#7579=CARTESIAN_POINT ( 'NONE',  ( -15.33310217279680288, 19.99999999999999645, -4.999999999999999112 ) ) ;
#7583=VERTEX_POINT ( 'NONE', #15670 ) ;
#7585=FACE_BOUND ( 'NONE', #14911, .T. ) ;
#7586=CIRCLE ( 'NONE', #14381, 30.00000000000000000 ) ;
#7588=ORIENTED_EDGE ( 'NONE', *, *, #9562, .F. ) ;
#7599=DIRECTION ( 'NONE',  ( 0.000000000000000000, 0.8660254037844413721, 0.4999999999999952816 ) ) ;
#7601=EDGE_LOOP ( 'NONE', ( #14739, #6534, #15227, #4634 ) ) ;
#7602=EDGE_LOOP ( 'NONE', ( #1275, #15487, #1713, #7768 ) ) ;
#7603=CARTESIAN_POINT ( 'NONE',  ( 17.69056612348262192, 19.99999999999999645, -14.65191630173004711 ) ) ;
#7604=DIRECTION ( 'NONE',  ( 0.000000000000000000, 0.000000000000000000, 1.000000000000000000 ) ) ;
#7606=DIRECTION ( 'NONE',  ( 1.000000000000000000, 0.000000000000000000, 0.000000000000000000 ) ) ;
#7609=ORIENTED_EDGE ( 'NONE', *, *, #2631, .F. ) ;
#7611=CARTESIAN_POINT ( 'NONE',  ( 30.00000000000000355, 196.6227766016838245, -16.00000000000000000 ) ) ;
#7613=CARTESIAN_POINT ( 'NONE',  ( 196.0000000000000000, 175.6227766016838245, -5.571800142134975431 ) ) ;
#7616=DIRECTION ( 'NONE',  ( 0.000000000000000000, 0.000000000000000000, -1.000000000000000000 ) ) ;
#7617=CARTESIAN_POINT ( 'NONE',  ( 30.54126313378810664, 140.6457587561385196, -16.29186131275297811 ) ) ;
#7619=DIRECTION ( 'NONE',  ( 0.000000000000000000, -0.4999999999999952816, 0.8660254037844413721 ) ) ;
#7620=AXIS2_PLACEMENT_3D ( 'NONE', #10332, #2198, #7599 ) ;
#7624=CARTESIAN_POINT ( 'NONE',  ( 24.00000000000000000, 146.6227766016838245, -16.00000000000000000 ) ) ;
#7626=ORIENTED_EDGE ( 'NONE', *, *, #575, .T. ) ;
#7631=AXIS2_PLACEMENT_3D ( 'NONE', #5539, #1386, #2799 ) ;
#7633=AXIS2_PLACEMENT_3D ( 'NONE', #12108, #10779, #4058 ) ;
#7634=CARTESIAN_POINT ( 'NONE',  ( -68.00000000000000000, 171.6227766016838245, 0.000000000000000000 ) ) ;
#7636=PLANE ( 'NONE',  #8231 ) ;
#7637=CARTESIAN_POINT ( 'NONE',  ( -16.30611068361784532, 32.76923076923076650, -4.999999999999998224 ) ) ;
#7638=ORIENTED_EDGE ( 'NONE', *, *, #9868, .T. ) ;
#7639=FACE_OUTER_BOUND ( 'NONE', #7305, .T. ) ;
#7640=ORIENTED_EDGE ( 'NONE', *, *, #16047, .F. ) ;
#7641=CARTESIAN_POINT ( 'NONE',  ( 24.44329345585415325, 194.3322840258869064, -26.63593000238176955 ) ) ;
#7647=ORIENTED_EDGE ( 'NONE', *, *, #4565, .T. ) ;
#7650=CIRCLE ( 'NONE', #12189, 2.499999999999998668 ) ;
#7651=CARTESIAN_POINT ( 'NONE',  ( -81.13499951972124791, 154.0589040539455539, -27.93804624201381515 ) ) ;
#7652=ORIENTED_EDGE ( 'NONE', *, *, #4400, .F. ) ;
#7656=CARTESIAN_POINT ( 'NONE',  ( 24.22132560812392299, 148.2463666031633807, -26.04982723689807500 ) ) ;
#7657=VECTOR ( 'NONE', #13946, 1000.000000000000000 ) ;
#7660=ORIENTED_EDGE ( 'NONE', *, *, #17290, .F. ) ;
#7662=CARTESIAN_POINT ( 'NONE',  ( 17.21487247493544714, 29.96934980803111159, -14.74175109707249831 ) ) ;
#7663=CARTESIAN_POINT ( 'NONE',  ( -20.49999999999998224, 10.00000000000000000, -28.00000000000000355 ) ) ;
#7664=ADVANCED_FACE ( 'NONE', ( #11953 ), #5227, .F. ) ;
#7666=ORIENTED_EDGE ( 'NONE', *, *, #720, .F. ) ;
#7667=CARTESIAN_POINT ( 'NONE',  ( -48.00000000000000000, 171.6227766016838245, -20.00000000000000355 ) ) ;
#7668=VECTOR ( 'NONE', #5432, 1000.000000000000000 ) ;
#7670=ORIENTED_EDGE ( 'NONE', *, *, #5964, .F. ) ;
#7672=DIRECTION ( 'NONE',  ( 0.000000000000000000, 0.000000000000000000, 1.000000000000000000 ) ) ;
#7675=CARTESIAN_POINT ( 'NONE',  ( 17.01529014380724192, 17.99999999999885958, -12.76845467807931733 ) ) ;
#7677=CARTESIAN_POINT ( 'NONE',  ( 6.803110712587624676, 134.0269829078799262, -12.98040381008119759 ) ) ;
#7679=DIRECTION ( 'NONE',  ( -1.000000000000000000, 0.000000000000000000, 0.000000000000000000 ) ) ;
#7681=EDGE_CURVE ( 'NONE', #3017, #1185, #11437, .T. ) ;
#7682=DIRECTION ( 'NONE',  ( -1.000000000000000000, 0.000000000000000000, 0.000000000000000000 ) ) ;
#7684=CARTESIAN_POINT ( 'NONE',  ( 24.00000000000000000, 196.6227766016838245, -24.49489742783178770 ) ) ;
#7685=ORIENTED_EDGE ( 'NONE', *, *, #3936, .T. ) ;
#7686=ORIENTED_EDGE ( 'NONE', *, *, #3503, .F. ) ;
#7687=CARTESIAN_POINT ( 'NONE',  ( 20.11141720500585350, 19.99999999999999645, -24.32074799214527516 ) ) ;
#7688=CARTESIAN_POINT ( 'NONE',  ( 40.00000000000000711, 196.6227766016838245, 0.000000000000000000 ) ) ;
#7689=EDGE_LOOP ( 'NONE', ( #1272, #16118, #5776, #10557, #9882, #10249, #800, #6290, #3618, #5462, #6200, #13293, #7350, #10544 ) ) ;
#7690=CARTESIAN_POINT ( 'NONE',  ( -100.0000000000000000, 136.6227766016838245, 0.000000000000000000 ) ) ;
#7691=EDGE_CURVE ( 'NONE', #5007, #13962, #2753, .T. ) ;
#7692=CARTESIAN_POINT ( 'NONE',  ( 14.46714703242257904, 138.5709836085849531, -4.391619799165513705 ) ) ;
#7693=EDGE_CURVE ( 'NONE', #9063, #1055, #9387, .T. ) ;
#7695=DIRECTION ( 'NONE',  ( 0.000000000000000000, 0.000000000000000000, 1.000000000000000000 ) ) ;
#7700=B_SPLINE_CURVE_WITH_KNOTS ( 'NONE', 3,
 ( #1915, #14221, #1826, #4837, #7141, #14143, #4659, #10044, #2083, #15458 ),
 .UNSPECIFIED., .F., .F.,
 ( 4, 2, 2, 2, 4 ),
 ( 0.03775390620236026423, 0.04033669301524706735, 0.04291947982813386353, 0.04550226664102066665, 0.04808505345390746977 ),
 .UNSPECIFIED. ) ;
#7709=DIRECTION ( 'NONE',  ( -1.000000000000000000, -0.000000000000000000, 0.000000000000000000 ) ) ;
#7714=CARTESIAN_POINT ( 'NONE',  ( -80.00000000000002842, 146.6227766016838245, 0.000000000000000000 ) ) ;
#7715=LINE ( 'NONE', #17292, #16940 ) ;
#7716=CARTESIAN_POINT ( 'NONE',  ( -12.61248932541308676, 31.15232071419451643, -13.80069170922183375 ) ) ;
#7717=ADVANCED_FACE ( 'NONE', ( #175, #12221 ), #1429, .T. ) ;
#7718=CARTESIAN_POINT ( 'NONE',  ( -10.50630597522742171, 31.01369813559846378, -12.50559288035636563 ) ) ;
#7719=VERTEX_POINT ( 'NONE', #6900 ) ;
#7722=CARTESIAN_POINT ( 'NONE',  ( 29.09601211296537571, 190.6868548533384455, -29.35237411376976269 ) ) ;
#7723=DIRECTION ( 'NONE',  ( 0.000000000000000000, 0.000000000000000000, 1.000000000000000000 ) ) ;
#7726=ORIENTED_EDGE ( 'NONE', *, *, #14841, .F. ) ;
#7728=CARTESIAN_POINT ( 'NONE',  ( -87.25061104762463060, 148.5880153409831905, -23.63707964515040416 ) ) ;
#7729=ORIENTED_EDGE ( 'NONE', *, *, #14504, .T. ) ;
#7733=CARTESIAN_POINT ( 'NONE',  ( 28.19759474139298305, 152.3499437555877876, -29.21584945930381494 ) ) ;
#7734=EDGE_CURVE ( 'NONE', #16797, #3065, #11870, .T. ) ;
#7736=EDGE_CURVE ( 'NONE', #14104, #11995, #6213, .T. ) ;
#7741=DIRECTION ( 'NONE',  ( 1.000000000000000000, 0.000000000000000000, 0.000000000000000000 ) ) ;
#7743=CARTESIAN_POINT ( 'NONE',  ( -15.00000000000002665, 130.0000000000000000, -15.00000000000000000 ) ) ;
#7744=DIRECTION ( 'NONE',  ( 0.000000000000000000, 0.000000000000000000, -1.000000000000000000 ) ) ;
#7750=CARTESIAN_POINT ( 'NONE',  ( -23.00000000000000000, 120.0000000000000426, -15.00000000000000000 ) ) ;
#7751=AXIS2_PLACEMENT_3D ( 'NONE', #6209, #9033, #7616 ) ;
#7752=AXIS2_PLACEMENT_3D ( 'NONE', #10677, #9348, #15010 ) ;
#7753=VERTEX_POINT ( 'NONE', #5415 ) ;
#7756=CARTESIAN_POINT ( 'NONE',  ( 15.97392895077415531, 29.97895215653467815, -12.94942366938410139 ) ) ;
#7757=CARTESIAN_POINT ( 'NONE',  ( -82.59785185926696727, 141.2103550623191381, -17.32402235562967618 ) ) ;
#7759=ORIENTED_EDGE ( 'NONE', *, *, #2696, .T. ) ;
#7761=DIRECTION ( 'NONE',  ( -1.000000000000000000, 0.000000000000000000, 0.000000000000000000 ) ) ;
#7765=CIRCLE ( 'NONE', #16832, 5.000000000000000888 ) ;
#7768=ORIENTED_EDGE ( 'NONE', *, *, #8316, .T. ) ;
#7769=CARTESIAN_POINT ( 'NONE',  ( 12.56741672263968290, 142.0153054307823481, -18.66563201629009328 ) ) ;
#7770=ORIENTED_EDGE ( 'NONE', *, *, #2304, .T. ) ;
#7772=CARTESIAN_POINT ( 'NONE',  ( 12.31199832339570577, 129.9194306174879046, -10.85217099066659685 ) ) ;
#7778=CARTESIAN_POINT ( 'NONE',  ( -87.50000000000004263, 196.6227766016838245, -21.54065922853802562 ) ) ;
#7783=CIRCLE ( 'NONE', #1290, 5.000000000000018652 ) ;
#7784=CARTESIAN_POINT ( 'NONE',  ( 196.0000000000000000, 151.6227766016839098, -5.571800142134973655 ) ) ;
#7786=CARTESIAN_POINT ( 'NONE',  ( 33.16115143954747424, 141.5060039278119177, -17.83622402891603187 ) ) ;
#7789=ORIENTED_EDGE ( 'NONE', *, *, #15984, .T. ) ;
#7792=AXIS2_PLACEMENT_3D ( 'NONE', #11445, #16943, #3314 ) ;
#7793=B_SPLINE_CURVE_WITH_KNOTS ( 'NONE', 3,
 ( #16171, #5531, #12258, #15079, #3044, #6942, #14824, #130, #9505, #2956, #8092, #12347, #8446, #13508, #13598, #15000, #8269, #221, #1468, #12439, #10922, #1639, #13770 ),
 .UNSPECIFIED., .F., .F.,
 ( 4, 2, 2, 2, 2, 2, 2, 2, 1, 2, 2, 4 ),
 ( 0.000000000000000000, 0.001562580732212274365, 0.002343871098318411547, 0.003125161464424548730, 0.004687742196636830901, 0.006250322928849113939, 0.007812903661061397845, 0.008594194027167533292, 0.009375484393273670475, 0.01015677475937980939, 0.01093806512548594484, 0.01250064585769823135 ),
 .UNSPECIFIED. ) ;
#7795=AXIS2_PLACEMENT_3D ( 'NONE', #5169, #17380, #11798 ) ;
#7797=DIRECTION ( 'NONE',  ( -1.000000000000000000, 0.000000000000000000, 0.000000000000000000 ) ) ;
#7799=EDGE_LOOP ( 'NONE', ( #4092, #7626, #2755, #16409 ) ) ;
#7800=PLANE ( 'NONE',  #5364 ) ;
#7803=DIRECTION ( 'NONE',  ( 0.000000000000000000, 0.000000000000000000, 1.000000000000000000 ) ) ;
#7804=TOROIDAL_SURFACE ( 'NONE', #1025, 240.0000000000000000, 8.000000000000000000 ) ;
#7806=CARTESIAN_POINT ( 'NONE',  ( 25.73052444394193472, 190.4340272497385058, -27.11642929875283059 ) ) ;
#7809=CIRCLE ( 'NONE', #8667, 2.499999999999998668 ) ;
#7810=CARTESIAN_POINT ( 'NONE',  ( -12.22383789047832181, 17.99999999999768363, -8.612907111650555336 ) ) ;
#7811=EDGE_CURVE ( 'NONE', #7814, #2789, #9554, .T. ) ;
#7812=ADVANCED_FACE ( 'NONE', ( #12394 ), #2835, .T. ) ;
#7813=VECTOR ( 'NONE', #14070, 1000.000000000000000 ) ;
#7814=VERTEX_POINT ( 'NONE', #10972 ) ;
#7815=LINE ( 'NONE', #14462, #5034 ) ;
#7816=ORIENTED_EDGE ( 'NONE', *, *, #15693, .T. ) ;
#7817=CARTESIAN_POINT ( 'NONE',  ( 35.61370932537138856, 194.4974200864254783, -26.49149599578360181 ) ) ;
#7819=ORIENTED_EDGE ( 'NONE', *, *, #4273, .T. ) ;
#7820=ORIENTED_EDGE ( 'NONE', *, *, #15767, .F. ) ;
#7821=ORIENTED_EDGE ( 'NONE', *, *, #5423, .T. ) ;
#7824=CARTESIAN_POINT ( 'NONE',  ( -74.37944869002585335, 151.5947363889490305, -26.22852547856965089 ) ) ;
#7826=VERTEX_POINT ( 'NONE', #10719 ) ;
#7827=CARTESIAN_POINT ( 'NONE',  ( 15.56337975240373162, 125.2134999403455851, -5.000000000000083489 ) ) ;
#7828=DIRECTION ( 'NONE',  ( -0.000000000000000000, -0.000000000000000000, -1.000000000000000000 ) ) ;
#7829=CARTESIAN_POINT ( 'NONE',  ( 31.77343803125589616, 152.3723237521624014, -29.23070922465767296 ) ) ;
#7831=CARTESIAN_POINT ( 'NONE',  ( 27.99999999999998224, 9.999999999999998224, -16.00000000000000000 ) ) ;
#7834=LINE ( 'NONE', #1019, #16545 ) ;
#7843=EDGE_CURVE ( 'NONE', #9042, #10642, #15690, .T. ) ;
#7850=AXIS2_PLACEMENT_3D ( 'NONE', #3410, #12871, #17112 ) ;
#7852=CARTESIAN_POINT ( 'NONE',  ( -15.00000000000001421, 130.0000000000000000, -13.00000000000000000 ) ) ;
#7853=DIRECTION ( 'NONE',  ( 0.000000000000000000, 0.000000000000000000, 1.000000000000000000 ) ) ;
#7854=DIRECTION ( 'NONE',  ( -1.000000000000000000, 0.000000000000000000, 8.673617379884037937E-17 ) ) ;
#7860=ORIENTED_EDGE ( 'NONE', *, *, #14504, .F. ) ;
#7863=CARTESIAN_POINT ( 'NONE',  ( 10.15450428991780285, 132.7081580017661224, -14.27405243007192581 ) ) ;
#7865=EDGE_CURVE ( 'NONE', #489, #4595, #9819, .T. ) ;
#7868=CARTESIAN_POINT ( 'NONE',  ( -85.04057431567690628, 149.8830506427268290, -27.43035542581613129 ) ) ;
#7869=EDGE_CURVE ( 'NONE', #10091, #3188, #3099, .T. ) ;
#7870=CARTESIAN_POINT ( 'NONE',  ( 19.90854668962690255, 142.0789032940274410, -14.70609183182490298 ) ) ;
#7875=CIRCLE ( 'NONE', #251, 2.500000000000002220 ) ;
#7877=CARTESIAN_POINT ( 'NONE',  ( 39.99999999999998579, 4.000000000000000000, -33.00000000000000711 ) ) ;
#7878=CIRCLE ( 'NONE', #14126, 5.000000000000000888 ) ;
#7880=CARTESIAN_POINT ( 'NONE',  ( 22.73076297281406255, 29.84603606043824442, -6.815711530131156159 ) ) ;
#7886=CARTESIAN_POINT ( 'NONE',  ( 14.80502546477524817, 129.0472650296936479, -11.28997929065621797 ) ) ;
#7887=CARTESIAN_POINT ( 'NONE',  ( -23.65835920965562877, 20.00000000000000000, -17.33937328557894020 ) ) ;
#7888=EDGE_LOOP ( 'NONE', ( #4492, #11707, #12824, #8526 ) ) ;
#7889=EDGE_CURVE ( 'NONE', #12193, #7826, #16687, .T. ) ;
#7892=DIRECTION ( 'NONE',  ( 1.000000000000000000, 0.000000000000000000, 0.000000000000000000 ) ) ;
#7893=AXIS2_PLACEMENT_3D ( 'NONE', #3918, #9303, #17456 ) ;
#7894=VERTEX_POINT ( 'NONE', #11498 ) ;
#7896=AXIS2_PLACEMENT_3D ( 'NONE', #7292, #10116, #15605 ) ;
#7898=VERTEX_POINT ( 'NONE', #8672 ) ;
#7899=CARTESIAN_POINT ( 'NONE',  ( -725.0000000000000000, 19.99999999999995737, -15.00000000000000000 ) ) ;
#7901=CARTESIAN_POINT ( 'NONE',  ( 16.17028938446068764, 143.0439382767918346, -16.49999999999050360 ) ) ;
#7902=CARTESIAN_POINT ( 'NONE',  ( 29.69361278289504114, 189.1234298779548624, -27.97726104294733673 ) ) ;
#7905=CARTESIAN_POINT ( 'NONE',  ( -11.06002279671335131, 18.00000000000227374, -10.55202560282026703 ) ) ;
#7906=AXIS2_PLACEMENT_3D ( 'NONE', #1256, #17466, #5337 ) ;
#7907=VERTEX_POINT ( 'NONE', #16817 ) ;
#7909=ORIENTED_EDGE ( 'NONE', *, *, #2912, .F. ) ;
#7911=CARTESIAN_POINT ( 'NONE',  ( 36.00000000000002132, 195.9827547425046816, -25.14811700250533733 ) ) ;
#7915=VERTEX_POINT ( 'NONE', #5125 ) ;
#7916=VECTOR ( 'NONE', #15221, 1000.000000000000000 ) ;
#7917=ADVANCED_FACE ( 'NONE', ( #4781 ), #8839, .T. ) ;
#7922=CARTESIAN_POINT ( 'NONE',  ( 27.48361012698968864, 138.6227766016838245, -1.063447695028167043E-14 ) ) ;
#7923=CARTESIAN_POINT ( 'NONE',  ( 22.99999999999997868, 9.999999999999998224, 0.000000000000000000 ) ) ;
#7924=SHAPE_REPRESENTATION ( 'MirrorLeft Housing Shell', ( #3583 ), #11532 ) ;
#7927=CYLINDRICAL_SURFACE ( 'NONE', #4373, 2.500000000000000444 ) ;
#7928=ORIENTED_EDGE ( 'NONE', *, *, #13498, .F. ) ;
#7929=CARTESIAN_POINT ( 'NONE',  ( -80.90809021110644039, 202.5550951275239413, -16.37659873159346446 ) ) ;
#7931=CARTESIAN_POINT ( 'NONE',  ( 24.60077399342406679, 29.87270634359742871, -7.584611049657961068 ) ) ;
#7936=VERTEX_POINT ( 'NONE', #8919 ) ;
#7939=DIRECTION ( 'NONE',  ( -1.000000000000000000, 0.000000000000000000, 0.000000000000000000 ) ) ;
#7942=DIRECTION ( 'NONE',  ( -1.000000000000000000, 0.000000000000000000, 0.000000000000000000 ) ) ;
#7943=EDGE_CURVE ( 'NONE', #15082, #7515, #15574, .T. ) ;
#7947=CARTESIAN_POINT ( 'NONE',  ( 14.93242934743710570, 18.00000000000000355, -12.99999999999999822 ) ) ;
#7948=CARTESIAN_POINT ( 'NONE',  ( -75.67138096537212277, 142.4529008285661575, -19.34799176589369196 ) ) ;
#7956=VECTOR ( 'NONE', #4024, 1000.000000000000000 ) ;
#7957=ORIENTED_EDGE ( 'NONE', *, *, #10861, .T. ) ;
#7958=CARTESIAN_POINT ( 'NONE',  ( 9.474973892937489595, 133.0798911729450538, -14.49933486760529355 ) ) ;
#7960=CARTESIAN_POINT ( 'NONE',  ( -82.42159468966464431, 152.1166601635960376, -29.06070213693889670 ) ) ;
#7961=CARTESIAN_POINT ( 'NONE',  ( 14.40670567839409344, 127.3124839991112083, -8.619616438334361419 ) ) ;
#7965=DIRECTION ( 'NONE',  ( -1.000000000000000000, -0.000000000000000000, 0.000000000000000000 ) ) ;
#7966=DIRECTION ( 'NONE',  ( -0.000000000000000000, -0.000000000000000000, -1.000000000000000000 ) ) ;
#7967=DIRECTION ( 'NONE',  ( 1.000000000000000000, 0.000000000000000000, 0.000000000000000000 ) ) ;
#7968=CARTESIAN_POINT ( 'NONE',  ( 21.28500206399612438, 29.87397908709612082, -9.872681979495178339 ) ) ;
#7970=CARTESIAN_POINT ( 'NONE',  ( 196.0000000000000000, 167.6227766016838530, -8.071800142134975431 ) ) ;
#7972=EDGE_CURVE ( 'NONE', #5354, #4853, #9889, .T. ) ;
#7973=CARTESIAN_POINT ( 'NONE',  ( -725.0000000000000000, 130.0000000000000000, -13.00000000000000000 ) ) ;
#7974=EDGE_CURVE ( 'NONE', #16285, #10197, #16963, .T. ) ;
#7975=CARTESIAN_POINT ( 'NONE',  ( 25.21634339652309365, 142.9837419059134334, -20.12545249291982330 ) ) ;
#7985=FACE_OUTER_BOUND ( 'NONE', #8661, .T. ) ;
#7986=EDGE_LOOP ( 'NONE', ( #11977, #9195, #3448, #2688, #16696, #5042 ) ) ;
#7987=CARTESIAN_POINT ( 'NONE',  ( 27.50000000000000355, 196.6227766016838245, 1.387778780781445676E-14 ) ) ;
#7990=CARTESIAN_POINT ( 'NONE',  ( -12.66151707385411740, 17.99999999999770495, -6.998435355972849159 ) ) ;
#7994=CARTESIAN_POINT ( 'NONE',  ( -73.02032457293853440, 193.8447098639589683, -24.40281628369250555 ) ) ;
#7996=ORIENTED_EDGE ( 'NONE', *, *, #13635, .T. ) ;
#7998=ORIENTED_EDGE ( 'NONE', *, *, #1101, .T. ) ;
#7999=DIRECTION ( 'NONE',  ( 0.000000000000000000, 0.000000000000000000, 1.000000000000000000 ) ) ;
#8005=CARTESIAN_POINT ( 'NONE',  ( 24.95942568432312214, 149.8830506427267721, -27.43035542581612773 ) ) ;
#8006=CARTESIAN_POINT ( 'NONE',  ( -90.80384757729339640, 204.6227766016838245, 0.000000000000000000 ) ) ;
#8010=DIRECTION ( 'NONE',  ( 0.000000000000000000, 0.000000000000000000, 1.000000000000000000 ) ) ;
#8019=CARTESIAN_POINT ( 'NONE',  ( -80.00000000000002842, 146.6227766016838245, -16.00000000000000000 ) ) ;
#8022=EDGE_CURVE ( 'NONE', #11848, #9167, #8478, .T. ) ;
#8023=CARTESIAN_POINT ( 'NONE',  ( -27.99999999999998224, 10.00000000000000000, -28.00000000000000355 ) ) ;
#8025=CARTESIAN_POINT ( 'NONE',  ( -77.58995968165618251, 141.1235162643940839, -17.17043012754695397 ) ) ;
#8026=CARTESIAN_POINT ( 'NONE',  ( -34.99999999999999289, 122.0000000000000000, 0.000000000000000000 ) ) ;
#8029=ADVANCED_FACE ( 'NONE', ( #2109 ), #796, .F. ) ;
#8031=DIRECTION ( 'NONE',  ( -1.000000000000000000, 0.000000000000000000, 0.000000000000000000 ) ) ;
#8033=CARTESIAN_POINT ( 'NONE',  ( -33.99999999999997868, 10.00000000000000000, -30.00000000000000355 ) ) ;
#8034=EDGE_CURVE ( 'NONE', #11303, #14615, #14150, .T. ) ;
#8035=ORIENTED_EDGE ( 'NONE', *, *, #5983, .T. ) ;
#8036=ADVANCED_BREP_SHAPE_REPRESENTATION ( '', ( #17066, #3583 ), #11532 ) ;
#8037=AXIS2_PLACEMENT_3D ( 'NONE', #10740, #9575, #14981 ) ;
#8038=CARTESIAN_POINT ( 'NONE',  ( 14.92319712166297840, 137.6313713749889587, -10.11910373048704770 ) ) ;
#8041=CARTESIAN_POINT ( 'NONE',  ( -79.55900457720692032, 152.6108673192418337, -29.38619085311482948 ) ) ;
#8042=CARTESIAN_POINT ( 'NONE',  ( 12.08578903453337183, 130.1663611114758510, -11.02150463548631976 ) ) ;
#8045=DIRECTION ( 'NONE',  ( -1.000000000000000000, -0.000000000000000000, 0.000000000000000000 ) ) ;
#8049=CARTESIAN_POINT ( 'NONE',  ( 23.79315516583586643, 18.00000000000000000, -22.94240041036162836 ) ) ;
#8050=AXIS2_PLACEMENT_3D ( 'NONE', #13028, #11677, #3465 ) ;
#8051=CARTESIAN_POINT ( 'NONE',  ( 20.95008785553089581, 29.88049067427350280, -10.28044474760307914 ) ) ;
#8055=EDGE_LOOP ( 'NONE', ( #12067, #10565, #16870, #15840 ) ) ;
#8057=ORIENTED_EDGE ( 'NONE', *, *, #16700, .T. ) ;
#8059=CARTESIAN_POINT ( 'NONE',  ( -8.719536044788691598, 18.00000000000000711, -25.00000000000000000 ) ) ;
#8060=VERTEX_POINT ( 'NONE', #10171 ) ;
#8066=DIRECTION ( 'NONE',  ( 1.000000000000000000, 0.000000000000000000, -0.000000000000000000 ) ) ;
#8071=CARTESIAN_POINT ( 'NONE',  ( 37.50000000000000711, 196.6227766016838245, -21.54065922853802562 ) ) ;
#8072=DIRECTION ( 'NONE',  ( -1.156482317317868274E-16, 1.000000000000000000, 0.000000000000000000 ) ) ;
#8074=ORIENTED_EDGE ( 'NONE', *, *, #15767, .T. ) ;
#8075=CARTESIAN_POINT ( 'NONE',  ( 49.99999999999998579, 167.6227766016838814, -16.92820660268601429 ) ) ;
#8079=CARTESIAN_POINT ( 'NONE',  ( -14.99999999999999467, 90.00000000000000000, -15.00000000000000000 ) ) ;
#8081=AXIS2_PLACEMENT_3D ( 'NONE', #6981, #9450, #15030 ) ;
#8082=EDGE_LOOP ( 'NONE', ( #2052, #15584, #9849, #5605 ) ) ;
#8084=EDGE_CURVE ( 'NONE', #9221, #5721, #5660, .T. ) ;
#8085=EDGE_CURVE ( 'NONE', #11298, #15769, #5202, .T. ) ;
#8092=CARTESIAN_POINT ( 'NONE',  ( 20.96141083122825322, 29.88026331201747254, -10.28670731940101923 ) ) ;
#8095=VERTEX_POINT ( 'NONE', #9442 ) ;
#8096=CARTESIAN_POINT ( 'NONE',  ( -85.99137549878169295, 196.9927911392394151, -24.11293157882131766 ) ) ;
#8103=AXIS2_PLACEMENT_3D ( 'NONE', #8227, #8399, #4428 ) ;
#8108=VERTEX_POINT ( 'NONE', #14074 ) ;
#8110=ORIENTED_EDGE ( 'NONE', *, *, #6233, .F. ) ;
#8111=DIRECTION ( 'NONE',  ( 1.000000000000000000, 0.000000000000000000, -0.000000000000000000 ) ) ;
#8112=DIRECTION ( 'NONE',  ( -1.000000000000000000, -0.000000000000000000, -0.000000000000000000 ) ) ;
#8114=VECTOR ( 'NONE', #11496, 1000.000000000000000 ) ;
#8119=CARTESIAN_POINT ( 'NONE',  ( 196.0000000000000000, 171.6227766016838245, -12.50000337241049131 ) ) ;
#8122=CARTESIAN_POINT ( 'NONE',  ( 35.34723643798712800, 199.3666727680386828, -21.34312735376096626 ) ) ;
#8124=EDGE_CURVE ( 'NONE', #12106, #11342, #12206, .T. ) ;
#8125=( BOUNDED_CURVE ( )  B_SPLINE_CURVE ( 3, ( #7743, #13152, #16979, #7411 ),
 .UNSPECIFIED., .F., .F. ) 
 B_SPLINE_CURVE_WITH_KNOTS ( ( 4, 4 ),
 ( 1.570796326794899000, 3.141592653589791340 ),
 .UNSPECIFIED. ) 
 CURVE ( )  GEOMETRIC_REPRESENTATION_ITEM ( )  RATIONAL_B_SPLINE_CURVE ( ( 1.000000000000000000, 0.8047378541243659367, 0.8047378541243659367, 1.000000000000000000 ) ) 
 REPRESENTATION_ITEM ( '' )  );
#8127=AXIS2_PLACEMENT_3D ( 'NONE', #2369, #14423, #8915 ) ;
#8130=CARTESIAN_POINT ( 'NONE',  ( -74.44332442587726462, 148.9132954376224518, -26.63594553516328034 ) ) ;
#8131=AXIS2_PLACEMENT_3D ( 'NONE', #5992, #8730, #16621 ) ;
#8134=CARTESIAN_POINT ( 'NONE',  ( -75.68538708090720490, 192.4344680579923761, -28.14280641908791836 ) ) ;
#8139=DIRECTION ( 'NONE',  ( 0.000000000000000000, 0.000000000000000000, 1.000000000000000000 ) ) ;
#8140=CARTESIAN_POINT ( 'NONE',  ( 18.50138388889793362, 17.99999999999999289, -12.24385303908842637 ) ) ;
#8141=CARTESIAN_POINT ( 'NONE',  ( 39.99999999999998579, 20.00000000000000000, -30.00000000000001066 ) ) ;
#8142=CYLINDRICAL_SURFACE ( 'NONE', #14953, 6.000000000000005329 ) ;
#8144=CARTESIAN_POINT ( 'NONE',  ( 35.00000000000000711, 146.6227766016838245, -35.00200000000000244 ) ) ;
#8147=CARTESIAN_POINT ( 'NONE',  ( 25.93662097725987437, 142.1921853732338548, -18.94830881272694612 ) ) ;
#8148=ORIENTED_EDGE ( 'NONE', *, *, #2349, .T. ) ;
#8151=CARTESIAN_POINT ( 'NONE',  ( 48.00000000000000711, 167.6227766016838530, -3.071800142134975431 ) ) ;
#8152=DIRECTION ( 'NONE',  ( 1.000000000000000000, 0.000000000000000000, 0.000000000000000000 ) ) ;
#8156=ORIENTED_EDGE ( 'NONE', *, *, #10406, .F. ) ;
#8157=AXIS2_PLACEMENT_3D ( 'NONE', #15149, #5608, #9664 ) ;
#8158=DIRECTION ( 'NONE',  ( 0.000000000000000000, 0.000000000000000000, -1.000000000000000000 ) ) ;
#8159=AXIS2_PLACEMENT_3D ( 'NONE', #8666, #11402, #11489 ) ;
#8161=PLANE ( 'NONE',  #10345 ) ;
#8163=CARTESIAN_POINT ( 'NONE',  ( 196.0000000000000000, 155.6227766016839098, -15.00000337241049486 ) ) ;
#8167=AXIS2_PLACEMENT_3D ( 'NONE', #3811, #6562, #10877 ) ;
#8168=EDGE_CURVE ( 'NONE', #7472, #2271, #11579, .T. ) ;
#8170=VERTEX_POINT ( 'NONE', #13443 ) ;
#8171=CARTESIAN_POINT ( 'NONE',  ( -74.91549491446249931, 191.0841166510127778, -26.65369102675423463 ) ) ;
#8173=DIRECTION ( 'NONE',  ( 1.000000000000000000, 0.000000000000000000, 0.000000000000000000 ) ) ;
#8178=AXIS2_PLACEMENT_3D ( 'NONE', #16977, #16722, #16884 ) ;
#8181=CIRCLE ( 'NONE', #14968, 5.000000000000004441 ) ;
#8185=CARTESIAN_POINT ( 'NONE',  ( 15.00000000000903455, 143.2885527162398489, -16.91661185963483760 ) ) ;
#8188=CARTESIAN_POINT ( 'NONE',  ( -81.75466519885634398, 202.3655582339691250, -16.73015311598867783 ) ) ;
#8193=CARTESIAN_POINT ( 'NONE',  ( 33.88556156013721932, 19.99999999999999645, -11.42442012027869858 ) ) ;
#8197=VECTOR ( 'NONE', #1223, 1000.000000000000000 ) ;
#8198=VERTEX_POINT ( 'NONE', #14849 ) ;
#8200=DIRECTION ( 'NONE',  ( 0.000000000000000000, 1.000000000000000000, 0.000000000000000000 ) ) ;
#8205=CARTESIAN_POINT ( 'NONE',  ( 17.58250999372313927, 125.2198453307267414, -1.671679122699602171 ) ) ;
#8208=CARTESIAN_POINT ( 'NONE',  ( -27.98221281347032274, 30.00000000000000000, -4.999999999999996447 ) ) ;
#8210=VECTOR ( 'NONE', #12887, 1000.000000000000000 ) ;
#8212=CARTESIAN_POINT ( 'NONE',  ( -91.33974596215564645, 171.6227766016838245, 0.000000000000000000 ) ) ;
#8214=FACE_OUTER_BOUND ( 'NONE', #16706, .T. ) ;
#8216=CIRCLE ( 'NONE', #599, 2.499999999999998668 ) ;
#8217=CARTESIAN_POINT ( 'NONE',  ( 25.87766738269516509, 137.9415577646583415, -9.529521052671011461 ) ) ;
#8220=CARTESIAN_POINT ( 'NONE',  ( 15.56337975240378846, 125.2134999403455851, -5.000000000000001776 ) ) ;
#8222=DIRECTION ( 'NONE',  ( 1.000000000000000000, 0.000000000000000000, 0.000000000000000000 ) ) ;
#8224=CARTESIAN_POINT ( 'NONE',  ( 196.0000000000000000, 167.6227766016838814, -19.42820660268601074 ) ) ;
#8226=ADVANCED_FACE ( 'NONE', ( #13533 ), #10862, .T. ) ;
#8227=CARTESIAN_POINT ( 'NONE',  ( -80.00000000000001421, 196.6227766016838245, -13.00000000000000000 ) ) ;
#8228=ADVANCED_FACE ( 'NONE', ( #8214 ), #16372, .T. ) ;
#8231=AXIS2_PLACEMENT_3D ( 'NONE', #13047, #916, #3664 ) ;
#8233=DIRECTION ( 'NONE',  ( 0.000000000000000000, -1.000000000000000000, 0.000000000000000000 ) ) ;
#8235=ORIENTED_EDGE ( 'NONE', *, *, #4592, .T. ) ;
#8236=CARTESIAN_POINT ( 'NONE',  ( -14.83003349241641722, 19.99999999999883116, -8.298189366023557056 ) ) ;
#8237=ORIENTED_EDGE ( 'NONE', *, *, #12607, .F. ) ;
#8238=DIRECTION ( 'NONE',  ( -0.000000000000000000, -0.000000000000000000, -1.000000000000000000 ) ) ;
#8241=ORIENTED_EDGE ( 'NONE', *, *, #14162, .F. ) ;
#8243=CARTESIAN_POINT ( 'NONE',  ( 36.00000000000000711, 196.6227766016838245, -35.00000000000000000 ) ) ;
#8245=ORIENTED_EDGE ( 'NONE', *, *, #12827, .T. ) ;
#8246=CARTESIAN_POINT ( 'NONE',  ( 32.81385839426210538, 153.5807122668280158, -27.63145166803555597 ) ) ;
#8247=ORIENTED_EDGE ( 'NONE', *, *, #8737, .F. ) ;
#8249=CARTESIAN_POINT ( 'NONE',  ( 15.56337975240373872, 125.2134999403456135, -4.999999999999997335 ) ) ;
#8250=CARTESIAN_POINT ( 'NONE',  ( -40.00000000000000000, 0.000000000000000000, -33.00000000000000711 ) ) ;
#8256=EDGE_CURVE ( 'NONE', #2414, #9987, #3980, .T. ) ;
#8257=CARTESIAN_POINT ( 'NONE',  ( -86.98037184620996243, 193.8465113367683443, -24.40116746791569469 ) ) ;
#8261=EDGE_LOOP ( 'NONE', ( #10168, #15508, #10574, #9977 ) ) ;
#8267=DIRECTION ( 'NONE',  ( -1.000000000000000000, 0.000000000000000000, 0.000000000000000000 ) ) ;
#8268=DIRECTION ( 'NONE',  ( 0.000000000000000000, 0.000000000000000000, 1.000000000000000000 ) ) ;
#8269=CARTESIAN_POINT ( 'NONE',  ( 18.00561851734427421, 29.93835620586352064, -12.40035566057732375 ) ) ;
#8273=CARTESIAN_POINT ( 'NONE',  ( -84.31988691467586250, 200.8020376890377463, -19.33395870482236845 ) ) ;
#8275=CARTESIAN_POINT ( 'NONE',  ( 19.49710218362280045, 19.99999999999999289, -24.48336163992366465 ) ) ;
#8276=CARTESIAN_POINT ( 'NONE',  ( -39.68629150101524061, 122.0000000000000000, -9.686291501015231731 ) ) ;
#8278=EDGE_LOOP ( 'NONE', ( #15389, #11150 ) ) ;
#8279=CARTESIAN_POINT ( 'NONE',  ( -3.000000000000000888, 154.3022685259950038, -9.999999999999900524 ) ) ;
#8286=CARTESIAN_POINT ( 'NONE',  ( 27.47046887371370616, 136.6950068244141221, -2.596529902249163690 ) ) ;
#8290=ORIENTED_EDGE ( 'NONE', *, *, #14847, .T. ) ;
#8292=DIRECTION ( 'NONE',  ( 0.000000000000000000, 0.000000000000000000, 1.000000000000000000 ) ) ;
#8293=CARTESIAN_POINT ( 'NONE',  ( -80.00000000000002842, 146.6227766016838245, -16.00000000000000000 ) ) ;
#8294=CARTESIAN_POINT ( 'NONE',  ( 16.01769397135448614, 136.8393535285713369, -3.937079669079308175 ) ) ;
#8296=DIRECTION ( 'NONE',  ( 0.000000000000000000, 0.000000000000000000, 1.000000000000000000 ) ) ;
#8298=ORIENTED_EDGE ( 'NONE', *, *, #6199, .F. ) ;
#8299=EDGE_CURVE ( 'NONE', #13669, #2967, #12548, .T. ) ;
#8300=CARTESIAN_POINT ( 'NONE',  ( -78.20073929934177670, 190.8809388003085417, -29.22564348704268511 ) ) ;
#8301=LINE ( 'NONE', #14952, #1084 ) ;
#8304=CARTESIAN_POINT ( 'NONE',  ( 196.0000000000000000, 171.6227766016838245, -12.50000337241049131 ) ) ;
#8309=ORIENTED_EDGE ( 'NONE', *, *, #5217, .F. ) ;
#8310=CARTESIAN_POINT ( 'NONE',  ( -11.99122994684825549, 19.99999999999999645, -24.50500383881168176 ) ) ;
#8311=VECTOR ( 'NONE', #11174, 1000.000000000000000 ) ;
#8312=ORIENTED_EDGE ( 'NONE', *, *, #624, .T. ) ;
#8315=ORIENTED_EDGE ( 'NONE', *, *, #9520, .T. ) ;
#8316=EDGE_CURVE ( 'NONE', #15643, #17487, #1927, .T. ) ;
#8320=CARTESIAN_POINT ( 'NONE',  ( 33.07446265461972956, 153.4692325703934159, -27.55849099911372591 ) ) ;
#8322=ORIENTED_EDGE ( 'NONE', *, *, #1653, .T. ) ;
#8324=B_SPLINE_CURVE_WITH_KNOTS ( 'NONE', 3,
 ( #14168, #701, #6269, #17151, #15570, #16991, #15647, #7421, #6093, #1043, #5026, #11492, #4858, #3617, #10248, #10510, #952, #7677, #16901, #3447 ),
 .UNSPECIFIED., .F., .F.,
 ( 4, 2, 2, 2, 2, 2, 2, 2, 2, 4 ),
 ( 0.000000000000000000, 0.002053780611527093129, 0.004107561223054186257, 0.006161341834581279819, 0.008215122446108372514, 0.01026890305763546694, 0.01232268366916255964, 0.01437646428068965233, 0.01540335458645322037, 0.01643024489221679013 ),
 .UNSPECIFIED. ) ;
#8330=CYLINDRICAL_SURFACE ( 'NONE', #1258, 5.000000000000004441 ) ;
#8333=CARTESIAN_POINT ( 'NONE',  ( 27.19159743497788284, 137.1791639268274992, -6.327035192214271575 ) ) ;
#8335=CARTESIAN_POINT ( 'NONE',  ( -83.81731182140758563, 190.1433283039765172, -27.31438289289431509 ) ) ;
#8336=CARTESIAN_POINT ( 'NONE',  ( -77.50000000000001421, 196.6227766016838245, 1.387778780781445676E-14 ) ) ;
#8338=CARTESIAN_POINT ( 'NONE',  ( -7.922882945419460476, 30.18055256556250399, -13.00000000000000355 ) ) ;
#8339=ORIENTED_EDGE ( 'NONE', *, *, #3064, .F. ) ;
#8343=AXIS2_PLACEMENT_3D ( 'NONE', #1511, #10978, #12306 ) ;
#8344=FACE_OUTER_BOUND ( 'NONE', #3994, .T. ) ;
#8346=VERTEX_POINT ( 'NONE', #3348 ) ;
#8348=DIRECTION ( 'NONE',  ( 0.000000000000000000, 0.000000000000000000, 1.000000000000000000 ) ) ;
#8349=EDGE_CURVE ( 'NONE', #11303, #1820, #13804, .T. ) ;
#8351=ADVANCED_FACE ( 'NONE', ( #1669 ), #13971, .T. ) ;
#8352=AXIS2_PLACEMENT_3D ( 'NONE', #5466, #4140, #9526 ) ;
#8353=DIRECTION ( 'NONE',  ( 1.000000000000000000, 0.000000000000000000, 0.000000000000000000 ) ) ;
#8359=VECTOR ( 'NONE', #13021, 1000.000000000000000 ) ;
#8360=DIRECTION ( 'NONE',  ( 0.000000000000000000, 0.000000000000000000, -1.000000000000000000 ) ) ;
#8366=ORIENTED_EDGE ( 'NONE', *, *, #8124, .T. ) ;
#8367=CIRCLE ( 'NONE', #6684, 25.00000000000000000 ) ;
#8368=CARTESIAN_POINT ( 'NONE',  ( -147.9615242270661213, 171.6227766016838245, 0.000000000000000000 ) ) ;
#8371=FACE_OUTER_BOUND ( 'NONE', #5527, .T. ) ;
#8374=CARTESIAN_POINT ( 'NONE',  ( -35.49999999999998579, 10.00000000000000178, -13.00000000000000000 ) ) ;
#8376=DIRECTION ( 'NONE',  ( -0.000000000000000000, -0.000000000000000000, -1.000000000000000000 ) ) ;
#8377=CARTESIAN_POINT ( 'NONE',  ( 37.50000000000000711, 146.6227766016838245, -21.54065922853802562 ) ) ;
#8379=CIRCLE ( 'NONE', #10070, 5.000000000000018652 ) ;
#8380=VERTEX_POINT ( 'NONE', #7234 ) ;
#8385=CYLINDRICAL_SURFACE ( 'NONE', #15137, 2.500000000000000444 ) ;
#8387=ADVANCED_FACE ( 'NONE', ( #14152 ), #12638, .T. ) ;
#8389=CARTESIAN_POINT ( 'NONE',  ( 27.25143353317894324, 137.1251711682953385, -6.002437647192902404 ) ) ;
#8390=ORIENTED_EDGE ( 'NONE', *, *, #14232, .F. ) ;
#8392=CARTESIAN_POINT ( 'NONE',  ( 13.73607130285369138, 138.7967234794426190, -3.453855393587564659 ) ) ;
#8393=ORIENTED_EDGE ( 'NONE', *, *, #2877, .T. ) ;
#8395=CARTESIAN_POINT ( 'NONE',  ( -74.00000000000001421, 195.9827547425045680, -25.14811700250532311 ) ) ;
#8399=DIRECTION ( 'NONE',  ( 0.000000000000000000, 0.000000000000000000, 1.000000000000000000 ) ) ;
#8405=EDGE_CURVE ( 'NONE', #2271, #7472, #12743, .T. ) ;
#8409=ORIENTED_EDGE ( 'NONE', *, *, #13073, .T. ) ;
#8410=VERTEX_POINT ( 'NONE', #13187 ) ;
#8412=EDGE_CURVE ( 'NONE', #6662, #14433, #8125, .T. ) ;
#8418=CARTESIAN_POINT ( 'NONE',  ( 25.75320729262171682, 152.8105824767976060, -27.11332964807918344 ) ) ;
#8420=VECTOR ( 'NONE', #12984, 1000.000000000000000 ) ;
#8423=CARTESIAN_POINT ( 'NONE',  ( 17.00000000000000000, 171.6227766016838245, 0.000000000000000000 ) ) ;
#8427=PLANE ( 'NONE',  #7195 ) ;
#8430=FACE_OUTER_BOUND ( 'NONE', #5000, .T. ) ;
#8433=DIRECTION ( 'NONE',  ( 1.000000000000000000, 0.000000000000000000, 0.000000000000000000 ) ) ;
#8434=CARTESIAN_POINT ( 'NONE',  ( 48.00000000000000711, 163.6227766016838530, -10.00000337241049309 ) ) ;
#8437=VERTEX_POINT ( 'NONE', #3511 ) ;
#8440=DIRECTION ( 'NONE',  ( 0.000000000000000000, -1.000000000000000000, 0.000000000000000000 ) ) ;
#8442=ORIENTED_EDGE ( 'NONE', *, *, #7355, .T. ) ;
#8444=DIRECTION ( 'NONE',  ( 1.000000000000000000, 0.000000000000000000, 0.000000000000000000 ) ) ;
#8445=CARTESIAN_POINT ( 'NONE',  ( 48.00000000000000711, 167.6227766016838530, -5.571800142134975431 ) ) ;
#8446=CARTESIAN_POINT ( 'NONE',  ( 19.82112781281243130, 29.90253658286262350, -11.35562597552217845 ) ) ;
#8454=ORIENTED_EDGE ( 'NONE', *, *, #5217, .T. ) ;
#8459=LINE ( 'NONE', #4128, #11196 ) ;
#8462=ADVANCED_FACE ( 'NONE', ( #17223 ), #11723, .F. ) ;
#8467=ORIENTED_EDGE ( 'NONE', *, *, #15639, .T. ) ;
#8469=AXIS2_PLACEMENT_3D ( 'NONE', #12598, #15160, #9940 ) ;
#8471=DIRECTION ( 'NONE',  ( -1.000000000000000000, 0.000000000000000000, 0.000000000000000000 ) ) ;
#8474=LINE ( 'NONE', #408, #16280 ) ;
#8475=CARTESIAN_POINT ( 'NONE',  ( 22.65507808637627818, 17.99999999999885958, -7.619675430596801746 ) ) ;
#8478=CIRCLE ( 'NONE', #8766, 10.00000000000000178 ) ;
#8486=CARTESIAN_POINT ( 'NONE',  ( 48.00000000000000711, 187.6227766016837961, -12.50000337241049309 ) ) ;
#8488=AXIS2_PLACEMENT_3D ( 'NONE', #6170, #15558, #8899 ) ;
#8490=CARTESIAN_POINT ( 'NONE',  ( -74.60025079181714602, 194.0006876528842383, -26.91236748077486141 ) ) ;
#8495=DIRECTION ( 'NONE',  ( 1.000000000000000000, 0.000000000000000000, 0.000000000000000000 ) ) ;
#8498=FACE_BOUND ( 'NONE', #9099, .T. ) ;
#8501=ORIENTED_EDGE ( 'NONE', *, *, #2294, .T. ) ;
#8504=DIRECTION ( 'NONE',  ( -1.000000000000000000, 0.000000000000000000, 0.000000000000000000 ) ) ;
#8505=VERTEX_POINT ( 'NONE', #7663 ) ;
#8509=CARTESIAN_POINT ( 'NONE',  ( 36.65543510501046143, 200.1146145092351958, -16.67123533649926870 ) ) ;
#8512=EDGE_CURVE ( 'NONE', #4546, #12075, #4919, .T. ) ;
#8514=EDGE_CURVE ( 'NONE', #8812, #8947, #11593, .T. ) ;
#8515=CARTESIAN_POINT ( 'NONE',  ( -75.00000000000002842, 146.6227766016838245, -12.99999999999999822 ) ) ;
#8516=FACE_OUTER_BOUND ( 'NONE', #9693, .T. ) ;
#8521=CARTESIAN_POINT ( 'NONE',  ( 26.38776508739448801, 137.6838126476015134, -8.633687169601740763 ) ) ;
#8522=VERTEX_POINT ( 'NONE', #14484 ) ;
#8524=AXIS2_PLACEMENT_3D ( 'NONE', #4278, #7016, #7272 ) ;
#8525=CARTESIAN_POINT ( 'NONE',  ( -12.54777316999452275, 31.64944667534048861, -11.54374194473465920 ) ) ;
#8526=ORIENTED_EDGE ( 'NONE', *, *, #5496, .F. ) ;
#8527=ORIENTED_EDGE ( 'NONE', *, *, #10443, .T. ) ;
#8528=DIRECTION ( 'NONE',  ( 0.000000000000000000, 8.410780489584519664E-16, 1.000000000000000000 ) ) ;
#8531=VERTEX_POINT ( 'NONE', #5102 ) ;
#8533=DIRECTION ( 'NONE',  ( 0.000000000000000000, 0.000000000000000000, -1.000000000000000000 ) ) ;
#8539=EDGE_LOOP ( 'NONE', ( #1081, #14176, #8035, #12509 ) ) ;
#8540=CARTESIAN_POINT ( 'NONE',  ( -75.66955265303195688, 200.7908024820230253, -19.35080275744227407 ) ) ;
#8541=DIRECTION ( 'NONE',  ( -1.000000000000000000, -0.000000000000000000, 0.000000000000000000 ) ) ;
#8547=VERTEX_POINT ( 'NONE', #3769 ) ;
#8548=CARTESIAN_POINT ( 'NONE',  ( 6.134011831684053284, 134.2062027339443944, -15.00000000000000000 ) ) ;
#8550=ADVANCED_FACE ( 'NONE', ( #9163 ), #14569, .F. ) ;
#8554=DIRECTION ( 'NONE',  ( -0.000000000000000000, -0.000000000000000000, 1.000000000000000000 ) ) ;
#8555=CARTESIAN_POINT ( 'NONE',  ( -27.99999999999998224, 10.00000000000000000, 0.000000000000000000 ) ) ;
#8556=DIRECTION ( 'NONE',  ( -0.000000000000000000, -0.000000000000000000, 1.000000000000000000 ) ) ;
#8559=DIRECTION ( 'NONE',  ( -1.000000000000000000, -0.000000000000000000, -0.000000000000000000 ) ) ;
#8561=CARTESIAN_POINT ( 'NONE',  ( -725.0000000000000000, 19.99999999999995737, -15.00000000000000000 ) ) ;
#8564=ORIENTED_EDGE ( 'NONE', *, *, #3503, .T. ) ;
#8566=CARTESIAN_POINT ( 'NONE',  ( 27.47054928355543169, 136.6945666198121216, -2.592592592592591672 ) ) ;
#8567=ORIENTED_EDGE ( 'NONE', *, *, #15097, .F. ) ;
#8570=DIRECTION ( 'NONE',  ( 1.000000000000000000, 0.000000000000000000, 0.000000000000000000 ) ) ;
#8576=CARTESIAN_POINT ( 'NONE',  ( -725.0000000000000000, 19.99999999999995737, -4.999999999999999112 ) ) ;
#8577=CYLINDRICAL_SURFACE ( 'NONE', #14667, 8.000000000000000000 ) ;
#8582=VERTEX_POINT ( 'NONE', #10577 ) ;
#8585=EDGE_CURVE ( 'NONE', #11464, #10357, #10844, .T. ) ;
#8587=CARTESIAN_POINT ( 'NONE',  ( 32.50000000000000711, 146.6227766016838245, 1.387778780781445676E-14 ) ) ;
#8590=CARTESIAN_POINT ( 'NONE',  ( 23.02032457293857348, 149.4008433394087092, -24.40281628369250200 ) ) ;
#8595=DIRECTION ( 'NONE',  ( 0.000000000000000000, 0.000000000000000000, 1.000000000000000000 ) ) ;
#8597=CIRCLE ( 'NONE', #2101, 20.00000000000000355 ) ;
#8598=LINE ( 'NONE', #369, #971 ) ;
#8599=CARTESIAN_POINT ( 'NONE',  ( -73.58001751434005655, 142.7179894756439751, -15.94334347237690430 ) ) ;
#8600=VERTEX_POINT ( 'NONE', #9510 ) ;
#8601=DIRECTION ( 'NONE',  ( 0.000000000000000000, 0.000000000000000000, 1.000000000000000000 ) ) ;
#8602=ORIENTED_EDGE ( 'NONE', *, *, #2237, .T. ) ;
#8603=DIRECTION ( 'NONE',  ( -6.938893903907228378E-16, 1.000000000000000000, 0.000000000000000000 ) ) ;
#8606=EDGE_CURVE ( 'NONE', #9042, #5256, #7373, .T. ) ;
#8607=EDGE_CURVE ( 'NONE', #6756, #10807, #13016, .T. ) ;
#8609=CARTESIAN_POINT ( 'NONE',  ( -22.99999999999998224, 10.00000000000000000, -35.00200000000000244 ) ) ;
#8610=CIRCLE ( 'NONE', #14547, 2.499999999999998668 ) ;
#8614=ORIENTED_EDGE ( 'NONE', *, *, #1484, .F. ) ;
#8615=CARTESIAN_POINT ( 'NONE',  ( 27.99999999999998224, 9.999999999999998224, -16.00000000000000000 ) ) ;
#8617=DIRECTION ( 'NONE',  ( -1.000000000000000000, 0.000000000000000000, 0.000000000000000000 ) ) ;
#8620=CARTESIAN_POINT ( 'NONE',  ( 25.00000000000000711, 146.6227766016838245, 0.000000000000000000 ) ) ;
#8621=AXIS2_PLACEMENT_3D ( 'NONE', #8423, #13841, #8595 ) ;
#8623=CARTESIAN_POINT ( 'NONE',  ( -68.00000000000000000, 154.3022685259950038, -9.999999999999900524 ) ) ;
#8624=CIRCLE ( 'NONE', #13721, 30.00000000000000000 ) ;
#8625=DIRECTION ( 'NONE',  ( 1.000000000000000000, 0.000000000000000000, 0.000000000000000000 ) ) ;
#8632=ORIENTED_EDGE ( 'NONE', *, *, #1653, .F. ) ;
#8639=ORIENTED_EDGE ( 'NONE', *, *, #7097, .F. ) ;
#8646=DIRECTION ( 'NONE',  ( -1.000000000000000000, 0.000000000000000000, 0.000000000000000000 ) ) ;
#8652=EDGE_CURVE ( 'NONE', #1245, #11878, #15277, .T. ) ;
#8653=CARTESIAN_POINT ( 'NONE',  ( -12.78554710720352894, 31.18907022382790117, -13.71297843187037202 ) ) ;
#8656=B_SPLINE_CURVE_WITH_KNOTS ( 'NONE', 3,
 ( #10991, #13576, #14806, #8249 ),
 .UNSPECIFIED., .F., .F.,
 ( 4, 4 ),
 ( 0.000000000000000000, 0.005007666328367723664 ),
 .UNSPECIFIED. ) ;
#8658=CYLINDRICAL_SURFACE ( 'NONE', #15826, 2.500000000000002220 ) ;
#8659=EDGE_LOOP ( 'NONE', ( #4458, #9821 ) ) ;
#8661=EDGE_LOOP ( 'NONE', ( #15110, #16420, #3102, #5987, #3998 ) ) ;
#8666=CARTESIAN_POINT ( 'NONE',  ( 15.00000000000000000, 171.6227766016838245, 0.000000000000000000 ) ) ;
#8667=AXIS2_PLACEMENT_3D ( 'NONE', #6734, #6642, #2581 ) ;
#8669=VERTEX_POINT ( 'NONE', #12444 ) ;
#8670=DIRECTION ( 'NONE',  ( 0.000000000000000000, 0.000000000000000000, 1.000000000000000000 ) ) ;
#8672=CARTESIAN_POINT ( 'NONE',  ( 21.99999999999998224, 9.999999999999998224, -16.00000000000000000 ) ) ;
#8674=PLANE ( 'NONE',  #9758 ) ;
#8677=CARTESIAN_POINT ( 'NONE',  ( 32.90650748920315039, 19.99999999999999645, -13.87185692902932921 ) ) ;
#8679=CARTESIAN_POINT ( 'NONE',  ( 21.47128797932978372, 141.5899928260317040, -13.68519783011616653 ) ) ;
#8682=ADVANCED_FACE ( 'NONE', ( #316 ), #4389, .F. ) ;
#8688=CARTESIAN_POINT ( 'NONE',  ( 35.27494917608787972, 201.9542783778900059, -13.00000000000000000 ) ) ;
#8693=CONICAL_SURFACE ( 'NONE', #8972, 35.00000000000000000, 0.5235987755983005920 ) ;
#8694=DIRECTION ( 'NONE',  ( -1.000000000000000000, -0.000000000000000000, -0.000000000000000000 ) ) ;
#8696=DIRECTION ( 'NONE',  ( 1.000000000000000000, 1.156482317317868274E-16, 0.000000000000000000 ) ) ;
#8698=DIRECTION ( 'NONE',  ( 0.000000000000000000, 0.000000000000000000, 1.000000000000000000 ) ) ;
#8699=ORIENTED_EDGE ( 'NONE', *, *, #843, .T. ) ;
#8700=DIRECTION ( 'NONE',  ( -1.000000000000000000, -0.000000000000000000, 0.000000000000000000 ) ) ;
#8701=DIRECTION ( 'NONE',  ( -0.000000000000000000, -0.000000000000000000, 1.000000000000000000 ) ) ;
#8705=AXIS2_PLACEMENT_3D ( 'NONE', #14038, #12706, #7207 ) ;
#8709=ORIENTED_EDGE ( 'NONE', *, *, #6612, .T. ) ;
#8711=CARTESIAN_POINT ( 'NONE',  ( -5.000000000000000888, 154.3022685259950038, -9.999999999999900524 ) ) ;
#8713=CARTESIAN_POINT ( 'NONE',  ( 27.44407568426044364, 136.8394969516870958, -3.888888888888887063 ) ) ;
#8714=EDGE_CURVE ( 'NONE', #11591, #8346, #15290, .T. ) ;
#8721=CARTESIAN_POINT ( 'NONE',  ( 196.0000000000000000, 187.6227766016837961, -10.00000337241049309 ) ) ;
#8725=FACE_BOUND ( 'NONE', #7112, .T. ) ;
#8729=ORIENTED_EDGE ( 'NONE', *, *, #8714, .F. ) ;
#8730=DIRECTION ( 'NONE',  ( -0.000000000000000000, -0.000000000000000000, -1.000000000000000000 ) ) ;
#8732=VECTOR ( 'NONE', #1022, 1000.000000000000000 ) ;
#8733=CARTESIAN_POINT ( 'NONE',  ( 196.0000000000000000, 175.6227766016838245, -3.071800142134975431 ) ) ;
#8737=EDGE_CURVE ( 'NONE', #5595, #11327, #1904, .T. ) ;
#8738=CARTESIAN_POINT ( 'NONE',  ( -15.00000000000002487, 120.0000000000000284, -4.999999999999999112 ) ) ;
#8741=DIRECTION ( 'NONE',  ( 0.000000000000000000, 1.000000000000000000, 0.000000000000000000 ) ) ;
#8742=CARTESIAN_POINT ( 'NONE',  ( -80.00000000000002842, 146.6227766016838245, 0.000000000000000000 ) ) ;
#8743=CARTESIAN_POINT ( 'NONE',  ( -33.99999999999997868, 10.00000000000000000, -35.00000000000000000 ) ) ;
#8744=CARTESIAN_POINT ( 'NONE',  ( -13.95500183466744382, 31.43484250012364001, -12.98634364776042638 ) ) ;
#8745=CIRCLE ( 'NONE', #5060, 2.499999999999998668 ) ;
#8748=DIRECTION ( 'NONE',  ( -0.000000000000000000, -0.000000000000000000, -1.000000000000000000 ) ) ;
#8750=CARTESIAN_POINT ( 'NONE',  ( 27.44407568426044364, 136.8394969516870958, -3.888888888888887063 ) ) ;
#8751=ORIENTED_EDGE ( 'NONE', *, *, #16101, .F. ) ;
#8753=DIRECTION ( 'NONE',  ( -0.000000000000000000, -0.000000000000000000, 1.000000000000000000 ) ) ;
#8754=VECTOR ( 'NONE', #13626, 1000.000000000000000 ) ;
#8761=CARTESIAN_POINT ( 'NONE',  ( 31.78129305203702870, 202.3573166656175033, -16.74530232247016315 ) ) ;
#8764=CARTESIAN_POINT ( 'NONE',  ( 14.93242934743711814, 30.00000000000000000, -15.00000000000000000 ) ) ;
#8765=AXIS2_PLACEMENT_3D ( 'NONE', #3175, #13975, #5824 ) ;
#8766=AXIS2_PLACEMENT_3D ( 'NONE', #11587, #15651, #7682 ) ;
#8768=VERTEX_POINT ( 'NONE', #15273 ) ;
#8771=CARTESIAN_POINT ( 'NONE',  ( 9.072488053085830728, 140.2836875516620978, -12.31648485192419784 ) ) ;
#8776=ADVANCED_FACE ( 'NONE', ( #16517 ), #6239, .F. ) ;
#8778=CARTESIAN_POINT ( 'NONE',  ( 30.00000000000001066, 146.6227766016838245, 0.000000000000000000 ) ) ;
#8781=CARTESIAN_POINT ( 'NONE',  ( -22.93725393319378369, 20.00000000000004263, -5.999999999999992895 ) ) ;
#8784=CARTESIAN_POINT ( 'NONE',  ( 30.27573706856752622, 140.6276388071887595, -16.25736180127249852 ) ) ;
#8787=EDGE_LOOP ( 'NONE', ( #10884, #6890 ) ) ;
#8791=DIRECTION ( 'NONE',  ( 1.000000000000000000, 0.000000000000000000, 0.000000000000000000 ) ) ;
#8795=EDGE_CURVE ( 'NONE', #15177, #1173, #12186, .T. ) ;
#8796=VERTEX_POINT ( 'NONE', #4481 ) ;
#8799=EDGE_CURVE ( 'NONE', #9221, #8198, #9866, .T. ) ;
#8800=CARTESIAN_POINT ( 'NONE',  ( -18.25212770525997286, 32.30769230769230660, -4.999999999999999112 ) ) ;
#8803=EDGE_CURVE ( 'NONE', #13322, #10334, #5889, .T. ) ;
#8804=ADVANCED_FACE ( 'NONE', ( #9952 ), #7300, .F. ) ;
#8806=CARTESIAN_POINT ( 'NONE',  ( 30.00000000000000355, 196.6227766016838245, -35.00200000000000244 ) ) ;
#8807=CIRCLE ( 'NONE', #2864, 12.00000000000000000 ) ;
#8808=CARTESIAN_POINT ( 'NONE',  ( -18.25212770525996930, 32.30769230769230660, 0.000000000000000000 ) ) ;
#8811=CARTESIAN_POINT ( 'NONE',  ( 225.0000000000000000, 89.99999999999997158, 0.000000000000000000 ) ) ;
#8812=VERTEX_POINT ( 'NONE', #8808 ) ;
#8814=ADVANCED_FACE ( 'NONE', ( #16956 ), #12964, .F. ) ;
#8821=CARTESIAN_POINT ( 'NONE',  ( -22.99999999999999289, 90.00000000000000000, -4.999999999999999112 ) ) ;
#8824=CARTESIAN_POINT ( 'NONE',  ( -9.703671380219324405, 20.00000000000114397, -14.18606485937966788 ) ) ;
#8828=EDGE_CURVE ( 'NONE', #3065, #4370, #3324, .T. ) ;
#8829=EDGE_CURVE ( 'NONE', #15643, #11995, #15405, .T. ) ;
#8832=ORIENTED_EDGE ( 'NONE', *, *, #6071, .F. ) ;
#8836=DIRECTION ( 'NONE',  ( 0.8660254037844378194, -0.5000000000000015543, -0.000000000000000000 ) ) ;
#8837=ORIENTED_EDGE ( 'NONE', *, *, #8412, .T. ) ;
#8838=CARTESIAN_POINT ( 'NONE',  ( -2.428612866367531510E-15, 18.00000000000000355, -28.00000000000000711 ) ) ;
#8839=PLANE ( 'NONE',  #7620 ) ;
#8840=CARTESIAN_POINT ( 'NONE',  ( 31.31294070251087192, 202.4787130041031560, -16.52010876963832331 ) ) ;
#8841=EDGE_LOOP ( 'NONE', ( #6766, #6868, #3575, #1254 ) ) ;
#8842=ORIENTED_EDGE ( 'NONE', *, *, #16680, .F. ) ;
#8843=CARTESIAN_POINT ( 'NONE',  ( 22.30340133326367180, 19.99999999999999645, -11.90876978475634651 ) ) ;
#8847=CARTESIAN_POINT ( 'NONE',  ( -15.00000000000002487, 120.0000000000000284, -4.999999999999999112 ) ) ;
#8848=FACE_OUTER_BOUND ( 'NONE', #1143, .T. ) ;
#8849=VERTEX_POINT ( 'NONE', #11628 ) ;
#8854=DIRECTION ( 'NONE',  ( 1.000000000000000000, 0.000000000000000000, 0.000000000000000000 ) ) ;
#8855=CYLINDRICAL_SURFACE ( 'NONE', #9447, 20.00000000000000355 ) ;
#8858=ORIENTED_EDGE ( 'NONE', *, *, #16392, .F. ) ;
#8861=CARTESIAN_POINT ( 'NONE',  ( -24.99999999999999645, 120.0000000000000284, -15.00000000000000000 ) ) ;
#8864=CARTESIAN_POINT ( 'NONE',  ( -74.72505082391211317, 201.9542783778900059, -13.00000000000000000 ) ) ;
#8868=CARTESIAN_POINT ( 'NONE',  ( -34.99999999999999289, 130.0000000000000000, -15.00000000000000000 ) ) ;
#8869=DIRECTION ( 'NONE',  ( -1.000000000000000000, -0.000000000000000000, 0.000000000000000000 ) ) ;
#8871=PLANE ( 'NONE',  #6062 ) ;
#8873=CARTESIAN_POINT ( 'NONE',  ( 30.00000000000001066, 146.6227766016838245, 0.000000000000000000 ) ) ;
#8874=CARTESIAN_POINT ( 'NONE',  ( 30.00000000000001066, 146.6227766016838245, -35.00000000000000000 ) ) ;
#8877=DIRECTION ( 'NONE',  ( 0.000000000000000000, 0.000000000000000000, -1.000000000000000000 ) ) ;
#8882=ORIENTED_EDGE ( 'NONE', *, *, #6876, .T. ) ;
#8883=ORIENTED_EDGE ( 'NONE', *, *, #564, .F. ) ;
#8886=CARTESIAN_POINT ( 'NONE',  ( -87.50000000000002842, 146.8102797458443547, -21.75827460206394193 ) ) ;
#8887=EDGE_CURVE ( 'NONE', #6145, #874, #1784, .T. ) ;
#8890=LINE ( 'NONE', #14299, #9198 ) ;
#8894=DIRECTION ( 'NONE',  ( 1.000000000000000000, 0.000000000000000000, 0.000000000000000000 ) ) ;
#8896=VERTEX_POINT ( 'NONE', #16753 ) ;
#8897=DIRECTION ( 'NONE',  ( -1.000000000000000000, 0.000000000000000000, 0.000000000000000000 ) ) ;
#8898=CARTESIAN_POINT ( 'NONE',  ( 27.44407568426044008, 126.9014170516880284, -4.999999999999997335 ) ) ;
#8899=DIRECTION ( 'NONE',  ( 0.000000000000000000, 0.000000000000000000, 1.000000000000000000 ) ) ;
#8900=CARTESIAN_POINT ( 'NONE',  ( -3.000000000000000888, 191.6227766016837961, 1.224646799147353454E-15 ) ) ;
#8902=VECTOR ( 'NONE', #5603, 1000.000000000000000 ) ;
#8904=ORIENTED_EDGE ( 'NONE', *, *, #13025, .F. ) ;
#8905=LINE ( 'NONE', #5826, #4729 ) ;
#8915=DIRECTION ( 'NONE',  ( -1.000000000000000000, 0.000000000000000000, 0.000000000000000000 ) ) ;
#8917=ADVANCED_FACE ( 'NONE', ( #5765 ), #15240, .T. ) ;
#8919=CARTESIAN_POINT ( 'NONE',  ( 15.60228996708978855, 124.9392590763941371, 1.387778780781445676E-14 ) ) ;
#8920=CARTESIAN_POINT ( 'NONE',  ( 34.79035048419334686, 200.2528945340144446, -20.13811431823772935 ) ) ;
#8921=ORIENTED_EDGE ( 'NONE', *, *, #13073, .F. ) ;
#8923=CIRCLE ( 'NONE', #8081, 740.0000000000000000 ) ;
#8925=CARTESIAN_POINT ( 'NONE',  ( 19.14963388379468157, 19.99999999999999645, -24.55317681541820463 ) ) ;
#8926=DIRECTION ( 'NONE',  ( 0.000000000000000000, 0.000000000000000000, -1.000000000000000000 ) ) ;
#8928=DIRECTION ( 'NONE',  ( 0.000000000000000000, 2.775557561562891351E-15, -1.000000000000000000 ) ) ;
#8930=AXIS2_PLACEMENT_3D ( 'NONE', #3660, #2239, #17291 ) ;
#8936=EDGE_CURVE ( 'NONE', #16407, #3419, #8216, .T. ) ;
#8942=DIRECTION ( 'NONE',  ( -1.000000000000000000, -6.938893903907228378E-16, -0.000000000000000000 ) ) ;
#8944=ORIENTED_EDGE ( 'NONE', *, *, #11935, .F. ) ;
#8946=VECTOR ( 'NONE', #10967, 1000.000000000000000 ) ;
#8947=VERTEX_POINT ( 'NONE', #11075 ) ;
#8951=CARTESIAN_POINT ( 'NONE',  ( -70.00000000000000000, 171.6227766016838245, -20.00000000000000355 ) ) ;
#8953=CARTESIAN_POINT ( 'NONE',  ( -27.98221281347037959, 30.00000000000000000, 0.000000000000000000 ) ) ;
#8956=EDGE_LOOP ( 'NONE', ( #14944, #13979, #15431, #5439 ) ) ;
#8960=CYLINDRICAL_SURFACE ( 'NONE', #7519, 7.500000000000000000 ) ;
#8962=CARTESIAN_POINT ( 'NONE',  ( 33.54345905997184474, 190.0067896460676309, -27.40528370530127233 ) ) ;
#8964=CARTESIAN_POINT ( 'NONE',  ( -10.22933296213221865, 30.92590585860461161, -12.59260918105267457 ) ) ;
#8966=CARTESIAN_POINT ( 'NONE',  ( -43.00000000000000000, 138.6227766016838245, 0.000000000000000000 ) ) ;
#8969=CARTESIAN_POINT ( 'NONE',  ( 35.04511979140807654, 193.3541989604593141, -27.43934207688683813 ) ) ;
#8971=VERTEX_POINT ( 'NONE', #16490 ) ;
#8972=AXIS2_PLACEMENT_3D ( 'NONE', #8212, #1311, #5298 ) ;
#8973=EDGE_LOOP ( 'NONE', ( #5170, #7437, #15682, #5013 ) ) ;
#8977=CARTESIAN_POINT ( 'NONE',  ( -77.72043220849697320, 153.7735974263995047, -27.75644086540375355 ) ) ;
#8980=CARTESIAN_POINT ( 'NONE',  ( 27.44407568426047561, 138.8271129316868837, -3.666666666666728247 ) ) ;
#8982=DIRECTION ( 'NONE',  ( -1.000000000000000000, -0.000000000000000000, 0.000000000000000000 ) ) ;
#8983=CARTESIAN_POINT ( 'NONE',  ( 30.89296198743065602, 152.5603119736738620, -29.35342143133167880 ) ) ;
#8986=CIRCLE ( 'NONE', #17485, 2.500000000000002220 ) ;
#8987=EDGE_LOOP ( 'NONE', ( #11064, #11121 ) ) ;
#8995=CARTESIAN_POINT ( 'NONE',  ( -68.00000000000000000, 191.6227766016837961, 1.224646799147353454E-15 ) ) ;
#8996=CIRCLE ( 'NONE', #238, 6.000000000000005329 ) ;
#8998=CARTESIAN_POINT ( 'NONE',  ( -27.99999999999998224, 10.00000000000000000, -16.00000000000000000 ) ) ;
#9000=CARTESIAN_POINT ( 'NONE',  ( 30.00000000000000355, 196.6227766016838245, -16.00000000000000000 ) ) ;
#9002=DIRECTION ( 'NONE',  ( 0.000000000000000000, 0.000000000000000000, 1.000000000000000000 ) ) ;
#9003=CARTESIAN_POINT ( 'NONE',  ( 16.74904763372935790, 29.96341334642810139, -12.79227977592015897 ) ) ;
#9010=AXIS2_PLACEMENT_3D ( 'NONE', #12795, #6060, #7214 ) ;
#9012=CIRCLE ( 'NONE', #7330, 7.500000000000007105 ) ;
#9013=CARTESIAN_POINT ( 'NONE',  ( 25.21468100261554568, 200.2598589880381610, -20.12830716182790169 ) ) ;
#9014=EDGE_CURVE ( 'NONE', #14931, #15920, #4274, .T. ) ;
#9017=CARTESIAN_POINT ( 'NONE',  ( 19.05951714192248403, 29.94485528828719367, -14.11495713418740294 ) ) ;
#9018=CARTESIAN_POINT ( 'NONE',  ( 6.134011831684060390, 139.5514275721929209, -14.99999999999999822 ) ) ;
#9019=VERTEX_POINT ( 'NONE', #222 ) ;
#9020=CARTESIAN_POINT ( 'NONE',  ( -83.36213377134494351, 151.5968920417502090, -28.70510347301451404 ) ) ;
#9021=CARTESIAN_POINT ( 'NONE',  ( 25.02538947966649729, 140.2588485512474392, -10.30263013689336304 ) ) ;
#9024=EDGE_LOOP ( 'NONE', ( #14639, #7957, #15699, #6494 ) ) ;
#9026=CIRCLE ( 'NONE', #7893, 2.500000000000002220 ) ;
#9029=DIRECTION ( 'NONE',  ( -1.000000000000000000, -0.000000000000000000, 0.000000000000000000 ) ) ;
#9031=DIRECTION ( 'NONE',  ( 0.000000000000000000, 0.000000000000000000, 1.000000000000000000 ) ) ;
#9033=DIRECTION ( 'NONE',  ( -1.000000000000000000, -0.000000000000000000, 0.000000000000000000 ) ) ;
#9034=DIRECTION ( 'NONE',  ( -1.000000000000000000, -0.000000000000000000, 0.000000000000000000 ) ) ;
#9036=PLANE ( 'NONE',  #2214 ) ;
#9042=VERTEX_POINT ( 'NONE', #8185 ) ;
#9048=EDGE_CURVE ( 'NONE', #17253, #16339, #10667, .T. ) ;
#9049=CIRCLE ( 'NONE', #10453, 33.00000000000000000 ) ;
#9054=CARTESIAN_POINT ( 'NONE',  ( -17.19488518268993715, 32.09742631896689602, -9.330173263366075886 ) ) ;
#9055=CARTESIAN_POINT ( 'NONE',  ( -27.98221281347032274, 18.00000000000000000, -4.999999999999996447 ) ) ;
#9057=CARTESIAN_POINT ( 'NONE',  ( -24.99999999999999645, 120.0000000000000284, -4.999999999999999112 ) ) ;
#9060=DIRECTION ( 'NONE',  ( 1.000000000000000000, 0.000000000000000000, -0.000000000000000000 ) ) ;
#9061=AXIS2_PLACEMENT_3D ( 'NONE', #2882, #227, #7046 ) ;
#9062=ORIENTED_EDGE ( 'NONE', *, *, #12167, .F. ) ;
#9063=VERTEX_POINT ( 'NONE', #14655 ) ;
#9065=CARTESIAN_POINT ( 'NONE',  ( -73.01962815379008020, 149.3990418665993332, -24.40116746791568758 ) ) ;
#9066=EDGE_LOOP ( 'NONE', ( #756, #15028, #7686, #8247 ) ) ;
#9071=LINE ( 'NONE', #16733, #11774 ) ;
#9074=DIRECTION ( 'NONE',  ( 0.000000000000000000, 1.000000000000000000, 0.000000000000000000 ) ) ;
#9075=CARTESIAN_POINT ( 'NONE',  ( 17.53512989260226362, 29.96507997281579350, -14.66107963853301399 ) ) ;
#9076=DIRECTION ( 'NONE',  ( -1.000000000000000000, 0.000000000000000000, 0.000000000000000000 ) ) ;
#9078=CARTESIAN_POINT ( 'NONE',  ( 39.99999999999998579, 20.00000000000000000, -30.00000000000001066 ) ) ;
#9079=ORIENTED_EDGE ( 'NONE', *, *, #14638, .T. ) ;
#9084=ORIENTED_EDGE ( 'NONE', *, *, #11698, .T. ) ;
#9088=( NAMED_UNIT ( * ) PLANE_ANGLE_UNIT ( ) SI_UNIT ( $, .RADIAN. ) );
#9091=CARTESIAN_POINT ( 'NONE',  ( -74.65470611475511475, 143.8751093726684473, -21.33821933965574758 ) ) ;
#9092=DIRECTION ( 'NONE',  ( 1.000000000000000000, 0.000000000000000000, 0.000000000000000000 ) ) ;
#9093=VERTEX_POINT ( 'NONE', #14749 ) ;
#9097=CARTESIAN_POINT ( 'NONE',  ( 24.50594157886344959, 199.0592542586747697, -21.73717956246133909 ) ) ;
#9099=EDGE_LOOP ( 'NONE', ( #9887, #7476 ) ) ;
#9101=VERTEX_POINT ( 'NONE', #1285 ) ;
#9103=CARTESIAN_POINT ( 'NONE',  ( 18.30724418481576166, 140.7653321920888345, -16.52022657272140904 ) ) ;
#9104=ORIENTED_EDGE ( 'NONE', *, *, #9353, .T. ) ;
#9105=DIRECTION ( 'NONE',  ( -1.000000000000000000, 0.000000000000000000, 0.000000000000000000 ) ) ;
#9106=CARTESIAN_POINT ( 'NONE',  ( 8.431728255697246155, 133.2562109147605156, -12.71722808757355949 ) ) ;
#9107=EDGE_CURVE ( 'NONE', #5512, #8410, #15588, .T. ) ;
#9108=ORIENTED_EDGE ( 'NONE', *, *, #16711, .T. ) ;
#9109=CARTESIAN_POINT ( 'NONE',  ( 30.00000000000000355, 196.6227766016838245, -16.00000000000000000 ) ) ;
#9111=EDGE_CURVE ( 'NONE', #1757, #7915, #6787, .T. ) ;
#9115=DIRECTION ( 'NONE',  ( -1.000000000000000000, 0.000000000000000000, 0.000000000000000000 ) ) ;
#9117=CYLINDRICAL_SURFACE ( 'NONE', #7751, 2.500000000000000444 ) ;
#9118=FACE_OUTER_BOUND ( 'NONE', #6507, .T. ) ;
#9121=ORIENTED_EDGE ( 'NONE', *, *, #7691, .F. ) ;
#9123=CARTESIAN_POINT ( 'NONE',  ( -13.90980987654338286, 18.00000000000000355, -23.98326992096529864 ) ) ;
#9132=CARTESIAN_POINT ( 'NONE',  ( 27.72043220849692702, 189.4719557769681444, -27.75644086540374644 ) ) ;
#9134=CARTESIAN_POINT ( 'NONE',  ( -14.45029498972267668, 32.22448475281832003, -9.930813566224275135 ) ) ;
#9137=EDGE_CURVE ( 'NONE', #8198, #5744, #5129, .T. ) ;
#9139=ADVANCED_FACE ( 'NONE', ( #13332, #5367, #16344 ), #12182, .F. ) ;
#9141=CARTESIAN_POINT ( 'NONE',  ( 34.31461291909280220, 192.4344680579923761, -28.14280641908791480 ) ) ;
#9142=CARTESIAN_POINT ( 'NONE',  ( -85.59781103574918859, 201.6348411963793410, -13.74530841833676220 ) ) ;
#9146=CARTESIAN_POINT ( 'NONE',  ( -82.79368516360898411, 153.6052450214444605, -27.64877209012308867 ) ) ;
#9153=CARTESIAN_POINT ( 'NONE',  ( 39.99999999999999289, 20.00000000000000000, 0.000000000000000000 ) ) ;
#9157=EDGE_LOOP ( 'NONE', ( #11222, #8156, #3536, #4578, #1363 ) ) ;
#9160=EDGE_CURVE ( 'NONE', #8796, #11521, #17007, .T. ) ;
#9161=EDGE_CURVE ( 'NONE', #8531, #8768, #1734, .T. ) ;
#9163=FACE_OUTER_BOUND ( 'NONE', #6211, .T. ) ;
#9165=CARTESIAN_POINT ( 'NONE',  ( -27.84784281930893357, 19.99999999999999645, -7.647248539284095870 ) ) ;
#9167=VERTEX_POINT ( 'NONE', #9770 ) ;
#9181=ORIENTED_EDGE ( 'NONE', *, *, #11547, .F. ) ;
#9182=DIRECTION ( 'NONE',  ( 1.000000000000000000, 0.000000000000000000, 0.000000000000000000 ) ) ;
#9185=CARTESIAN_POINT ( 'NONE',  ( -82.50000000000002842, 146.6227766016838245, 1.387778780781445676E-14 ) ) ;
#9186=AXIS2_PLACEMENT_3D ( 'NONE', #5196, #14582, #1040 ) ;
#9187=CIRCLE ( 'NONE', #4955, 5.000000000000004441 ) ;
#9189=ORIENTED_EDGE ( 'NONE', *, *, #14906, .F. ) ;
#9191=LINE ( 'NONE', #13361, #12924 ) ;
#9193=CARTESIAN_POINT ( 'NONE',  ( -85.14000932857697990, 149.7234947166294603, -27.30319596934542048 ) ) ;
#9194=CARTESIAN_POINT ( 'NONE',  ( 21.38051303318334462, 141.6185065902053282, -13.74313897096208414 ) ) ;
#9195=ORIENTED_EDGE ( 'NONE', *, *, #11943, .T. ) ;
#9198=VECTOR ( 'NONE', #2171, 1000.000000000000000 ) ;
#9201=EDGE_CURVE ( 'NONE', #6832, #5595, #9859, .T. ) ;
#9202=VECTOR ( 'NONE', #16430, 1000.000000000000000 ) ;
#9203=DIRECTION ( 'NONE',  ( 1.000000000000000000, 0.000000000000000000, 0.000000000000000000 ) ) ;
#9204=CARTESIAN_POINT ( 'NONE',  ( 22.88332935572807969, 29.84310215611307271, -6.048604702147989620 ) ) ;
#9206=CARTESIAN_POINT ( 'NONE',  ( -23.00000000000000000, 120.0000000000000284, -15.00000000000000000 ) ) ;
#9209=CARTESIAN_POINT ( 'NONE',  ( 16.97539380423070909, 126.5649914159620266, -7.928130581088665529 ) ) ;
#9215=VECTOR ( 'NONE', #10477, 1000.000000000000000 ) ;
#9217=CARTESIAN_POINT ( 'NONE',  ( -80.00000000000002842, 146.6227766016838245, -16.00000000000000000 ) ) ;
#9221=VERTEX_POINT ( 'NONE', #4561 ) ;
#9222=CARTESIAN_POINT ( 'NONE',  ( -27.99999999999998224, 10.00000000000000000, -35.00200000000000244 ) ) ;
#9224=VECTOR ( 'NONE', #4188, 1000.000000000000000 ) ;
#9225=CARTESIAN_POINT ( 'NONE',  ( 27.99239453806529099, 189.3908747183072592, -27.80828541846619828 ) ) ;
#9227=AXIS2_PLACEMENT_3D ( 'NONE', #12133, #7966, #1153 ) ;
#9228=CARTESIAN_POINT ( 'NONE',  ( -20.86241502029199424, 18.00000000000000000, -20.14618526197082460 ) ) ;
#9229=AXIS2_PLACEMENT_3D ( 'NONE', #14091, #631, #7606 ) ;
#9233=CARTESIAN_POINT ( 'NONE',  ( 26.63661590110499233, 191.6363561590497966, -28.71510896997970264 ) ) ;
#9237=ORIENTED_EDGE ( 'NONE', *, *, #12954, .T. ) ;
#9240=CARTESIAN_POINT ( 'NONE',  ( -78.54584381417873828, 153.9859494455611468, -27.89172594985639364 ) ) ;
#9241=( GEOMETRIC_REPRESENTATION_CONTEXT ( 3 ) GLOBAL_UNCERTAINTY_ASSIGNED_CONTEXT ( ( #17426 ) ) GLOBAL_UNIT_ASSIGNED_CONTEXT ( ( #3157, #16874, #9789 ) ) REPRESENTATION_CONTEXT ( 'NONE', 'WORKASPACE' ) );
#9247=CARTESIAN_POINT ( 'NONE',  ( 24.02490146132329940, 147.2612100285404608, -25.13395616064557103 ) ) ;
#9248=DIRECTION ( 'NONE',  ( 1.000000000000000000, 0.000000000000000000, 0.000000000000000000 ) ) ;
#9253=AXIS2_PLACEMENT_3D ( 'NONE', #939, #2537, #9074 ) ;
#9257=FACE_OUTER_BOUND ( 'NONE', #2315, .T. ) ;
#9259=CARTESIAN_POINT ( 'NONE',  ( 34.93420767853316988, 20.00000000000000000, -15.00000000000000000 ) ) ;
#9264=EDGE_CURVE ( 'NONE', #12122, #2736, #2019, .T. ) ;
#9265=EDGE_CURVE ( 'NONE', #8108, #4701, #5976, .T. ) ;
#9271=LINE ( 'NONE', #5292, #2503 ) ;
#9277=CARTESIAN_POINT ( 'NONE',  ( 35.99999999999999289, 196.9987679943316721, -24.11115281963766321 ) ) ;
#9279=CIRCLE ( 'NONE', #15516, 5.000000000000004441 ) ;
#9281=CARTESIAN_POINT ( 'NONE',  ( 8.904477399772744661, 142.4465447428235620, -19.33413753149157088 ) ) ;
#9283=DIRECTION ( 'NONE',  ( -1.000000000000000000, -0.000000000000000000, 0.000000000000000000 ) ) ;
#9284=CARTESIAN_POINT ( 'NONE',  ( 14.44088586081352688, 138.6571688462224472, -6.678806037552732278 ) ) ;
#9288=DIRECTION ( 'NONE',  ( 0.000000000000000000, 0.000000000000000000, -1.000000000000000000 ) ) ;
#9295=CARTESIAN_POINT ( 'NONE',  ( 34.26467700469002153, 18.00000000000000000, -10.17319632352554137 ) ) ;
#9296=CARTESIAN_POINT ( 'NONE',  ( -7.379000772445021283, 30.00000000000000000, -25.00000000000000000 ) ) ;
#9299=DIRECTION ( 'NONE',  ( -0.000000000000000000, -0.000000000000000000, -1.000000000000000000 ) ) ;
#9303=DIRECTION ( 'NONE',  ( -0.000000000000000000, -0.000000000000000000, -1.000000000000000000 ) ) ;
#9312=LINE ( 'NONE', #1083, #11015 ) ;
#9313=VERTEX_POINT ( 'NONE', #15174 ) ;
#9314=CARTESIAN_POINT ( 'NONE',  ( -30.49999999999998224, 10.00000000000000000, -16.00000000000000000 ) ) ;
#9315=CARTESIAN_POINT ( 'NONE',  ( 22.74907522843311369, 194.6587679740005115, -23.63587233142071042 ) ) ;
#9316=AXIS2_PLACEMENT_3D ( 'NONE', #11842, #15743, #14503 ) ;
#9318=CARTESIAN_POINT ( 'NONE',  ( -19.80886414215282798, 18.00000000000000000, -20.97268729564153489 ) ) ;
#9323=CARTESIAN_POINT ( 'NONE',  ( -76.45654094002816237, 190.0067896460675740, -27.40528370530127233 ) ) ;
#9326=VERTEX_POINT ( 'NONE', #16777 ) ;
#9327=ORIENTED_EDGE ( 'NONE', *, *, #8606, .T. ) ;
#9330=AXIS2_PLACEMENT_3D ( 'NONE', #684, #2090, #2351 ) ;
#9334=VERTEX_POINT ( 'NONE', #8713 ) ;
#9336=DIRECTION ( 'NONE',  ( -0.000000000000000000, -0.000000000000000000, -1.000000000000000000 ) ) ;
#9339=EDGE_CURVE ( 'NONE', #10807, #1310, #14278, .T. ) ;
#9340=CARTESIAN_POINT ( 'NONE',  ( 24.44272481504117778, 148.9119151679986430, -26.63478011418836644 ) ) ;
#9345=AXIS2_PLACEMENT_3D ( 'NONE', #7363, #11153, #12498 ) ;
#9346=CARTESIAN_POINT ( 'NONE',  ( 19.36310082087489803, 29.94084738964976111, -13.97143931599698874 ) ) ;
#9348=DIRECTION ( 'NONE',  ( -1.000000000000000000, 0.000000000000000000, 2.312964634635742464E-16 ) ) ;
#9353=EDGE_CURVE ( 'NONE', #14104, #6709, #11581, .T. ) ;
#9355=CYLINDRICAL_SURFACE ( 'NONE', #13876, 20.00000000000000355 ) ;
#9359=EDGE_LOOP ( 'NONE', ( #8639, #37, #1732, #14874 ) ) ;
#9361=CARTESIAN_POINT ( 'NONE',  ( 16.23725950538872809, 18.00000000000000000, -24.99999999982344789 ) ) ;
#9362=CARTESIAN_POINT ( 'NONE',  ( -84.32132260856947426, 142.4452037501735902, -19.33642647557002192 ) ) ;
#9363=CARTESIAN_POINT ( 'NONE',  ( 30.00000000000001066, 146.6227766016838245, -35.00200000000000244 ) ) ;
#9364=ORIENTED_EDGE ( 'NONE', *, *, #11493, .F. ) ;
#9371=EDGE_CURVE ( 'NONE', #8437, #10436, #11536, .T. ) ;
#9373=ORIENTED_EDGE ( 'NONE', *, *, #5274, .T. ) ;
#9374=CARTESIAN_POINT ( 'NONE',  ( 16.26529498815335373, 136.8354558863973409, -4.782531348471686705 ) ) ;
#9376=CARTESIAN_POINT ( 'NONE',  ( -85.77867439187610898, 148.2463666031633238, -26.04982723689806434 ) ) ;
#9377=CARTESIAN_POINT ( 'NONE',  ( 25.87766738269754541, 139.8661988410599406, -8.984976992518891592 ) ) ;
#9381=DIRECTION ( 'NONE',  ( -1.000000000000000000, -0.000000000000000000, 0.000000000000000000 ) ) ;
#9382=DIRECTION ( 'NONE',  ( 1.000000000000000000, 0.000000000000000000, 0.000000000000000000 ) ) ;
#9384=CARTESIAN_POINT ( 'NONE',  ( 28.14717441101696593, 18.00000000000000000, -20.07001214884044415 ) ) ;
#9385=DIRECTION ( 'NONE',  ( 1.000000000000000000, 0.000000000000000000, 0.000000000000000000 ) ) ;
#9387=LINE ( 'NONE', #8144, #13860 ) ;
#9388=CARTESIAN_POINT ( 'NONE',  ( -95.00000000000000000, 171.6227766016838245, 0.000000000000000000 ) ) ;
#9392=VERTEX_POINT ( 'NONE', #17108 ) ;
#9395=EDGE_LOOP ( 'NONE', ( #1933, #8110 ) ) ;
#9396=CYLINDRICAL_SURFACE ( 'NONE', #10002, 2.500000000000002220 ) ;
#9400=ORIENTED_EDGE ( 'NONE', *, *, #6199, .T. ) ;
#9401=FACE_OUTER_BOUND ( 'NONE', #2518, .T. ) ;
#9402=CARTESIAN_POINT ( 'NONE',  ( -95.00000000000000000, 171.6227766016838245, -27.69059892324149530 ) ) ;
#9403=DIRECTION ( 'NONE',  ( -1.000000000000000000, -0.000000000000000000, 0.000000000000000000 ) ) ;
#9404=CARTESIAN_POINT ( 'NONE',  ( -3.000000000000000888, 154.3022685259950038, -9.999999999999900524 ) ) ;
#9405=ADVANCED_FACE ( 'NONE', ( #6304, #3746 ), #7636, .F. ) ;
#9409=CARTESIAN_POINT ( 'NONE',  ( -87.25092477156692894, 194.6587679740005115, -23.63587233142071042 ) ) ;
#9410=CARTESIAN_POINT ( 'NONE',  ( -87.20996884815647832, 198.7539484232961513, -18.80562413441371206 ) ) ;
#9412=ORIENTED_EDGE ( 'NONE', *, *, #17363, .T. ) ;
#9414=DIRECTION ( 'NONE',  ( -1.000000000000000000, 0.000000000000000000, 0.000000000000000000 ) ) ;
#9415=ORIENTED_EDGE ( 'NONE', *, *, #10825, .F. ) ;
#9420=DIRECTION ( 'NONE',  ( 1.000000000000000000, 0.000000000000000000, 0.000000000000000000 ) ) ;
#9422=EDGE_CURVE ( 'NONE', #8896, #14332, #16453, .T. ) ;
#9424=CARTESIAN_POINT ( 'NONE',  ( -84.06062570790729183, 201.0559264674919291, -18.94433901724533342 ) ) ;
#9430=EDGE_CURVE ( 'NONE', #2922, #1718, #7109, .T. ) ;
#9431=DIRECTION ( 'NONE',  ( 0.000000000000000000, 0.000000000000000000, 1.000000000000000000 ) ) ;
#9433=DIRECTION ( 'NONE',  ( -1.000000000000000000, -0.000000000000000000, 0.000000000000000000 ) ) ;
#9435=FACE_OUTER_BOUND ( 'NONE', #14140, .T. ) ;
#9437=CARTESIAN_POINT ( 'NONE',  ( -86.00000000000002842, 146.6227766016838245, -24.49489742783179480 ) ) ;
#9441=DIRECTION ( 'NONE',  ( 1.000000000000000000, 0.000000000000000000, -0.000000000000000000 ) ) ;
#9442=CARTESIAN_POINT ( 'NONE',  ( -34.99999999999999289, 122.0000000000000284, -4.999999999999999112 ) ) ;
#9443=CARTESIAN_POINT ( 'NONE',  ( 35.96514256823365940, 197.3601060891146517, -23.72478281133074773 ) ) ;
#9446=CARTESIAN_POINT ( 'NONE',  ( 16.64812168497169864, 126.9869021000460663, -8.626120676703536105 ) ) ;
#9447=AXIS2_PLACEMENT_3D ( 'NONE', #3384, #9034, #14264 ) ;
#9449=DIRECTION ( 'NONE',  ( 0.000000000000000000, 0.000000000000000000, 1.000000000000000000 ) ) ;
#9450=DIRECTION ( 'NONE',  ( -0.000000000000000000, -0.000000000000000000, 1.000000000000000000 ) ) ;
#9451=EDGE_LOOP ( 'NONE', ( #7283, #4316, #17367, #13968, #3166, #17280, #2525, #7006, #15250, #6957, #6154, #5754, #6405, #8298, #5175 ) ) ;
#9453=CARTESIAN_POINT ( 'NONE',  ( -85.41098039551273757, 194.0039740083362858, -26.91197613625889673 ) ) ;
#9454=CARTESIAN_POINT ( 'NONE',  ( 17.00000000000000000, 191.6227766016837961, 1.224646799147353454E-15 ) ) ;
#9456=CARTESIAN_POINT ( 'NONE',  ( 30.00000000000001066, 146.6227766016838245, -12.99999999999999822 ) ) ;
#9457=CARTESIAN_POINT ( 'NONE',  ( 29.98123639043839006, 18.00000000000000000, -18.19121573219640098 ) ) ;
#9459=CARTESIAN_POINT ( 'NONE',  ( 19.20424459521615290, 18.00000000000228439, -11.86908137778077688 ) ) ;
#9460=CARTESIAN_POINT ( 'NONE',  ( 34.93420767853318409, 30.00000000000000000, -5.000000000000010658 ) ) ;
#9464=CARTESIAN_POINT ( 'NONE',  ( 24.26049027360500432, 144.8396561671642360, -22.53731575973597501 ) ) ;
#9466=DIRECTION ( 'NONE',  ( -1.000000000000000000, -0.000000000000000000, 0.000000000000000000 ) ) ;
#9467=VERTEX_POINT ( 'NONE', #10549 ) ;
#9468=FACE_OUTER_BOUND ( 'NONE', #17344, .T. ) ;
#9470=ORIENTED_EDGE ( 'NONE', *, *, #9430, .F. ) ;
#9477=AXIS2_PLACEMENT_3D ( 'NONE', #7144, #14058, #13890 ) ;
#9480=EDGE_CURVE ( 'NONE', #10541, #7474, #14344, .T. ) ;
#9481=EDGE_CURVE ( 'NONE', #14947, #9019, #15957, .T. ) ;
#9482=EDGE_CURVE ( 'NONE', #6730, #7936, #8807, .T. ) ;
#9484=CARTESIAN_POINT ( 'NONE',  ( 34.46470488465457294, 190.5906835324045119, -27.00480063125523600 ) ) ;
#9491=ORIENTED_EDGE ( 'NONE', *, *, #14606, .T. ) ;
#9492=CARTESIAN_POINT ( 'NONE',  ( 48.00000000000000711, 191.6227766016837677, -5.571800142134975431 ) ) ;
#9499=CIRCLE ( 'NONE', #452, 2.499999999999998668 ) ;
#9502=FACE_OUTER_BOUND ( 'NONE', #11357, .T. ) ;
#9503=VECTOR ( 'NONE', #9780, 1000.000000000000000 ) ;
#9504=DIRECTION ( 'NONE',  ( -0.000000000000000000, -0.000000000000000000, -1.000000000000000000 ) ) ;
#9505=CARTESIAN_POINT ( 'NONE',  ( 21.87945022329474298, 29.86245334106958538, -9.005757899690800983 ) ) ;
#9510=CARTESIAN_POINT ( 'NONE',  ( -87.50000000000004263, 196.6227766016838245, -13.00000000000000000 ) ) ;
#9511=CARTESIAN_POINT ( 'NONE',  ( 14.93242934743711992, 20.00000000000000000, -25.00000000000000000 ) ) ;
#9514=CIRCLE ( 'NONE', #1891, 747.9999999999998863 ) ;
#9518=AXIS2_PLACEMENT_3D ( 'NONE', #1497, #16283, #10867 ) ;
#9520=EDGE_CURVE ( 'NONE', #874, #1820, #5413, .T. ) ;
#9523=CARTESIAN_POINT ( 'NONE',  ( -22.93725393319379435, 100.0000000000000142, -6.000000000000000000 ) ) ;
#9524=ORIENTED_EDGE ( 'NONE', *, *, #11054, .F. ) ;
#9525=CARTESIAN_POINT ( 'NONE',  ( 17.56954167074719919, 125.3114906870353167, -3.338394383324010395 ) ) ;
#9526=DIRECTION ( 'NONE',  ( 0.000000000000000000, 0.000000000000000000, 1.000000000000000000 ) ) ;
#9529=EDGE_CURVE ( 'NONE', #16965, #3735, #14729, .T. ) ;
#9531=ORIENTED_EDGE ( 'NONE', *, *, #15171, .T. ) ;
#9532=EDGE_CURVE ( 'NONE', #3735, #15620, #11060, .T. ) ;
#9534=DIRECTION ( 'NONE',  ( 1.000000000000000000, 0.000000000000000000, 0.000000000000000000 ) ) ;
#9537=CARTESIAN_POINT ( 'NONE',  ( -40.00000000000000000, 20.00000000000000000, -30.00000000000000355 ) ) ;
#9541=CARTESIAN_POINT ( 'NONE',  ( 27.42233521511133887, 138.9393305618597481, -4.670371664028303726 ) ) ;
#9542=ORIENTED_EDGE ( 'NONE', *, *, #15204, .T. ) ;
#9544=DIRECTION ( 'NONE',  ( 0.000000000000000000, 0.000000000000000000, -1.000000000000000000 ) ) ;
#9547=EDGE_CURVE ( 'NONE', #13466, #11970, #10739, .T. ) ;
#9548=CARTESIAN_POINT ( 'NONE',  ( 34.93420767853316988, 18.00000000000000355, -4.999999999999999112 ) ) ;
#9549=ADVANCED_FACE ( 'NONE', ( #3836 ), #13579, .F. ) ;
#9550=CARTESIAN_POINT ( 'NONE',  ( 17.52334770333193248, 18.00000000000227018, -12.62810114740270606 ) ) ;
#9554=LINE ( 'NONE', #14960, #3401 ) ;
#9557=EDGE_LOOP ( 'NONE', ( #1580, #14889 ) ) ;
#9558=CARTESIAN_POINT ( 'NONE',  ( 17.54349574104648823, 125.4948194589026684, -4.999999999999997335 ) ) ;
#9562=EDGE_CURVE ( 'NONE', #11405, #6602, #12159, .T. ) ;
#9563=ORIENTED_EDGE ( 'NONE', *, *, #14841, .T. ) ;
#9565=CARTESIAN_POINT ( 'NONE',  ( -725.0000000000000000, 30.00000000000000000, -25.00000000000000000 ) ) ;
#9568=CARTESIAN_POINT ( 'NONE',  ( 26.45654094002815526, 153.2387635573001319, -27.40528370530127233 ) ) ;
#9569=AXIS2_PLACEMENT_3D ( 'NONE', #9964, #5997, #11560 ) ;
#9572=CARTESIAN_POINT ( 'NONE',  ( -725.0000000000000000, 19.99999999999995737, -13.00000000000000000 ) ) ;
#9575=DIRECTION ( 'NONE',  ( 0.000000000000000000, 0.000000000000000000, 1.000000000000000000 ) ) ;
#9576=EDGE_LOOP ( 'NONE', ( #8245, #6179, #9706, #5895 ) ) ;
#9581=AXIS2_PLACEMENT_3D ( 'NONE', #6785, #1729, #5712 ) ;
#9585=CARTESIAN_POINT ( 'NONE',  ( -16.17053951239850207, 32.72994544565565889, -6.425226171708652956 ) ) ;
#9588=EDGE_CURVE ( 'NONE', #1561, #16968, #12237, .T. ) ;
#9592=CIRCLE ( 'NONE', #5931, 35.00000000000000000 ) ;
#9599=DIRECTION ( 'NONE',  ( -0.000000000000000000, -0.000000000000000000, 1.000000000000000000 ) ) ;
#9602=CARTESIAN_POINT ( 'NONE',  ( -76.84835529096334028, 201.7321575960915538, -17.84571802696395082 ) ) ;
#9607=VECTOR ( 'NONE', #13426, 1000.000000000000000 ) ;
#9614=EDGE_LOOP ( 'NONE', ( #13350, #2686 ) ) ;
#9618=DIRECTION ( 'NONE',  ( -1.337133840571206485E-16, 0.000000000000000000, -1.000000000000000000 ) ) ;
#9624=CARTESIAN_POINT ( 'NONE',  ( -80.00000000000001421, 196.6227766016838245, -35.00200000000000244 ) ) ;
#9627=CARTESIAN_POINT ( 'NONE',  ( 26.85584576128377066, 137.3904121345421458, -7.294850950184896377 ) ) ;
#9633=CARTESIAN_POINT ( 'NONE',  ( -50.00000000000000000, 171.6227766016838245, 0.000000000000000000 ) ) ;
#9637=CARTESIAN_POINT ( 'NONE',  ( 48.00000000000000711, 187.6227766016837961, -12.50000337241049309 ) ) ;
#9639=DIRECTION ( 'NONE',  ( -1.000000000000000000, 0.000000000000000000, 0.000000000000000000 ) ) ;
#9640=DIRECTION ( 'NONE',  ( 0.000000000000000000, 0.000000000000000000, 1.000000000000000000 ) ) ;
#9643=ORIENTED_EDGE ( 'NONE', *, *, #3823, .F. ) ;
#9644=CARTESIAN_POINT ( 'NONE',  ( -11.18069906337402664, 30.84474844633047397, -14.38199110044527274 ) ) ;
#9646=CARTESIAN_POINT ( 'NONE',  ( 24.67949051125555826, 29.87169671703155771, -7.269639412668861489 ) ) ;
#9649=ORIENTED_EDGE ( 'NONE', *, *, #7974, .F. ) ;
#9653=LINE ( 'NONE', #1516, #17210 ) ;
#9655=CARTESIAN_POINT ( 'NONE',  ( 33.81731182140757852, 153.1022248993912171, -27.31438289289431864 ) ) ;
#9658=DIRECTION ( 'NONE',  ( 0.000000000000000000, 0.000000000000000000, 1.000000000000000000 ) ) ;
#9664=DIRECTION ( 'NONE',  ( 0.000000000000000000, 0.000000000000000000, 1.000000000000000000 ) ) ;
#9665=ORIENTED_EDGE ( 'NONE', *, *, #9160, .T. ) ;
#9666=CARTESIAN_POINT ( 'NONE',  ( -86.08081429761091385, 192.2260612991243534, -25.77925661938086677 ) ) ;
#9667=LINE ( 'NONE', #15153, #12621 ) ;
#9669=ORIENTED_EDGE ( 'NONE', *, *, #3638, .T. ) ;
#9671=DIRECTION ( 'NONE',  ( 0.000000000000000000, 0.000000000000000000, 1.000000000000000000 ) ) ;
#9672=CARTESIAN_POINT ( 'NONE',  ( -72.94847233519770668, 199.2234891967518422, -18.10843944793621674 ) ) ;
#9677=FACE_OUTER_BOUND ( 'NONE', #8082, .T. ) ;
#9679=ADVANCED_FACE ( 'NONE', ( #5858 ), #12321, .F. ) ;
#9680=DIRECTION ( 'NONE',  ( -1.000000000000000000, 0.000000000000000000, 0.000000000000000000 ) ) ;
#9685=CARTESIAN_POINT ( 'NONE',  ( -86.00000000000004263, 196.8086972563010022, -24.30514295430833371 ) ) ;
#9686=CARTESIAN_POINT ( 'NONE',  ( -2.428612866367531510E-15, 2.000000000000000000, -28.00000000000000711 ) ) ;
#9688=DIRECTION ( 'NONE',  ( -1.000000000000000000, -6.938893903907228378E-16, -0.000000000000000000 ) ) ;
#9689=CYLINDRICAL_SURFACE ( 'NONE', #10060, 5.000000000000018652 ) ;
#9691=VERTEX_POINT ( 'NONE', #16672 ) ;
#9692=CARTESIAN_POINT ( 'NONE',  ( -15.00000000000002132, 100.0000000000000142, -4.999999999999999112 ) ) ;
#9693=EDGE_LOOP ( 'NONE', ( #10222, #4745 ) ) ;
#9696=PRESENTATION_STYLE_ASSIGNMENT (( #16187 ) ) ;
#9698=DIRECTION ( 'NONE',  ( -1.000000000000000000, -0.000000000000000000, 0.000000000000000000 ) ) ;
#9700=EDGE_CURVE ( 'NONE', #1100, #7826, #13741, .T. ) ;
#9706=ORIENTED_EDGE ( 'NONE', *, *, #7461, .T. ) ;
#9712=CARTESIAN_POINT ( 'NONE',  ( 14.91849273675205545, 128.9263856399286396, -11.14803070335530855 ) ) ;
#9715=CARTESIAN_POINT ( 'NONE',  ( 26.76721132277178228, 139.3994271089711958, -7.121518580654788266 ) ) ;
#9718=CYLINDRICAL_SURFACE ( 'NONE', #1135, 12.00000000000000000 ) ;
#9722=CARTESIAN_POINT ( 'NONE',  ( 25.49999999999998579, 9.999999999999998224, -16.00000000000000000 ) ) ;
#9727=DIRECTION ( 'NONE',  ( 1.000000000000000000, 0.000000000000000000, 0.000000000000000000 ) ) ;
#9729=VERTEX_POINT ( 'NONE', #11078 ) ;
#9735=CARTESIAN_POINT ( 'NONE',  ( -95.00000000000000000, 171.6227766016838245, -30.00000000000000000 ) ) ;
#9737=EDGE_CURVE ( 'NONE', #4814, #730, #12677, .T. ) ;
#9738=CARTESIAN_POINT ( 'NONE',  ( 22.50701606102701646, 147.0010062438373382, -21.97388680505720515 ) ) ;
#9740=AXIS2_PLACEMENT_3D ( 'NONE', #9404, #16494, #16233 ) ;
#9743=DIRECTION ( 'NONE',  ( -1.000000000000000000, 0.000000000000000000, 0.000000000000000000 ) ) ;
#9749=CARTESIAN_POINT ( 'NONE',  ( 17.00000000000000000, 171.6227766016838245, -20.00000000000000355 ) ) ;
#9750=EDGE_LOOP ( 'NONE', ( #16334, #468 ) ) ;
#9758=AXIS2_PLACEMENT_3D ( 'NONE', #15314, #14084, #4521 ) ;
#9767=DIRECTION ( 'NONE',  ( 0.000000000000000000, 0.000000000000000000, 1.000000000000000000 ) ) ;
#9769=FACE_OUTER_BOUND ( 'NONE', #3128, .T. ) ;
#9770=CARTESIAN_POINT ( 'NONE',  ( -34.99999999999999289, 120.0000000000000000, 0.000000000000000000 ) ) ;
#9774=ADVANCED_FACE ( 'NONE', ( #6648 ), #11952, .T. ) ;
#9775=ORIENTED_EDGE ( 'NONE', *, *, #3798, .F. ) ;
#9780=DIRECTION ( 'NONE',  ( 0.000000000000000000, -1.000000000000000000, -6.123233995736762338E-17 ) ) ;
#9782=ORIENTED_EDGE ( 'NONE', *, *, #15742, .F. ) ;
#9786=ADVANCED_FACE ( 'NONE', ( #17354 ), #2484, .F. ) ;
#9788=ORIENTED_EDGE ( 'NONE', *, *, #2294, .F. ) ;
#9789=( NAMED_UNIT ( * ) SI_UNIT ( $, .STERADIAN. ) SOLID_ANGLE_UNIT ( ) );
#9790=ORIENTED_EDGE ( 'NONE', *, *, #7490, .T. ) ;
#9793=DIRECTION ( 'NONE',  ( 1.000000000000000000, -0.000000000000000000, -0.000000000000000000 ) ) ;
#9794=LINE ( 'NONE', #15194, #14854 ) ;
#9797=VERTEX_POINT ( 'NONE', #3910 ) ;
#9798=CARTESIAN_POINT ( 'NONE',  ( 50.00000000000000000, 171.6227766016838245, 0.000000000000000000 ) ) ;
#9800=VECTOR ( 'NONE', #169, 1000.000000000000000 ) ;
#9806=ADVANCED_FACE ( 'NONE', ( #13291 ), #10622, .T. ) ;
#9809=ORIENTED_EDGE ( 'NONE', *, *, #11106, .T. ) ;
#9810=CYLINDRICAL_SURFACE ( 'NONE', #17152, 7.499999999999996447 ) ;
#9812=CARTESIAN_POINT ( 'NONE',  ( -100.0000000000000000, 134.2062027339443944, -25.00000000000000000 ) ) ;
#9813=CIRCLE ( 'NONE', #15471, 20.00000000000000355 ) ;
#9814=DIRECTION ( 'NONE',  ( -1.000000000000000000, 0.000000000000000000, 0.000000000000000000 ) ) ;
#9815=LINE ( 'NONE', #12559, #9800 ) ;
#9817=CARTESIAN_POINT ( 'NONE',  ( 27.99999999999998224, 9.999999999999998224, -16.00000000000000000 ) ) ;
#9818=DIRECTION ( 'NONE',  ( -1.000000000000000000, -0.000000000000000000, 0.000000000000000000 ) ) ;
#9819=LINE ( 'NONE', #2033, #7916 ) ;
#9820=CARTESIAN_POINT ( 'NONE',  ( 20.49999999999998224, 10.00000000000000000, -13.00000000000000000 ) ) ;
#9821=ORIENTED_EDGE ( 'NONE', *, *, #13803, .T. ) ;
#9823=CARTESIAN_POINT ( 'NONE',  ( 24.93507336697353338, 29.86842105263157521, -5.000000000000004441 ) ) ;
#9831=CARTESIAN_POINT ( 'NONE',  ( 37.47214505283547936, 147.3844239155462503, -22.40167687543584663 ) ) ;
#9832=( BOUNDED_CURVE ( )  B_SPLINE_CURVE ( 3, ( #7852, #11739, #10780, #17241 ),
 .UNSPECIFIED., .F., .F. ) 
 B_SPLINE_CURVE_WITH_KNOTS ( ( 4, 4 ),
 ( 4.712388980384692339, 6.283185307179586232 ),
 .UNSPECIFIED. ) 
 CURVE ( )  GEOMETRIC_REPRESENTATION_ITEM ( )  RATIONAL_B_SPLINE_CURVE ( ( 1.000000000000000000, 0.8047378541243654926, 0.8047378541243654926, 1.000000000000000000 ) ) 
 REPRESENTATION_ITEM ( '' )  );
#9835=AXIS2_PLACEMENT_3D ( 'NONE', #6641, #13368, #12037 ) ;
#9836=DIRECTION ( 'NONE',  ( 0.000000000000000000, -1.000000000000000000, 0.000000000000000000 ) ) ;
#9841=CARTESIAN_POINT ( 'NONE',  ( 30.00000000000000355, 196.6227766016838245, -12.99999999999999822 ) ) ;
#9843=CARTESIAN_POINT ( 'NONE',  ( 11.02544963116560517, 142.2295695439714791, -19.00161275228506952 ) ) ;
#9844=ORIENTED_EDGE ( 'NONE', *, *, #15009, .F. ) ;
#9845=EDGE_CURVE ( 'NONE', #14060, #15553, #6469, .T. ) ;
#9846=CARTESIAN_POINT ( 'NONE',  ( 49.99999999999998579, 179.6227766016838245, -10.00000337241049309 ) ) ;
#9849=ORIENTED_EDGE ( 'NONE', *, *, #5496, .T. ) ;
#9850=ORIENTED_EDGE ( 'NONE', *, *, #4565, .F. ) ;
#9852=CIRCLE ( 'NONE', #11266, 2.500000000000000444 ) ;
#9857=DIRECTION ( 'NONE',  ( 1.000000000000000000, 0.000000000000000000, 0.000000000000000000 ) ) ;
#9859=LINE ( 'NONE', #11278, #15868 ) ;
#9862=DIRECTION ( 'NONE',  ( 1.000000000000000000, 0.000000000000000000, 0.000000000000000000 ) ) ;
#9864=ORIENTED_EDGE ( 'NONE', *, *, #1457, .F. ) ;
#9865=CARTESIAN_POINT ( 'NONE',  ( -76.36507656924925413, 201.4000939832746724, -18.39459910103776963 ) ) ;
#9866=LINE ( 'NONE', #3148, #6815 ) ;
#9868=EDGE_CURVE ( 'NONE', #2736, #8582, #2661, .T. ) ;
#9872=VERTEX_POINT ( 'NONE', #1067 ) ;
#9873=AXIS2_PLACEMENT_3D ( 'NONE', #5471, #246, #9534 ) ;
#9879=DIRECTION ( 'NONE',  ( -1.000000000000000000, 0.000000000000000000, 0.000000000000000000 ) ) ;
#9882=ORIENTED_EDGE ( 'NONE', *, *, #8299, .F. ) ;
#9883=CYLINDRICAL_SURFACE ( 'NONE', #13020, 5.000000000000000888 ) ;
#9887=ORIENTED_EDGE ( 'NONE', *, *, #3616, .T. ) ;
#9888=DIRECTION ( 'NONE',  ( -1.000000000000000000, -0.000000000000000000, 0.000000000000000000 ) ) ;
#9889=CIRCLE ( 'NONE', #9316, 27.69059892324149530 ) ;
#9890=PLANE ( 'NONE',  #14136 ) ;
#9891=EDGE_CURVE ( 'NONE', #15022, #13094, #8745, .T. ) ;
#9893=FACE_OUTER_BOUND ( 'NONE', #11821, .T. ) ;
#9896=AXIS2_PLACEMENT_3D ( 'NONE', #12103, #15091, #17410 ) ;
#9897=AXIS2_PLACEMENT_3D ( 'NONE', #5913, #11308, #16723 ) ;
#9901=VECTOR ( 'NONE', #12540, 1000.000000000000000 ) ;
#9902=DIRECTION ( 'NONE',  ( 0.000000000000000000, 1.000000000000000000, 0.000000000000000000 ) ) ;
#9903=FACE_OUTER_BOUND ( 'NONE', #15596, .T. ) ;
#9907=ADVANCED_FACE ( 'NONE', ( #12220 ), #8142, .F. ) ;
#9914=CARTESIAN_POINT ( 'NONE',  ( 24.93507336697333798, 29.86842105264641845, -5.660862367392566874 ) ) ;
#9915=CIRCLE ( 'NONE', #2282, 10.00000000000000178 ) ;
#9916=CARTESIAN_POINT ( 'NONE',  ( 24.75325409605274274, 140.3706687641101212, -10.61653890585399296 ) ) ;
#9917=ORIENTED_EDGE ( 'NONE', *, *, #373, .F. ) ;
#9919=CARTESIAN_POINT ( 'NONE',  ( 49.99999999999998579, 171.6227766016838245, -15.00000337241049131 ) ) ;
#9921=CARTESIAN_POINT ( 'NONE',  ( 22.65335638526122963, 148.1846496461902234, -23.23759988234781204 ) ) ;
#9925=DIRECTION ( 'NONE',  ( 1.224646799147353207E-16, 1.000000000000000000, 0.000000000000000000 ) ) ;
#9930=LINE ( 'NONE', #15060, #709 ) ;
#9936=CARTESIAN_POINT ( 'NONE',  ( -80.00000000000001421, 196.6227766016838245, -16.00000000000000000 ) ) ;
#9938=CARTESIAN_POINT ( 'NONE',  ( -48.00000000000000000, 191.6227766016837961, 1.224646799147353454E-15 ) ) ;
#9940=DIRECTION ( 'NONE',  ( 0.000000000000000000, 0.000000000000000000, 1.000000000000000000 ) ) ;
#9942=EDGE_LOOP ( 'NONE', ( #4916, #1105, #3674, #15794 ) ) ;
#9943=DIRECTION ( 'NONE',  ( 0.000000000000000000, 0.000000000000000000, 1.000000000000000000 ) ) ;
#9945=DIRECTION ( 'NONE',  ( -0.000000000000000000, -0.000000000000000000, 1.000000000000000000 ) ) ;
#9949=CARTESIAN_POINT ( 'NONE',  ( -7.970809231268917827, 17.99999999998357936, -12.80353734461080428 ) ) ;
#9951=CARTESIAN_POINT ( 'NONE',  ( 24.00000000000000000, 196.6227766016838245, -35.00000000000000000 ) ) ;
#9952=FACE_OUTER_BOUND ( 'NONE', #4903, .T. ) ;
#9953=ORIENTED_EDGE ( 'NONE', *, *, #13254, .T. ) ;
#9955=DIRECTION ( 'NONE',  ( -1.000000000000000000, -0.000000000000000000, -0.000000000000000000 ) ) ;
#9959=VERTEX_POINT ( 'NONE', #4258 ) ;
#9961=FACE_BOUND ( 'NONE', #13879, .T. ) ;
#9962=ADVANCED_FACE ( 'NONE', ( #13909 ), #8577, .F. ) ;
#9964=CARTESIAN_POINT ( 'NONE',  ( 49.99999999999998579, 191.6227766016837677, -5.571800142134975431 ) ) ;
#9965=CARTESIAN_POINT ( 'NONE',  ( 37.43654228017073393, 145.5167101299681178, -20.20458554073936241 ) ) ;
#9966=ORIENTED_EDGE ( 'NONE', *, *, #1988, .F. ) ;
#9970=ADVANCED_FACE ( 'NONE', ( #4338 ), #16474, .F. ) ;
#9971=CARTESIAN_POINT ( 'NONE',  ( -12.14981508666162036, 19.99999999999315037, -12.53017279448777366 ) ) ;
#9972=CARTESIAN_POINT ( 'NONE',  ( -48.00000000000000000, 154.3022685259950038, -9.999999999999900524 ) ) ;
#9975=ORIENTED_EDGE ( 'NONE', *, *, #9737, .T. ) ;
#9977=ORIENTED_EDGE ( 'NONE', *, *, #112, .T. ) ;
#9983=DIRECTION ( 'NONE',  ( -0.000000000000000000, -0.000000000000000000, -1.000000000000000000 ) ) ;
#9985=DIRECTION ( 'NONE',  ( -0.000000000000000000, -0.000000000000000000, 1.000000000000000000 ) ) ;
#9987=VERTEX_POINT ( 'NONE', #5750 ) ;
#9988=VERTEX_POINT ( 'NONE', #1688 ) ;
#9989=CARTESIAN_POINT ( 'NONE',  ( 24.80291332262510196, 19.99999999999999645, -7.298429162487363620 ) ) ;
#9990=CARTESIAN_POINT ( 'NONE',  ( -27.98221281347037959, 30.00000000000000000, 0.000000000000000000 ) ) ;
#9996=CARTESIAN_POINT ( 'NONE',  ( 35.59761955342209916, 201.6350306476045091, -13.74486639216963901 ) ) ;
#9999=VECTOR ( 'NONE', #16472, 1000.000000000000000 ) ;
#10000=CARTESIAN_POINT ( 'NONE',  ( -40.00000000000000000, 20.00000000000000000, -30.00000000000000355 ) ) ;
#10002=AXIS2_PLACEMENT_3D ( 'NONE', #9217, #16225, #7797 ) ;
#10003=DIRECTION ( 'NONE',  ( -1.000000000000000000, -0.000000000000000000, -0.000000000000000000 ) ) ;
#10004=CARTESIAN_POINT ( 'NONE',  ( -72.95161576004603887, 144.0140295085316779, -18.09598853029520171 ) ) ;
#10005=ORIENTED_EDGE ( 'NONE', *, *, #8412, .F. ) ;
#10008=CARTESIAN_POINT ( 'NONE',  ( -72.50000000000000000, 196.6227766016838245, -21.54065922853802562 ) ) ;
#10009=CARTESIAN_POINT ( 'NONE',  ( -25.15885279626527549, 18.00000000000000355, -15.13659797665870066 ) ) ;
#10011=DIRECTION ( 'NONE',  ( 0.000000000000000000, 0.000000000000000000, 1.000000000000000000 ) ) ;
#10012=EDGE_CURVE ( 'NONE', #14627, #4871, #3096, .T. ) ;
#10027=AXIS2_PLACEMENT_3D ( 'NONE', #4101, #14977, #10737 ) ;
#10028=ORIENTED_EDGE ( 'NONE', *, *, #994, .F. ) ;
#10031=CARTESIAN_POINT ( 'NONE',  ( -27.98221281347037959, 20.00000000000000355, -5.670874406215274277 ) ) ;
#10032=EDGE_LOOP ( 'NONE', ( #5518, #17104, #8729 ) ) ;
#10033=CARTESIAN_POINT ( 'NONE',  ( -96.00000000000001421, 171.6227766016838245, -30.00000000000000000 ) ) ;
#10040=ORIENTED_EDGE ( 'NONE', *, *, #12951, .T. ) ;
#10041=DIRECTION ( 'NONE',  ( -0.000000000000000000, -0.000000000000000000, -1.000000000000000000 ) ) ;
#10042=VECTOR ( 'NONE', #3425, 1000.000000000000000 ) ;
#10044=CARTESIAN_POINT ( 'NONE',  ( 24.10786375645522384, 141.9593924407984957, -14.48320912595415244 ) ) ;
#10045=AXIS2_PLACEMENT_3D ( 'NONE', #14404, #6082, #12988 ) ;
#10046=VECTOR ( 'NONE', #4552, 1000.000000000000000 ) ;
#10049=CARTESIAN_POINT ( 'NONE',  ( 48.00000000000000711, 159.6227766016838814, -8.071800142134975431 ) ) ;
#10053=DIRECTION ( 'NONE',  ( -0.000000000000000000, -0.000000000000000000, 1.000000000000000000 ) ) ;
#10054=CARTESIAN_POINT ( 'NONE',  ( -14.55266450408011636, 19.99999999999999645, -23.76398220081675206 ) ) ;
#10056=AXIS2_PLACEMENT_3D ( 'NONE', #207, #11002, #7449 ) ;
#10057=CIRCLE ( 'NONE', #14030, 2.500000000000002220 ) ;
#10058=AXIS2_PLACEMENT_3D ( 'NONE', #15727, #947, #7942 ) ;
#10059=EDGE_CURVE ( 'NONE', #14104, #15177, #6097, .T. ) ;
#10060=AXIS2_PLACEMENT_3D ( 'NONE', #4485, #397, #15012 ) ;
#10062=CARTESIAN_POINT ( 'NONE',  ( -80.00000000000001421, 196.6227766016838245, -16.00000000000000000 ) ) ;
#10064=DIRECTION ( 'NONE',  ( 0.000000000000000000, 0.000000000000000000, 1.000000000000000000 ) ) ;
#10065=EDGE_LOOP ( 'NONE', ( #3983, #5261, #3335, #784 ) ) ;
#10067=CARTESIAN_POINT ( 'NONE',  ( -95.00000000000000000, 201.6227766016838245, 0.000000000000000000 ) ) ;
#10069=VECTOR ( 'NONE', #1077, 1000.000000000000000 ) ;
#10070=AXIS2_PLACEMENT_3D ( 'NONE', #5509, #14890, #6761 ) ;
#10071=DIRECTION ( 'NONE',  ( 0.000000000000000000, 0.000000000000000000, 1.000000000000000000 ) ) ;
#10076=CARTESIAN_POINT ( 'NONE',  ( 20.49999999999998224, 10.00000000000000000, -35.00200000000000244 ) ) ;
#10079=CARTESIAN_POINT ( 'NONE',  ( 24.04231242562121551, 197.3572491277162158, -23.72357542124676044 ) ) ;
#10081=ORIENTED_EDGE ( 'NONE', *, *, #12533, .T. ) ;
#10083=CARTESIAN_POINT ( 'NONE',  ( 18.47379060770018810, 20.00000000000225953, -14.40819024183099728 ) ) ;
#10089=CARTESIAN_POINT ( 'NONE',  ( -87.50000000000004263, 146.6227766016838245, -35.00200000000000244 ) ) ;
#10091=VERTEX_POINT ( 'NONE', #795 ) ;
#10095=CARTESIAN_POINT ( 'NONE',  ( 196.0000000000000000, 155.6227766016839098, -12.50000337241049309 ) ) ;
#10101=DIRECTION ( 'NONE',  ( -1.000000000000000000, 0.000000000000000000, 0.000000000000000000 ) ) ;
#10104=EDGE_CURVE ( 'NONE', #16267, #11049, #7875, .T. ) ;
#10106=CARTESIAN_POINT ( 'NONE',  ( -45.00000000000000000, 120.0000000000000142, -15.00000000000000000 ) ) ;
#10107=CARTESIAN_POINT ( 'NONE',  ( -27.81025873171734375, 18.00000000000000355, -7.666431193274476641 ) ) ;
#10112=STYLED_ITEM ( 'NONE', ( #9696 ), #8036 ) ;
#10113=ORIENTED_EDGE ( 'NONE', *, *, #4947, .T. ) ;
#10116=DIRECTION ( 'NONE',  ( -1.000000000000000000, -0.000000000000000000, 0.000000000000000000 ) ) ;
#10117=CARTESIAN_POINT ( 'NONE',  ( -17.63576980228536328, 32.18555361985414720, -8.400096275226864861 ) ) ;
#10122=CARTESIAN_POINT ( 'NONE',  ( 15.00000000000000000, 171.6227766016838245, 0.000000000000000000 ) ) ;
#10131=FACE_BOUND ( 'NONE', #860, .T. ) ;
#10132=ADVANCED_FACE ( 'NONE', ( #1942 ), #619, .F. ) ;
#10133=ORIENTED_EDGE ( 'NONE', *, *, #15927, .F. ) ;
#10134=ORIENTED_EDGE ( 'NONE', *, *, #9371, .F. ) ;
#10135=ORIENTED_EDGE ( 'NONE', *, *, #1278, .F. ) ;
#10138=VERTEX_POINT ( 'NONE', #15741 ) ;
#10141=CARTESIAN_POINT ( 'NONE',  ( -40.00000000000000000, 4.000000000000000000, -33.00000000000000711 ) ) ;
#10148=ADVANCED_FACE ( 'NONE', ( #14082 ), #2288, .F. ) ;
#10150=CARTESIAN_POINT ( 'NONE',  ( -22.80699178664306004, 19.99999999999999645, -18.33022619056923119 ) ) ;
#10151=EDGE_CURVE ( 'NONE', #1517, #6848, #16091, .T. ) ;
#10153=CIRCLE ( 'NONE', #4792, 9.999999999999998224 ) ;
#10155=CIRCLE ( 'NONE', #3954, 2.500000000000002220 ) ;
#10156=CARTESIAN_POINT ( 'NONE',  ( 0.000000000000000000, 20.00000000000000000, 0.000000000000000000 ) ) ;
#10158=CARTESIAN_POINT ( 'NONE',  ( -85.27494917608791525, 141.2912748254776147, -13.00000000000000000 ) ) ;
#10161=CARTESIAN_POINT ( 'NONE',  ( -85.86147415632849800, 195.3295718346067531, -25.74952675241122080 ) ) ;
#10162=VECTOR ( 'NONE', #11671, 1000.000000000000000 ) ;
#10163=CARTESIAN_POINT ( 'NONE',  ( 49.99999999999998579, 175.6227766016838245, -3.071800142134975431 ) ) ;
#10164=AXIS2_PLACEMENT_3D ( 'NONE', #3510, #12897, #15716 ) ;
#10167=CARTESIAN_POINT ( 'NONE',  ( -151.9615242270660929, 171.6227766016838245, 0.000000000000000000 ) ) ;
#10168=ORIENTED_EDGE ( 'NONE', *, *, #4203, .T. ) ;
#10169=DIRECTION ( 'NONE',  ( 0.000000000000000000, 0.000000000000000000, 1.000000000000000000 ) ) ;
#10171=CARTESIAN_POINT ( 'NONE',  ( -75.00000000000000000, 196.6227766016838245, -12.99999999999999822 ) ) ;
#10172=CARTESIAN_POINT ( 'NONE',  ( 30.28723734794761313, 202.6220268295897426, -16.24950730846250835 ) ) ;
#10173=VERTEX_POINT ( 'NONE', #6719 ) ;
#10175=CARTESIAN_POINT ( 'NONE',  ( 23.18512258076559007, 19.99999999999999645, -23.22991426836919260 ) ) ;
#10181=AXIS2_PLACEMENT_3D ( 'NONE', #14933, #13525, #13885 ) ;
#10189=AXIS2_PLACEMENT_3D ( 'NONE', #1475, #3962, #14754 ) ;
#10193=DIRECTION ( 'NONE',  ( -1.156482317317868274E-16, 1.000000000000000000, 0.000000000000000000 ) ) ;
#10194=ORIENTED_EDGE ( 'NONE', *, *, #4895, .F. ) ;
#10195=CARTESIAN_POINT ( 'NONE',  ( 22.50000000000001421, 146.6227766016838245, -13.00000000000000000 ) ) ;
#10197=VERTEX_POINT ( 'NONE', #11839 ) ;
#10202=ORIENTED_EDGE ( 'NONE', *, *, #10666, .F. ) ;
#10206=ORIENTED_EDGE ( 'NONE', *, *, #1656, .T. ) ;
#10209=CARTESIAN_POINT ( 'NONE',  ( -14.60673078645093703, 31.57037919282903360, -12.49506642855920724 ) ) ;
#10213=CYLINDRICAL_SURFACE ( 'NONE', #10688, 750.0000000000001137 ) ;
#10214=VECTOR ( 'NONE', #8072, 1000.000000000000000 ) ;
#10215=CARTESIAN_POINT ( 'NONE',  ( -7.379000772444994638, 20.00000000000000000, -25.00000000000000000 ) ) ;
#10217=CARTESIAN_POINT ( 'NONE',  ( 28.87291500020774393, 190.7253031951458411, -29.32741221247050234 ) ) ;
#10222=ORIENTED_EDGE ( 'NONE', *, *, #3444, .T. ) ;
#10223=CARTESIAN_POINT ( 'NONE',  ( -83.78675088369342916, 153.1023373578139797, -27.31345131271289972 ) ) ;
#10227=DIRECTION ( 'NONE',  ( 0.000000000000000000, 0.000000000000000000, -1.000000000000000000 ) ) ;
#10228=CARTESIAN_POINT ( 'NONE',  ( -40.00000000000000000, 20.00000000000000000, -30.00000000000000355 ) ) ;
#10234=CARTESIAN_POINT ( 'NONE',  ( 49.99999999999998579, 167.6227766016838530, -5.571800142134975431 ) ) ;
#10236=CARTESIAN_POINT ( 'NONE',  ( -10.59078875499043981, 19.99999999999999645, -13.69642986623834702 ) ) ;
#10243=ADVANCED_FACE ( 'NONE', ( #5201, #6542 ), #3710, .T. ) ;
#10244=CARTESIAN_POINT ( 'NONE',  ( 49.99999999999998579, 167.6227766016838530, -8.071800142134975431 ) ) ;
#10247=LINE ( 'NONE', #5930, #10411 ) ;
#10248=CARTESIAN_POINT ( 'NONE',  ( 8.630636718464335999, 133.1548047818457690, -12.68018750699619268 ) ) ;
#10249=ORIENTED_EDGE ( 'NONE', *, *, #16389, .T. ) ;
#10255=ORIENTED_EDGE ( 'NONE', *, *, #8085, .T. ) ;
#10256=CARTESIAN_POINT ( 'NONE',  ( 17.04141343047935564, 29.97166846511136029, -14.77658840773744409 ) ) ;
#10257=DIRECTION ( 'NONE',  ( -1.000000000000000000, -0.000000000000000000, 0.000000000000000000 ) ) ;
#10261=DIRECTION ( 'NONE',  ( 1.000000000000000000, 0.000000000000000000, 0.000000000000000000 ) ) ;
#10263=DIRECTION ( 'NONE',  ( 0.000000000000000000, 0.000000000000000000, 1.000000000000000000 ) ) ;
#10264=PLANE ( 'NONE',  #14321 ) ;
#10267=DIRECTION ( 'NONE',  ( -1.000000000000000000, 0.000000000000000000, 0.000000000000000000 ) ) ;
#10268=CARTESIAN_POINT ( 'NONE',  ( 35.86376614940371610, 145.1725333695280256, -22.94453145061437382 ) ) ;
#10271=ORIENTED_EDGE ( 'NONE', *, *, #12254, .T. ) ;
#10273=CARTESIAN_POINT ( 'NONE',  ( -80.00000000000002842, 146.6227766016838245, -35.00200000000000244 ) ) ;
#10281=FACE_OUTER_BOUND ( 'NONE', #1629, .T. ) ;
#10282=EDGE_CURVE ( 'NONE', #11263, #6590, #6778, .T. ) ;
#10285=CARTESIAN_POINT ( 'NONE',  ( -21.36854569161881301, 18.00000000000000000, -19.70709815271291632 ) ) ;
#10288=CARTESIAN_POINT ( 'NONE',  ( -14.54670497998687217, 20.00000000000000000, -23.76610458325320607 ) ) ;
#10290=CARTESIAN_POINT ( 'NONE',  ( 25.68328880728000030, 192.4368082929522075, -28.14105258436205403 ) ) ;
#10291=DIRECTION ( 'NONE',  ( 0.000000000000000000, 0.000000000000000000, 1.000000000000000000 ) ) ;
#10292=EDGE_LOOP ( 'NONE', ( #4597, #1751, #3937, #16066 ) ) ;
#10296=CARTESIAN_POINT ( 'NONE',  ( -72.65282855708331056, 148.1823054118431742, -23.23525722188764675 ) ) ;
#10298=ORIENTED_EDGE ( 'NONE', *, *, #10666, .T. ) ;
#10303=CARTESIAN_POINT ( 'NONE',  ( 30.44099542279310810, 152.6108673192418905, -29.38619085311482237 ) ) ;
#10304=CARTESIAN_POINT ( 'NONE',  ( 196.0000000000000000, 151.6227766016839098, -8.071800142134973655 ) ) ;
#10306=AXIS2_PLACEMENT_3D ( 'NONE', #7019, #4359, #11680 ) ;
#10312=ORIENTED_EDGE ( 'NONE', *, *, #884, .T. ) ;
#10316=ORIENTED_EDGE ( 'NONE', *, *, #8936, .T. ) ;
#10327=VECTOR ( 'NONE', #6940, 1000.000000000000000 ) ;
#10328=ORIENTED_EDGE ( 'NONE', *, *, #16040, .T. ) ;
#10332=CARTESIAN_POINT ( 'NONE',  ( -48.00000000000000000, 154.3022685259950038, -9.999999999999900524 ) ) ;
#10334=VERTEX_POINT ( 'NONE', #72 ) ;
#10335=EDGE_CURVE ( 'NONE', #8522, #7175, #3387, .T. ) ;
#10336=EDGE_CURVE ( 'NONE', #7753, #7553, #4237, .T. ) ;
#10339=CARTESIAN_POINT ( 'NONE',  ( 17.53546816055562374, 19.99999999999999645, -24.87355917367628422 ) ) ;
#10341=CARTESIAN_POINT ( 'NONE',  ( 11.28101412774664958, 138.8108036852440250, -13.45198100927934348 ) ) ;
#10344=CARTESIAN_POINT ( 'NONE',  ( 12.56741672263938625, 143.7071609262609400, -17.59902447249972113 ) ) ;
#10345=AXIS2_PLACEMENT_3D ( 'NONE', #12235, #16150, #13575 ) ;
#10348=FACE_OUTER_BOUND ( 'NONE', #12271, .T. ) ;
#10350=DIRECTION ( 'NONE',  ( -1.000000000000000000, -0.000000000000000000, 0.000000000000000000 ) ) ;
#10355=CARTESIAN_POINT ( 'NONE',  ( 34.32861903462791986, 142.4529008285661575, -19.34799176589369907 ) ) ;
#10356=AXIS2_PLACEMENT_3D ( 'NONE', #4003, #10715, #8139 ) ;
#10357=VERTEX_POINT ( 'NONE', #12278 ) ;
#10360=ORIENTED_EDGE ( 'NONE', *, *, #3440, .T. ) ;
#10361=CARTESIAN_POINT ( 'NONE',  ( -25.49999999999998579, 10.00000000000000000, 1.387778780781445676E-14 ) ) ;
#10364=ORIENTED_EDGE ( 'NONE', *, *, #6527, .F. ) ;
#10369=AXIS2_PLACEMENT_3D ( 'NONE', #5578, #5671, #14958 ) ;
#10371=CARTESIAN_POINT ( 'NONE',  ( 26.18268817859244280, 190.1433283039765172, -27.31438289289431864 ) ) ;
#10373=CARTESIAN_POINT ( 'NONE',  ( -26.90043998675938397, 18.00000000000000000, -11.53672424425030840 ) ) ;
#10375=ORIENTED_EDGE ( 'NONE', *, *, #4471, .F. ) ;
#10378=CARTESIAN_POINT ( 'NONE',  ( 32.99829944797550496, 191.4074798671405233, -28.87243506922801473 ) ) ;
#10379=CARTESIAN_POINT ( 'NONE',  ( -100.0000000000000000, 201.9542783778900059, -13.00000000000000000 ) ) ;
#10380=ORIENTED_EDGE ( 'NONE', *, *, #8034, .T. ) ;
#10383=ORIENTED_EDGE ( 'NONE', *, *, #3532, .T. ) ;
#10385=CIRCLE ( 'NONE', #4747, 5.000000000000004441 ) ;
#10389=PLANE ( 'NONE',  #15280 ) ;
#10391=CARTESIAN_POINT ( 'NONE',  ( 27.57840531033536990, 152.1166601635960944, -29.06070213693891091 ) ) ;
#10396=ORIENTED_EDGE ( 'NONE', *, *, #8349, .F. ) ;
#10400=CARTESIAN_POINT ( 'NONE',  ( 225.0000000000000000, 89.99999999999997158, 0.000000000000000000 ) ) ;
#10401=CARTESIAN_POINT ( 'NONE',  ( -27.98221281347032274, 19.99999999999999645, -4.999999999999996447 ) ) ;
#10402=VERTEX_POINT ( 'NONE', #11042 ) ;
#10403=CARTESIAN_POINT ( 'NONE',  ( -86.42104199761078576, 142.7196187763571515, -15.94638436093396727 ) ) ;
#10405=EDGE_CURVE ( 'NONE', #17378, #13903, #4513, .T. ) ;
#10406=EDGE_CURVE ( 'NONE', #9101, #12781, #9592, .T. ) ;
#10411=VECTOR ( 'NONE', #615, 1000.000000000000000 ) ;
#10413=ORIENTED_EDGE ( 'NONE', *, *, #625, .T. ) ;
#10416=CARTESIAN_POINT ( 'NONE',  ( -80.26436704404596867, 140.6225526278765017, -16.24764948572450507 ) ) ;
#10417=CARTESIAN_POINT ( 'NONE',  ( 48.00000000000000711, 191.6227766016837677, -5.571800142134975431 ) ) ;
#10420=AXIS2_PLACEMENT_3D ( 'NONE', #10891, #5683, #5504 ) ;
#10421=VECTOR ( 'NONE', #1241, 1000.000000000000000 ) ;
#10423=AXIS2_PLACEMENT_3D ( 'NONE', #12265, #12446, #16352 ) ;
#10426=CARTESIAN_POINT ( 'NONE',  ( 28.59595936524185689, 202.4574374834314483, -16.55982638047048283 ) ) ;
#10431=CARTESIAN_POINT ( 'NONE',  ( 12.52734837489390785, 131.0783166553242722, -13.12014565386486176 ) ) ;
#10433=CARTESIAN_POINT ( 'NONE',  ( -84.82208992409042025, 150.1982800653300387, -27.67726561134452723 ) ) ;
#10434=CARTESIAN_POINT ( 'NONE',  ( 15.42236477930291549, 143.2198172345435410, -16.80652640733168823 ) ) ;
#10436=VERTEX_POINT ( 'NONE', #13802 ) ;
#10437=CYLINDRICAL_SURFACE ( 'NONE', #14354, 2.500000000000000444 ) ;
#10442=ADVANCED_FACE ( 'NONE', ( #15104 ), #9890, .F. ) ;
#10443=EDGE_CURVE ( 'NONE', #14506, #16820, #13970, .T. ) ;
#10444=EDGE_CURVE ( 'NONE', #9042, #16339, #12422, .T. ) ;
#10450=LINE ( 'NONE', #6121, #10590 ) ;
#10453=AXIS2_PLACEMENT_3D ( 'NONE', #1557, #2715, #12268 ) ;
#10454=AXIS2_PLACEMENT_3D ( 'NONE', #3186, #9985, #3270 ) ;
#10464=VERTEX_POINT ( 'NONE', #16371 ) ;
#10470=CARTESIAN_POINT ( 'NONE',  ( 24.06456496986166016, 192.0313071030112155, -25.93356563065114173 ) ) ;
#10472=CARTESIAN_POINT ( 'NONE',  ( -23.66837786582113878, 18.00000000000000000, -17.32703391568840345 ) ) ;
#10474=DIRECTION ( 'NONE',  ( -1.156482317317868274E-16, 1.000000000000000000, -0.000000000000000000 ) ) ;
#10475=ORIENTED_EDGE ( 'NONE', *, *, #11462, .T. ) ;
#10477=DIRECTION ( 'NONE',  ( -0.000000000000000000, -1.000000000000000000, 0.000000000000000000 ) ) ;
#10479=ORIENTED_EDGE ( 'NONE', *, *, #5983, .F. ) ;
#10481=ORIENTED_EDGE ( 'NONE', *, *, #7115, .T. ) ;
#10483=LINE ( 'NONE', #15887, #2770 ) ;
#10487=CARTESIAN_POINT ( 'NONE',  ( 36.00000000000003553, 147.2627523208502964, -25.14806991105193035 ) ) ;
#10488=VECTOR ( 'NONE', #6582, 1000.000000000000000 ) ;
#10493=CARTESIAN_POINT ( 'NONE',  ( 6.134011831684049731, 144.1839557653416080, -18.33333333333335702 ) ) ;
#10498=CARTESIAN_POINT ( 'NONE',  ( 34.93420767853316988, 30.00000000000000000, 0.000000000000000000 ) ) ;
#10500=ORIENTED_EDGE ( 'NONE', *, *, #1385, .T. ) ;
#10502=DIRECTION ( 'NONE',  ( 1.000000000000000000, 0.000000000000000000, -0.000000000000000000 ) ) ;
#10503=CARTESIAN_POINT ( 'NONE',  ( 49.99999999999998579, 163.6227766016838530, -12.50000337241049309 ) ) ;
#10504=ORIENTED_EDGE ( 'NONE', *, *, #12794, .T. ) ;
#10506=CARTESIAN_POINT ( 'NONE',  ( -27.98221281347037959, 18.00000000000000355, 0.000000000000000000 ) ) ;
#10508=CARTESIAN_POINT ( 'NONE',  ( -74.50324869458546573, 144.1922489206527018, -21.74472059540656232 ) ) ;
#10509=EDGE_CURVE ( 'NONE', #7894, #11405, #11569, .T. ) ;
#10510=CARTESIAN_POINT ( 'NONE',  ( 7.743794661876905572, 133.6328069455646528, -12.86244959688548128 ) ) ;
#10513=CARTESIAN_POINT ( 'NONE',  ( 48.00000000000000711, 155.6227766016839098, -10.00000337241049309 ) ) ;
#10516=CARTESIAN_POINT ( 'NONE',  ( 37.99999999999998579, 2.000000000000000000, -28.00000000000001066 ) ) ;
#10517=ORIENTED_EDGE ( 'NONE', *, *, #2349, .F. ) ;
#10518=ORIENTED_EDGE ( 'NONE', *, *, #4082, .T. ) ;
#10519=CARTESIAN_POINT ( 'NONE',  ( 7.098239199200468086, 139.5131674267937854, -14.94273745765201866 ) ) ;
#10523=CARTESIAN_POINT ( 'NONE',  ( 20.41303537789175948, 141.9260521957599508, -14.39564681615556907 ) ) ;
#10525=FACE_OUTER_BOUND ( 'NONE', #11012, .T. ) ;
#10526=DIRECTION ( 'NONE',  ( -1.000000000000000000, 0.000000000000000000, 0.000000000000000000 ) ) ;
#10527=CARTESIAN_POINT ( 'NONE',  ( 22.95161576004601045, 199.2315236948359143, -18.09598853029519816 ) ) ;
#10529=DIRECTION ( 'NONE',  ( 0.000000000000000000, 1.000000000000000000, 0.000000000000000000 ) ) ;
#10530=CARTESIAN_POINT ( 'NONE',  ( 49.99999999999998579, 191.6227766016837677, -5.571800142134975431 ) ) ;
#10531=CARTESIAN_POINT ( 'NONE',  ( -24.99999999999999289, 90.00000000000000000, -4.999999999999999112 ) ) ;
#10538=DIRECTION ( 'NONE',  ( 1.000000000000000000, 0.000000000000000000, 0.000000000000000000 ) ) ;
#10539=CARTESIAN_POINT ( 'NONE',  ( -7.379000772445021283, 18.00000000000000000, -25.00000000000000355 ) ) ;
#10540=EDGE_CURVE ( 'NONE', #1367, #14130, #1123, .T. ) ;
#10541=VERTEX_POINT ( 'NONE', #683 ) ;
#10544=ORIENTED_EDGE ( 'NONE', *, *, #2959, .F. ) ;
#10548=CARTESIAN_POINT ( 'NONE',  ( 23.91918570238912167, 192.2260612991243818, -25.77925661938085611 ) ) ;
#10549=CARTESIAN_POINT ( 'NONE',  ( -96.00000000000001421, 141.6227766016838245, 5.510910596163088767E-15 ) ) ;
#10550=CARTESIAN_POINT ( 'NONE',  ( -10.72783954291835151, 17.99999999999999289, -10.92811494094397951 ) ) ;
#10551=VERTEX_POINT ( 'NONE', #2089 ) ;
#10553=ORIENTED_EDGE ( 'NONE', *, *, #14232, .T. ) ;
#10556=EDGE_CURVE ( 'NONE', #4348, #4546, #15557, .T. ) ;
#10557=ORIENTED_EDGE ( 'NONE', *, *, #1101, .F. ) ;
#10560=ADVANCED_FACE ( 'NONE', ( #11564, #3346 ), #12732, .F. ) ;
#10563=CARTESIAN_POINT ( 'NONE',  ( -75.11153254487454944, 152.3168652870156450, -26.76420670456568729 ) ) ;
#10565=ORIENTED_EDGE ( 'NONE', *, *, #5189, .T. ) ;
#10573=VECTOR ( 'NONE', #7391, 1000.000000000000000 ) ;
#10574=ORIENTED_EDGE ( 'NONE', *, *, #12827, .F. ) ;
#10577=CARTESIAN_POINT ( 'NONE',  ( 48.00000000000000711, 167.6227766016838530, -8.071800142134975431 ) ) ;
#10578=CARTESIAN_POINT ( 'NONE',  ( -90.80384757729339640, 204.6227766016838245, 0.000000000000000000 ) ) ;
#10582=LINE ( 'NONE', #12993, #16975 ) ;
#10584=FACE_OUTER_BOUND ( 'NONE', #7349, .T. ) ;
#10587=ORIENTED_EDGE ( 'NONE', *, *, #13621, .F. ) ;
#10590=VECTOR ( 'NONE', #10101, 1000.000000000000000 ) ;
#10592=CARTESIAN_POINT ( 'NONE',  ( -79.32805325232327220, 140.6591056634353265, -16.31724425057295136 ) ) ;
#10599=EDGE_CURVE ( 'NONE', #2736, #12122, #15540, .T. ) ;
#10600=DIRECTION ( 'NONE',  ( 1.000000000000000000, 0.000000000000000000, 0.000000000000000000 ) ) ;
#10601=AXIS2_PLACEMENT_3D ( 'NONE', #15825, #2283, #15912 ) ;
#10604=CIRCLE ( 'NONE', #7497, 2.500000000000002220 ) ;
#10605=ORIENTED_EDGE ( 'NONE', *, *, #16105, .T. ) ;
#10608=CARTESIAN_POINT ( 'NONE',  ( -85.97509853867674678, 147.2612100285404040, -25.13395616064556037 ) ) ;
#10609=EDGE_CURVE ( 'NONE', #1185, #3017, #5071, .T. ) ;
#10610=CARTESIAN_POINT ( 'NONE',  ( 12.74723713713078155, 129.4272226793184473, -10.49625762048852451 ) ) ;
#10615=FACE_OUTER_BOUND ( 'NONE', #14000, .T. ) ;
#10617=CARTESIAN_POINT ( 'NONE',  ( 196.0000000000000000, 191.6227766016837677, -8.071800142134975431 ) ) ;
#10619=CARTESIAN_POINT ( 'NONE',  ( 20.85766706164172035, 17.99999999999999645, -10.55326734450395954 ) ) ;
#10621=CARTESIAN_POINT ( 'NONE',  ( -3.000000000000000888, 206.6227766016838245, 2.143131898507868248E-15 ) ) ;
#10622=PLANE ( 'NONE',  #543 ) ;
#10623=CARTESIAN_POINT ( 'NONE',  ( 34.93420767853316988, 30.00000000000000000, -15.00000000000000000 ) ) ;
#10627=CARTESIAN_POINT ( 'NONE',  ( -25.00000000000002132, 120.0000000000000284, -5.000000000000023093 ) ) ;
#10628=CARTESIAN_POINT ( 'NONE',  ( -19.25702671965661850, 19.99999999999999645, -21.36300512502526416 ) ) ;
#10631=AXIS2_PLACEMENT_3D ( 'NONE', #5449, #13597, #3043 ) ;
#10632=EDGE_CURVE ( 'NONE', #7474, #9334, #10153, .T. ) ;
#10642=VERTEX_POINT ( 'NONE', #10493 ) ;
#10644=AXIS2_PLACEMENT_3D ( 'NONE', #11241, #16912, #8926 ) ;
#10646=CARTESIAN_POINT ( 'NONE',  ( 26.92553734538028110, 189.7763206329742047, -27.55849099911373301 ) ) ;
#10649=AXIS2_PLACEMENT_3D ( 'NONE', #6558, #4002, #5 ) ;
#10650=CARTESIAN_POINT ( 'NONE',  ( -15.50256837817153333, 32.53516993624282350, -8.343687756225392604 ) ) ;
#10655=CARTESIAN_POINT ( 'NONE',  ( -80.59986690501729356, 189.1412428432857951, -27.96613953460097690 ) ) ;
#10663=CARTESIAN_POINT ( 'NONE',  ( 15.58935622847965163, 125.0306600298041815, -3.338394242842863679 ) ) ;
#10665=CARTESIAN_POINT ( 'NONE',  ( 25.29742550462585982, 150.3543615375533022, -27.79730406782767105 ) ) ;
#10666=EDGE_CURVE ( 'NONE', #10091, #15177, #5444, .T. ) ;
#10667=LINE ( 'NONE', #8006, #11047 ) ;
#10668=ADVANCED_FACE ( 'NONE', ( #15810 ), #6328, .F. ) ;
#10672=CARTESIAN_POINT ( 'NONE',  ( -83.47514333733060710, 201.5283731665715834, -18.18938113080313101 ) ) ;
#10673=CARTESIAN_POINT ( 'NONE',  ( 23.61565302391275267, 29.88537503463918554, -10.00682404417760551 ) ) ;
#10677=CARTESIAN_POINT ( 'NONE',  ( 37.99999999999998579, 20.00000000000000000, -30.00000000000001066 ) ) ;
#10678=DIRECTION ( 'NONE',  ( -2.312964634635742464E-16, 0.000000000000000000, -1.000000000000000000 ) ) ;
#10681=VECTOR ( 'NONE', #214, 1000.000000000000000 ) ;
#10688=AXIS2_PLACEMENT_3D ( 'NONE', #6400, #16953, #3749 ) ;
#10690=CARTESIAN_POINT ( 'NONE',  ( 15.45427063382542165, 18.00000000000226663, -13.01057400152831711 ) ) ;
#10691=CARTESIAN_POINT ( 'NONE',  ( -82.40346994510062473, 141.1206502181308622, -17.16533225383573935 ) ) ;
#10697=CARTESIAN_POINT ( 'NONE',  ( -27.99999999999998224, 10.00000000000000000, -16.00000000000000000 ) ) ;
#10698=FACE_BOUND ( 'NONE', #15566, .T. ) ;
#10700=EDGE_LOOP ( 'NONE', ( #14475, #4181, #14216, #2931 ) ) ;
#10701=CARTESIAN_POINT ( 'NONE',  ( 9.819856892917396607, 139.1316717379867214, -14.17181165802795206 ) ) ;
#10703=LINE ( 'NONE', #15752, #11494 ) ;
#10704=CARTESIAN_POINT ( 'NONE',  ( 14.24850047812951104, 138.6393229685333779, -3.919138222309428876 ) ) ;
#10708=EDGE_CURVE ( 'NONE', #15255, #2414, #7834, .T. ) ;
#10715=DIRECTION ( 'NONE',  ( -1.000000000000000000, -0.000000000000000000, -0.000000000000000000 ) ) ;
#10716=CARTESIAN_POINT ( 'NONE',  ( 21.44211297938456084, 29.87092986353274426, -9.660732976998257726 ) ) ;
#10719=CARTESIAN_POINT ( 'NONE',  ( 35.00000000000000000, 196.6227766016838245, 0.000000000000000000 ) ) ;
#10724=CARTESIAN_POINT ( 'NONE',  ( 39.99999999999998579, 0.000000000000000000, -33.00000000000000711 ) ) ;
#10728=EDGE_LOOP ( 'NONE', ( #7401, #16004, #1483, #5167, #5136, #14811, #16240 ) ) ;
#10737=DIRECTION ( 'NONE',  ( 0.000000000000000000, 0.000000000000000000, 1.000000000000000000 ) ) ;
#10739=LINE ( 'NONE', #11884, #10214 ) ;
#10740=CARTESIAN_POINT ( 'NONE',  ( -80.00000000000001421, 196.6227766016838245, -16.00000000000000000 ) ) ;
#10742=VECTOR ( 'NONE', #16987, 1000.000000000000000 ) ;
#10748=DIRECTION ( 'NONE',  ( 1.000000000000000000, 0.000000000000000000, 0.000000000000000000 ) ) ;
#10751=EDGE_LOOP ( 'NONE', ( #7860, #4831, #1678, #11556 ) ) ;
#10753=VECTOR ( 'NONE', #2539, 1000.000000000000000 ) ;
#10756=ORIENTED_EDGE ( 'NONE', *, *, #16605, .F. ) ;
#10758=CARTESIAN_POINT ( 'NONE',  ( 6.134011831684053284, 142.5209969267753820, -19.44444444444444642 ) ) ;
#10769=AXIS2_PLACEMENT_3D ( 'NONE', #5878, #15167, #8444 ) ;
#10770=FACE_OUTER_BOUND ( 'NONE', #15383, .T. ) ;
#10773=CARTESIAN_POINT ( 'NONE',  ( -80.00000000000001421, 196.6227766016838245, 0.000000000000000000 ) ) ;
#10774=EDGE_CURVE ( 'NONE', #5721, #5744, #15414, .T. ) ;
#10775=ORIENTED_EDGE ( 'NONE', *, *, #16534, .F. ) ;
#10776=AXIS2_PLACEMENT_3D ( 'NONE', #4980, #1088, #14459 ) ;
#10777=EDGE_LOOP ( 'NONE', ( #16589, #10475, #2517, #14403 ) ) ;
#10779=DIRECTION ( 'NONE',  ( 0.000000000000000000, 0.000000000000000000, 1.000000000000000000 ) ) ;
#10780=CARTESIAN_POINT ( 'NONE',  ( -23.00000000000002132, 122.0000000000000142, -9.686291501015228178 ) ) ;
#10781=CARTESIAN_POINT ( 'NONE',  ( -84.78365660347692767, 142.9837419059134334, -20.12545249291982330 ) ) ;
#10782=FACE_OUTER_BOUND ( 'NONE', #15906, .T. ) ;
#10787=AXIS2_PLACEMENT_3D ( 'NONE', #17293, #9403, #31 ) ;
#10789=CARTESIAN_POINT ( 'NONE',  ( 48.00000000000000711, 175.6227766016838245, -8.071800142134975431 ) ) ;
#10791=EDGE_CURVE ( 'NONE', #1100, #7583, #7482, .T. ) ;
#10795=DIRECTION ( 'NONE',  ( -1.000000000000000000, -0.000000000000000000, 0.000000000000000000 ) ) ;
#10797=CARTESIAN_POINT ( 'NONE',  ( -22.99999999999998224, 10.00000000000000000, 0.000000000000000000 ) ) ;
#10801=DIRECTION ( 'NONE',  ( -1.000000000000000000, 0.000000000000000000, 0.000000000000000000 ) ) ;
#10802=CARTESIAN_POINT ( 'NONE',  ( 18.97220464449422295, 17.99999999999999645, -12.00279687791388383 ) ) ;
#10804=CARTESIAN_POINT ( 'NONE',  ( -80.00000000000001421, 196.6227766016838245, -35.00000000000000000 ) ) ;
#10806=DIRECTION ( 'NONE',  ( -1.000000000000000000, 0.000000000000000000, 0.000000000000000000 ) ) ;
#10807=VERTEX_POINT ( 'NONE', #9749 ) ;
#10809=ORIENTED_EDGE ( 'NONE', *, *, #987, .T. ) ;
#10813=ORIENTED_EDGE ( 'NONE', *, *, #10151, .F. ) ;
#10820=LINE ( 'NONE', #194, #8902 ) ;
#10825=EDGE_CURVE ( 'NONE', #4808, #16973, #14549, .T. ) ;
#10826=ORIENTED_EDGE ( 'NONE', *, *, #843, .F. ) ;
#10828=CARTESIAN_POINT ( 'NONE',  ( -75.75320729262173813, 190.4349707265699294, -27.11332964807919765 ) ) ;
#10831=ORIENTED_EDGE ( 'NONE', *, *, #5157, .F. ) ;
#10833=CARTESIAN_POINT ( 'NONE',  ( -7.379000772445021283, 30.00000000000000000, -13.00000000000000000 ) ) ;
#10840=CARTESIAN_POINT ( 'NONE',  ( -80.00000000000002842, 146.6227766016838245, 0.000000000000000000 ) ) ;
#10842=ORIENTED_EDGE ( 'NONE', *, *, #14418, .T. ) ;
#10843=CARTESIAN_POINT ( 'NONE',  ( -78.93349828499714249, 202.5285685493726362, -16.42664996635052432 ) ) ;
#10844=LINE ( 'NONE', #2710, #10753 ) ;
#10845=CARTESIAN_POINT ( 'NONE',  ( 33.66231827095856488, 20.00000000000000000, -12.04861179558545636 ) ) ;
#10848=FACE_OUTER_BOUND ( 'NONE', #196, .T. ) ;
#10849=ORIENTED_EDGE ( 'NONE', *, *, #11223, .T. ) ;
#10852=ORIENTED_EDGE ( 'NONE', *, *, #6293, .T. ) ;
#10853=CARTESIAN_POINT ( 'NONE',  ( 24.00000000000000000, 196.6227766016838245, -24.49489742783178770 ) ) ;
#10854=DIRECTION ( 'NONE',  ( 1.000000000000000000, 0.000000000000000000, 0.000000000000000000 ) ) ;
#10856=CIRCLE ( 'NONE', #4691, 33.00000000000000000 ) ;
#10861=EDGE_CURVE ( 'NONE', #12804, #8947, #9930, .T. ) ;
#10862=CYLINDRICAL_SURFACE ( 'NONE', #2267, 5.000000000000004441 ) ;
#10863=AXIS2_PLACEMENT_3D ( 'NONE', #3869, #2540, #13339 ) ;
#10864=CARTESIAN_POINT ( 'NONE',  ( 15.51497662817079082, 137.3737080369936905, -9.118346648348486738 ) ) ;
#10867=DIRECTION ( 'NONE',  ( 1.000000000000000000, 0.000000000000000000, 0.000000000000000000 ) ) ;
#10869=VERTEX_POINT ( 'NONE', #5692 ) ;
#10870=CARTESIAN_POINT ( 'NONE',  ( -80.21954352204551242, 190.6224931067073953, -29.39406016266899968 ) ) ;
#10872=DIRECTION ( 'NONE',  ( -1.000000000000000000, -0.000000000000000000, -0.000000000000000000 ) ) ;
#10873=CARTESIAN_POINT ( 'NONE',  ( 34.42405209918207731, 18.00000000000000000, -9.535225002503356251 ) ) ;
#10875=CARTESIAN_POINT ( 'NONE',  ( 23.18512258076444610, 18.00000000000000000, -23.22991426836919615 ) ) ;
#10877=DIRECTION ( 'NONE',  ( 1.000000000000000000, 0.000000000000000000, 0.000000000000000000 ) ) ;
#10878=EDGE_CURVE ( 'NONE', #8582, #15415, #11154, .T. ) ;
#10882=ADVANCED_FACE ( 'NONE', ( #11160 ), #8427, .T. ) ;
#10884=ORIENTED_EDGE ( 'NONE', *, *, #3059, .T. ) ;
#10885=CARTESIAN_POINT ( 'NONE',  ( -70.00000000000000000, 171.6227766016838245, 0.000000000000000000 ) ) ;
#10888=DIRECTION ( 'NONE',  ( -0.000000000000000000, -0.000000000000000000, 1.000000000000000000 ) ) ;
#10891=CARTESIAN_POINT ( 'NONE',  ( 48.00000000000000711, 151.6227766016839098, -5.571800142134973655 ) ) ;
#10892=ORIENTED_EDGE ( 'NONE', *, *, #8829, .T. ) ;
#10894=CARTESIAN_POINT ( 'NONE',  ( 31.45415618582128658, 153.9859494455611468, -27.89172594985638653 ) ) ;
#10895=AXIS2_PLACEMENT_3D ( 'NONE', #627, #1693, #7351 ) ;
#10897=LINE ( 'NONE', #6845, #9224 ) ;
#10899=DIRECTION ( 'NONE',  ( -1.000000000000000000, 0.000000000000000000, 0.000000000000000000 ) ) ;
#10902=CIRCLE ( 'NONE', #15705, 2.500000000000002220 ) ;
#10907=LINE ( 'NONE', #12165, #4226 ) ;
#10908=CARTESIAN_POINT ( 'NONE',  ( 30.00000000000000355, 196.6227766016838245, -13.00000000000000000 ) ) ;
#10909=CARTESIAN_POINT ( 'NONE',  ( -15.77503540472913457, 32.61497647743762229, -7.787339510197840653 ) ) ;
#10911=ORIENTED_EDGE ( 'NONE', *, *, #7545, .F. ) ;
#10914=CIRCLE ( 'NONE', #17137, 2.500000000000002220 ) ;
#10919=AXIS2_PLACEMENT_3D ( 'NONE', #16130, #9385, #5224 ) ;
#10920=EDGE_CURVE ( 'NONE', #588, #8971, #15342, .T. ) ;
#10922=CARTESIAN_POINT ( 'NONE',  ( 15.98317902225257470, 29.97876603371781457, -12.94822346880645902 ) ) ;
#10923=DIRECTION ( 'NONE',  ( 0.000000000000000000, 0.000000000000000000, 1.000000000000000000 ) ) ;
#10926=CARTESIAN_POINT ( 'NONE',  ( -78.68705929748917072, 202.4787130041031560, -16.52010876963831620 ) ) ;
#10928=CARTESIAN_POINT ( 'NONE',  ( 34.93420767853314146, 20.00000000000000000, -6.320602137672510779 ) ) ;
#10930=DIRECTION ( 'NONE',  ( -1.000000000000000000, -0.000000000000000000, -0.000000000000000000 ) ) ;
#10933=VECTOR ( 'NONE', #10169, 1000.000000000000000 ) ;
#10936=CARTESIAN_POINT ( 'NONE',  ( 35.00000000000000000, 196.6227766016838245, -12.99999999999999822 ) ) ;
#10942=EDGE_CURVE ( 'NONE', #4284, #5792, #3534, .T. ) ;
#10943=AXIS2_PLACEMENT_3D ( 'NONE', #7688, #7604, #6359 ) ;
#10944=PLANE ( 'NONE',  #5804 ) ;
#10949=ORIENTED_EDGE ( 'NONE', *, *, #10632, .F. ) ;
#10951=EDGE_CURVE ( 'NONE', #1170, #17378, #136, .T. ) ;
#10952=CARTESIAN_POINT ( 'NONE',  ( -43.00000000000000000, 171.6227766016838245, 0.000000000000000000 ) ) ;
#10954=EDGE_CURVE ( 'NONE', #5946, #15177, #4663, .T. ) ;
#10955=ADVANCED_FACE ( 'NONE', ( #9118 ), #3468, .F. ) ;
#10957=CARTESIAN_POINT ( 'NONE',  ( 18.85693063296981009, 140.6075696125688239, -16.22282984566914621 ) ) ;
#10958=AXIS2_PLACEMENT_3D ( 'NONE', #15614, #3489, #11626 ) ;
#10959=ORIENTED_EDGE ( 'NONE', *, *, #6191, .T. ) ;
#10961=CIRCLE ( 'NONE', #7004, 747.9999999999998863 ) ;
#10967=DIRECTION ( 'NONE',  ( 0.000000000000000000, -1.000000000000000000, 0.000000000000000000 ) ) ;
#10968=CARTESIAN_POINT ( 'NONE',  ( 34.80468147095351128, 17.99999999999999645, -7.619145204522578041 ) ) ;
#10969=LINE ( 'NONE', #16393, #11504 ) ;
#10971=VECTOR ( 'NONE', #12355, 1000.000000000000000 ) ;
#10972=CARTESIAN_POINT ( 'NONE',  ( 49.99999999999998579, 191.6227766016837677, -3.071800142134975431 ) ) ;
#10973=AXIS2_PLACEMENT_3D ( 'NONE', #5832, #13714, #9902 ) ;
#10976=CARTESIAN_POINT ( 'NONE',  ( -19.80886414215398261, 19.99999999999999645, -20.97268729564270728 ) ) ;
#10978=DIRECTION ( 'NONE',  ( -1.000000000000000000, -0.000000000000000000, 0.000000000000000000 ) ) ;
#10979=CARTESIAN_POINT ( 'NONE',  ( 36.00000000000000711, 196.6227766016838245, -24.49489742783179125 ) ) ;
#10982=CARTESIAN_POINT ( 'NONE',  ( -85.00000000000002842, 146.6227766016838245, -35.00200000000000244 ) ) ;
#10983=EDGE_CURVE ( 'NONE', #793, #9467, #10450, .T. ) ;
#10984=ORIENTED_EDGE ( 'NONE', *, *, #16290, .T. ) ;
#10985=EDGE_CURVE ( 'NONE', #14433, #9729, #14190, .T. ) ;
#10986=AXIS2_PLACEMENT_3D ( 'NONE', #3771, #14832, #5458 ) ;
#10991=CARTESIAN_POINT ( 'NONE',  ( 15.60228996708978855, 124.9392590763941371, 1.387778780781445676E-14 ) ) ;
#10993=EDGE_LOOP ( 'NONE', ( #15714, #16613, #15363, #8632 ) ) ;
#10995=VERTEX_POINT ( 'NONE', #15507 ) ;
#10996=CARTESIAN_POINT ( 'NONE',  ( 23.67803828928656884, 138.9414820825090544, -12.55787835418278675 ) ) ;
#10999=CARTESIAN_POINT ( 'NONE',  ( -86.34904889156064201, 192.6231533511310374, -25.45681811525071225 ) ) ;
#11002=DIRECTION ( 'NONE',  ( 1.000000000000000000, 0.000000000000000000, -0.000000000000000000 ) ) ;
#11005=CARTESIAN_POINT ( 'NONE',  ( -16.30611068361787019, 32.76923076923078781, 0.000000000000000000 ) ) ;
#11006=ADVANCED_FACE ( 'NONE', ( #6210 ), #8855, .F. ) ;
#11009=EDGE_CURVE ( 'NONE', #10138, #10436, #6915, .T. ) ;
#11012=EDGE_LOOP ( 'NONE', ( #7567, #11210, #8322, #15947 ) ) ;
#11015=VECTOR ( 'NONE', #12057, 1000.000000000000000 ) ;
#11020=EDGE_LOOP ( 'NONE', ( #4016, #5620 ) ) ;
#11023=CARTESIAN_POINT ( 'NONE',  ( -24.94987437106622252, 100.0000000000000142, -6.000000000000000000 ) ) ;
#11024=CARTESIAN_POINT ( 'NONE',  ( -45.00000000000000000, 122.0000000000000142, -15.00000000000000000 ) ) ;
#11028=AXIS2_PLACEMENT_3D ( 'NONE', #6813, #16008, #12019 ) ;
#11029=ORIENTED_EDGE ( 'NONE', *, *, #1318, .T. ) ;
#11030=EDGE_CURVE ( 'NONE', #13521, #4808, #7531, .T. ) ;
#11033=VERTEX_POINT ( 'NONE', #17013 ) ;
#11036=DIRECTION ( 'NONE',  ( 0.000000000000000000, -1.000000000000000000, 0.000000000000000000 ) ) ;
#11037=CARTESIAN_POINT ( 'NONE',  ( -77.50000000000001421, 196.6227766016838245, -16.00000000000000000 ) ) ;
#11038=AXIS2_PLACEMENT_3D ( 'NONE', #9624, #14685, #2902 ) ;
#11039=AXIS2_PLACEMENT_3D ( 'NONE', #15096, #16188, #2811 ) ;
#11041=DIRECTION ( 'NONE',  ( -1.000000000000000000, -0.000000000000000000, 0.000000000000000000 ) ) ;
#11042=CARTESIAN_POINT ( 'NONE',  ( 48.00000000000000711, 191.6227766016837677, -8.071800142134975431 ) ) ;
#11047=VECTOR ( 'NONE', #9420, 1000.000000000000000 ) ;
#11048=CARTESIAN_POINT ( 'NONE',  ( 17.52204077229825785, 125.6458339596819798, -5.684362142990314837 ) ) ;
#11049=VERTEX_POINT ( 'NONE', #3732 ) ;
#11051=CARTESIAN_POINT ( 'NONE',  ( 15.26338903195270547, 125.9505563168691111, -6.751637631526196337 ) ) ;
#11053=CARTESIAN_POINT ( 'NONE',  ( -82.40832088953489176, 191.1229741556853128, -29.06467671913510031 ) ) ;
#11054=EDGE_CURVE ( 'NONE', #11464, #16539, #11954, .T. ) ;
#11058=CARTESIAN_POINT ( 'NONE',  ( -15.00000000000002665, 130.0000000000000000, -15.00000000000000000 ) ) ;
#11059=DIRECTION ( 'NONE',  ( -1.000000000000000000, 0.000000000000000000, 5.782411586589356653E-16 ) ) ;
#11060=CIRCLE ( 'NONE', #325, 2.500000000000002220 ) ;
#11064=ORIENTED_EDGE ( 'NONE', *, *, #5964, .T. ) ;
#11065=ORIENTED_EDGE ( 'NONE', *, *, #7151, .F. ) ;
#11066=FACE_OUTER_BOUND ( 'NONE', #8539, .T. ) ;
#11067=DIRECTION ( 'NONE',  ( -1.000000000000000000, -0.000000000000000000, -0.000000000000000000 ) ) ;
#11068=VERTEX_POINT ( 'NONE', #13557 ) ;
#11071=ORIENTED_EDGE ( 'NONE', *, *, #16534, .T. ) ;
#11074=( BOUNDED_SURFACE ( )  B_SPLINE_SURFACE ( 3, 2, ( 
 ( #5132, #9018, #11847 ),
 ( #6547, #10519, #14688 ),
 ( #3794, #962, #9281 ),
 ( #2471, #2571, #1228 ),
 ( #17340, #10701, #13017 ),
 ( #7958, #16117, #7769 ),
 ( #3990, #890, #6278 ),
 ( #11668, #17077, #4946 ),
 ( #7863, #10341, #17255 ),
 ( #3628, #2296, #11754 ),
 ( #17165, #13277, #5038 ),
 ( #10431, #15844, #9103 ),
 ( #13447, #253, #10957 ),
 ( #16463, #1412, #1495 ),
 ( #2988, #8038, #159 ),
 ( #6816, #16281, #13538 ),
 ( #4153, #10864, #2905 ),
 ( #9712, #12470, #2648 ),
 ( #1317, #4326, #13704 ),
 ( #6886, #11126, #12209 ),
 ( #4242, #6724, #338 ),
 ( #9446, #5477, #8217 ),
 ( #1579, #12123, #5740 ),
 ( #13806, #5565, #6978 ),
 ( #16544, #16376, #4068 ),
 ( #14856, #9374, #14776 ),
 ( #12285, #7563, #9627 ),
 ( #15027, #5399, #8389 ),
 ( #11048, #8294, #1674 ),
 ( #12377, #75, #7072 ) ),
 .UNSPECIFIED., .F., .F., .F. ) 
 B_SPLINE_SURFACE_WITH_KNOTS ( ( 4, 2, 2, 2, 2, 2, 2, 2, 2, 2, 2, 2, 2, 2, 4 ),
 ( 3, 3 ),
 ( 0.01165250788892074896, 0.01579789672993320987, 0.01787059115043944033, 0.01890693836069255729, 0.01994328557094567078, 0.02408867441195813169, 0.02616136883246436215, 0.02823406325297059261, 0.03030675767347682306, 0.03237945209398305352, 0.03652484093499551443, 0.03859753535550174142, 0.03963388256575485491, 0.04067022977600797534, 0.04481561861702043625 ),
 ( 0.000000000000000000, 1.000000000000000000 ),
 .UNSPECIFIED. ) 
 GEOMETRIC_REPRESENTATION_ITEM ( )  RATIONAL_B_SPLINE_SURFACE ( (
 ( 1.000000000000000000, 0.8819171036881967574, 1.000000000000000000),
 ( 1.000000000000000000, 0.8793942645247267986, 1.000000000000000000),
 ( 1.000000000000000000, 0.8749458316895478704, 1.000000000000000000),
 ( 1.000000000000000000, 0.8656814021268812720, 1.000000000000000000),
 ( 1.000000000000000000, 0.8621600075896179716, 1.000000000000000000),
 ( 1.000000000000000000, 0.8562492930711324002, 1.000000000000000000),
 ( 1.000000000000000000, 0.8541736901085718037, 1.000000000000000000),
 ( 1.000000000000000000, 0.8498659178639272893, 1.000000000000000000),
 ( 1.000000000000000000, 0.8476283308601378907, 1.000000000000000000),
 ( 1.000000000000000000, 0.8360458749412158497, 1.000000000000000000),
 ( 1.000000000000000000, 0.8255221978280062878, 1.000000000000000000),
 ( 1.000000000000000000, 0.8082270345002190437, 1.000000000000000000),
 ( 1.000000000000000000, 0.8022128341710524913, 1.000000000000000000),
 ( 1.000000000000000000, 0.7899684886178014454, 1.000000000000000000),
 ( 1.000000000000000000, 0.7837128169315926707, 1.000000000000000000),
 ( 1.000000000000000000, 0.7710263478624882483, 1.000000000000000000),
 ( 1.000000000000000000, 0.7645952338536526893, 1.000000000000000000),
 ( 1.000000000000000000, 0.7516613202048504361, 1.000000000000000000),
 ( 1.000000000000000000, 0.7451386183437513910, 1.000000000000000000),
 ( 1.000000000000000000, 0.7257808243684673588, 1.000000000000000000),
 ( 1.000000000000000000, 0.7133953845776390690, 1.000000000000000000),
 ( 1.000000000000000000, 0.6965170042221164870, 1.000000000000000000),
 ( 1.000000000000000000, 0.6911767420095684678, 1.000000000000000000),
 ( 1.000000000000000000, 0.6837405640632492343, 1.000000000000000000),
 ( 1.000000000000000000, 0.6813577907325653049, 1.000000000000000000),
 ( 1.000000000000000000, 0.6768117804539316440, 1.000000000000000000),
 ( 1.000000000000000000, 0.6746439590912862716, 1.000000000000000000),
 ( 1.000000000000000000, 0.6645663254999056857, 1.000000000000000000),
 ( 1.000000000000000000, 0.6588263891901358082, 1.000000000000000000),
 ( 1.000000000000000000, 0.6558243695371221982, 1.000000000000000000) ) ) 
 REPRESENTATION_ITEM ( '' )  SURFACE ( )  );
#11075=CARTESIAN_POINT ( 'NONE',  ( -24.99999999999999289, 90.00000000000000000, 0.000000000000000000 ) ) ;
#11076=DIRECTION ( 'NONE',  ( -0.000000000000000000, -0.000000000000000000, -1.000000000000000000 ) ) ;
#11077=CARTESIAN_POINT ( 'NONE',  ( 37.25061104762458797, 194.6575378623844585, -23.63707964515041482 ) ) ;
#11078=CARTESIAN_POINT ( 'NONE',  ( -34.99999999999999289, 120.0000000000000284, -4.999999999999999112 ) ) ;
#11081=ORIENTED_EDGE ( 'NONE', *, *, #14694, .F. ) ;
#11086=CARTESIAN_POINT ( 'NONE',  ( -100.0000000000000000, 120.0000000000000284, -6.000000000000001776 ) ) ;
#11088=ORIENTED_EDGE ( 'NONE', *, *, #5752, .T. ) ;
#11093=ORIENTED_EDGE ( 'NONE', *, *, #2820, .T. ) ;
#11097=CYLINDRICAL_SURFACE ( 'NONE', #10631, 5.000000000000004441 ) ;
#11098=DIRECTION ( 'NONE',  ( 1.000000000000000000, 0.000000000000000000, 0.000000000000000000 ) ) ;
#11101=ORIENTED_EDGE ( 'NONE', *, *, #12702, .T. ) ;
#11104=ADVANCED_FACE ( 'NONE', ( #2587 ), #1163, .F. ) ;
#11106=EDGE_CURVE ( 'NONE', #4216, #1489, #9187, .T. ) ;
#11107=CARTESIAN_POINT ( 'NONE',  ( 21.38845554303141938, 19.99999999999999289, -23.94082098111162082 ) ) ;
#11109=PLANE ( 'NONE',  #2732 ) ;
#11110=ADVANCED_FACE ( 'NONE', ( #11955 ), #14709, .F. ) ;
#11112=VERTEX_POINT ( 'NONE', #9820 ) ;
#11113=DIRECTION ( 'NONE',  ( -1.000000000000000000, 0.000000000000000000, 0.000000000000000000 ) ) ;
#11114=VERTEX_POINT ( 'NONE', #5753 ) ;
#11117=PLANE ( 'NONE',  #13310 ) ;
#11120=CYLINDRICAL_SURFACE ( 'NONE', #12876, 7.499999999999996447 ) ;
#11121=ORIENTED_EDGE ( 'NONE', *, *, #1030, .T. ) ;
#11125=DIRECTION ( 'NONE',  ( 0.000000000000000000, 0.000000000000000000, 1.000000000000000000 ) ) ;
#11126=CARTESIAN_POINT ( 'NONE',  ( 16.25737266305939599, 136.9911583880083015, -7.117438641154834045 ) ) ;
#11129=EDGE_LOOP ( 'NONE', ( #1740, #11845 ) ) ;
#11131=CARTESIAN_POINT ( 'NONE',  ( -85.03936963251346981, 193.3606217133605583, -27.43184792633612545 ) ) ;
#11134=EDGE_CURVE ( 'NONE', #9063, #15728, #7765, .T. ) ;
#11135=CARTESIAN_POINT ( 'NONE',  ( 49.99999999999998579, 179.6227766016838245, -12.50000337241049309 ) ) ;
#11139=FACE_BOUND ( 'NONE', #14973, .T. ) ;
#11146=ORIENTED_EDGE ( 'NONE', *, *, #11588, .T. ) ;
#11150=ORIENTED_EDGE ( 'NONE', *, *, #8256, .F. ) ;
#11151=CARTESIAN_POINT ( 'NONE',  ( 35.45105639388463459, 151.7804781109684313, -26.36917907415268658 ) ) ;
#11152=CIRCLE ( 'NONE', #8621, 20.00000000000000355 ) ;
#11153=DIRECTION ( 'NONE',  ( 0.000000000000000000, 0.000000000000000000, 1.000000000000000000 ) ) ;
#11154=CIRCLE ( 'NONE', #4388, 2.500000000000002220 ) ;
#11160=FACE_OUTER_BOUND ( 'NONE', #12587, .T. ) ;
#11163=EDGE_CURVE ( 'NONE', #9872, #6476, #1839, .T. ) ;
#11166=ADVANCED_FACE ( 'NONE', ( #11139, #3101, #1594, #433, #8498, #13911, #1772, #7167, #2919, #16743, #4608, #15393, #12565, #11235 ), #8674, .F. ) ;
#11167=CARTESIAN_POINT ( 'NONE',  ( -72.50701606102703067, 196.2445469595302825, -21.97388680505723713 ) ) ;
#11174=DIRECTION ( 'NONE',  ( -0.000000000000000000, -0.000000000000000000, 1.000000000000000000 ) ) ;
#11175=VECTOR ( 'NONE', #8556, 1000.000000000000000 ) ;
#11177=ORIENTED_EDGE ( 'NONE', *, *, #10942, .T. ) ;
#11188=CARTESIAN_POINT ( 'NONE',  ( -74.03485743176636902, 197.3601060891146233, -23.72478281133074063 ) ) ;
#11190=CARTESIAN_POINT ( 'NONE',  ( 28.15871609335591685, 19.99999999999999289, -20.05978710182010971 ) ) ;
#11196=VECTOR ( 'NONE', #13875, 1000.000000000000000 ) ;
#11197=ORIENTED_EDGE ( 'NONE', *, *, #9481, .F. ) ;
#11198=DIRECTION ( 'NONE',  ( -0.000000000000000000, -0.000000000000000000, 1.000000000000000000 ) ) ;
#11203=EDGE_CURVE ( 'NONE', #2935, #457, #356, .T. ) ;
#11206=DIRECTION ( 'NONE',  ( 1.000000000000000000, 0.000000000000000000, 0.000000000000000000 ) ) ;
#11207=CARTESIAN_POINT ( 'NONE',  ( 18.23439605415255471, 29.93382634594462743, -12.29196570735054728 ) ) ;
#11210=ORIENTED_EDGE ( 'NONE', *, *, #4147, .F. ) ;
#11213=VECTOR ( 'NONE', #2262, 1000.000000000000000 ) ;
#11214=CARTESIAN_POINT ( 'NONE',  ( -27.98221281347037959, 20.00000000000000000, 15.00000000000000000 ) ) ;
#11215=COLOUR_RGB ( '', 0.08235294, 0.09019608, 0.10196078) ;
#11218=AXIS2_PLACEMENT_3D ( 'NONE', #11507, #13019, #12664 ) ;
#11222=ORIENTED_EDGE ( 'NONE', *, *, #3935, .T. ) ;
#11223=EDGE_CURVE ( 'NONE', #9797, #2837, #8624, .T. ) ;
#11226=CARTESIAN_POINT ( 'NONE',  ( 196.0000000000000000, 175.6227766016838530, -19.42820660268601074 ) ) ;
#11229=CARTESIAN_POINT ( 'NONE',  ( 27.48361012698968864, 136.6227766016838245, 0.000000000000000000 ) ) ;
#11235=FACE_OUTER_BOUND ( 'NONE', #8987, .T. ) ;
#11236=EDGE_LOOP ( 'NONE', ( #1004, #8148 ) ) ;
#11237=VECTOR ( 'NONE', #8741, 1000.000000000000000 ) ;
#11241=CARTESIAN_POINT ( 'NONE',  ( -95.00000000000000000, 171.6227766016838245, 0.000000000000000000 ) ) ;
#11242=ORIENTED_EDGE ( 'NONE', *, *, #12573, .T. ) ;
#11245=FACE_OUTER_BOUND ( 'NONE', #10700, .T. ) ;
#11246=ORIENTED_EDGE ( 'NONE', *, *, #8084, .T. ) ;
#11247=CARTESIAN_POINT ( 'NONE',  ( 31.17267072074456991, 154.0361450035975110, -27.92332374485729218 ) ) ;
#11248=VECTOR ( 'NONE', #5654, 1000.000000000000000 ) ;
#11259=ORIENTED_EDGE ( 'NONE', *, *, #10942, .F. ) ;
#11262=VECTOR ( 'NONE', #7534, 1000.000000000000114 ) ;
#11263=VERTEX_POINT ( 'NONE', #9185 ) ;
#11265=DIRECTION ( 'NONE',  ( 0.000000000000000000, 0.000000000000000000, -1.000000000000000000 ) ) ;
#11266=AXIS2_PLACEMENT_3D ( 'NONE', #4601, #14416, #10071 ) ;
#11269=EDGE_LOOP ( 'NONE', ( #7816, #15953, #4301 ) ) ;
#11271=DIRECTION ( 'NONE',  ( -1.000000000000000000, 0.000000000000000000, 0.000000000000000000 ) ) ;
#11274=CARTESIAN_POINT ( 'NONE',  ( -74.00000000000002842, 146.6227766016838245, -35.00000000000000000 ) ) ;
#11275=ADVANCED_FACE ( 'NONE', ( #10698, #4151 ), #6630, .T. ) ;
#11277=AXIS2_PLACEMENT_3D ( 'NONE', #14243, #11662, #17070 ) ;
#11278=CARTESIAN_POINT ( 'NONE',  ( -38.00000000000000000, 2.000000000000000000, 0.000000000000000000 ) ) ;
#11284=DIRECTION ( 'NONE',  ( -0.000000000000000000, -0.000000000000000000, 1.000000000000000000 ) ) ;
#11288=FACE_BOUND ( 'NONE', #11888, .T. ) ;
#11291=EDGE_LOOP ( 'NONE', ( #1610, #15089, #13846, #11574 ) ) ;
#11293=AXIS2_PLACEMENT_3D ( 'NONE', #7233, #12985, #3248 ) ;
#11295=CIRCLE ( 'NONE', #11570, 2.499999999999998668 ) ;
#11296=ORIENTED_EDGE ( 'NONE', *, *, #5854, .T. ) ;
#11298=VERTEX_POINT ( 'NONE', #14774 ) ;
#11302=DIRECTION ( 'NONE',  ( 0.000000000000000000, 0.000000000000000000, 1.000000000000000000 ) ) ;
#11303=VERTEX_POINT ( 'NONE', #8033 ) ;
#11305=AXIS2_PLACEMENT_3D ( 'NONE', #7219, #4654, #17100 ) ;
#11308=DIRECTION ( 'NONE',  ( -1.000000000000000000, 0.000000000000000000, 0.000000000000000000 ) ) ;
#11309=AXIS2_PLACEMENT_3D ( 'NONE', #11226, #6894, #9544 ) ;
#11310=CARTESIAN_POINT ( 'NONE',  ( -12.16365208422963740, 31.05675767351161909, -14.01395464075509878 ) ) ;
#11312=ADVANCED_FACE ( 'NONE', ( #13444 ), #1314, .T. ) ;
#11316=AXIS2_PLACEMENT_3D ( 'NONE', #12817, #16805, #1931 ) ;
#11317=AXIS2_PLACEMENT_3D ( 'NONE', #10697, #16112, #3986 ) ;
#11323=EDGE_LOOP ( 'NONE', ( #13448, #419, #11633, #16451 ) ) ;
#11325=CARTESIAN_POINT ( 'NONE',  ( 34.93420767853316988, 20.00000000000000000, -4.999999999999999112 ) ) ;
#11327=VERTEX_POINT ( 'NONE', #10516 ) ;
#11335=EDGE_CURVE ( 'NONE', #5097, #9988, #15026, .T. ) ;
#11336=ORIENTED_EDGE ( 'NONE', *, *, #15034, .T. ) ;
#11337=CARTESIAN_POINT ( 'NONE',  ( 24.52650527911658074, 19.99999999999999645, -8.254754350130129481 ) ) ;
#11339=EDGE_LOOP ( 'NONE', ( #7759, #13423, #9665, #1324 ) ) ;
#11342=VERTEX_POINT ( 'NONE', #4414 ) ;
#11350=CARTESIAN_POINT ( 'NONE',  ( 48.00000000000000711, 167.6227766016838530, -5.571800142134975431 ) ) ;
#11355=VECTOR ( 'NONE', #5511, 1000.000000000000000 ) ;
#11356=CARTESIAN_POINT ( 'NONE',  ( 48.00000000000000711, 146.6227766016838245, -4.592425496802573578E-15 ) ) ;
#11357=EDGE_LOOP ( 'NONE', ( #4261, #4098, #10605, #946 ) ) ;
#11366=CARTESIAN_POINT ( 'NONE',  ( 196.0000000000000000, 183.6227766016837961, -3.071800142134975431 ) ) ;
#11367=ADVANCED_FACE ( 'NONE', ( #16543 ), #2822, .F. ) ;
#11374=EDGE_LOOP ( 'NONE', ( #4394, #7334, #7638, #16457 ) ) ;
#11376=DIRECTION ( 'NONE',  ( 0.000000000000000000, 0.000000000000000000, 1.000000000000000000 ) ) ;
#11382=SURFACE_SIDE_STYLE ('',( #14138 ) ) ;
#11383=ORIENTED_EDGE ( 'NONE', *, *, #15984, .F. ) ;
#11385=CARTESIAN_POINT ( 'NONE',  ( -23.00000000000000000, 120.0000000000000284, 0.000000000000000000 ) ) ;
#11388=CARTESIAN_POINT ( 'NONE',  ( 49.99999999999998579, 175.6227766016838530, -19.42820660268601074 ) ) ;
#11389=ORIENTED_EDGE ( 'NONE', *, *, #7889, .T. ) ;
#11393=CARTESIAN_POINT ( 'NONE',  ( -13.34744738361370509, 19.99999999999999645, -11.18154278182822026 ) ) ;
#11396=EDGE_CURVE ( 'NONE', #12075, #9019, #415, .T. ) ;
#11399=DIRECTION ( 'NONE',  ( -1.000000000000000000, 0.000000000000000000, 0.000000000000000000 ) ) ;
#11401=LINE ( 'NONE', #14163, #14153 ) ;
#11402=DIRECTION ( 'NONE',  ( 1.000000000000000000, 0.000000000000000000, -0.000000000000000000 ) ) ;
#11405=VERTEX_POINT ( 'NONE', #1572 ) ;
#11406=FACE_OUTER_BOUND ( 'NONE', #14294, .T. ) ;
#11410=ORIENTED_EDGE ( 'NONE', *, *, #6037, .T. ) ;
#11411=CARTESIAN_POINT ( 'NONE',  ( 21.59801423301730239, 19.99999999999999645, -12.60094170202890140 ) ) ;
#11413=ORIENTED_EDGE ( 'NONE', *, *, #16700, .F. ) ;
#11415=CARTESIAN_POINT ( 'NONE',  ( 7.863372401969320968, 140.4786490112420552, -12.74411896114139076 ) ) ;
#11416=ORIENTED_EDGE ( 'NONE', *, *, #13623, .T. ) ;
#11420=ADVANCED_FACE ( 'NONE', ( #2985 ), #8385, .F. ) ;
#11421=EDGE_CURVE ( 'NONE', #14117, #14296, #12888, .T. ) ;
#11424=CIRCLE ( 'NONE', #12842, 2.500000000000002220 ) ;
#11425=DIRECTION ( 'NONE',  ( -0.000000000000000000, -0.000000000000000000, -1.000000000000000000 ) ) ;
#11428=LINE ( 'NONE', #7103, #16254 ) ;
#11434=PLANE ( 'NONE',  #2998 ) ;
#11435=VERTEX_POINT ( 'NONE', #9972 ) ;
#11436=CARTESIAN_POINT ( 'NONE',  ( 15.00000000000000000, 171.6227766016838245, 0.000000000000000000 ) ) ;
#11437=CIRCLE ( 'NONE', #13703, 7.500000000000000000 ) ;
#11438=VECTOR ( 'NONE', #3293, 1000.000000000000000 ) ;
#11440=LINE ( 'NONE', #16852, #6728 ) ;
#11445=CARTESIAN_POINT ( 'NONE',  ( 27.99999999999998224, 9.999999999999998224, -30.00000000000001066 ) ) ;
#11447=DIRECTION ( 'NONE',  ( 0.000000000000000000, 0.000000000000000000, -1.000000000000000000 ) ) ;
#11448=DIRECTION ( 'NONE',  ( 0.000000000000000000, 0.000000000000000000, -1.000000000000000000 ) ) ;
#11451=EDGE_LOOP ( 'NONE', ( #9531, #15303 ) ) ;
#11452=DIRECTION ( 'NONE',  ( -1.000000000000000000, -0.000000000000000000, 0.000000000000000000 ) ) ;
#11454=CARTESIAN_POINT ( 'NONE',  ( -27.29618490519992591, 19.99999999999999645, -10.29570512375934399 ) ) ;
#11455=ORIENTED_EDGE ( 'NONE', *, *, #8737, .T. ) ;
#11457=LINE ( 'NONE', #842, #5548 ) ;
#11462=EDGE_CURVE ( 'NONE', #8600, #10173, #14018, .T. ) ;
#11463=CIRCLE ( 'NONE', #8352, 2.500000000000000444 ) ;
#11464=VERTEX_POINT ( 'NONE', #1929 ) ;
#11465=CYLINDRICAL_SURFACE ( 'NONE', #7369, 20.00000000000000355 ) ;
#11466=VECTOR ( 'NONE', #3694, 1000.000000000000000 ) ;
#11468=CIRCLE ( 'NONE', #13737, 5.000000000000000888 ) ;
#11471=ORIENTED_EDGE ( 'NONE', *, *, #15055, .F. ) ;
#11476=CARTESIAN_POINT ( 'NONE',  ( -21.36854569161992856, 19.99999999999999645, -19.70709815271291632 ) ) ;
#11478=AXIS2_PLACEMENT_3D ( 'NONE', #3559, #12855, #14269 ) ;
#11479=VECTOR ( 'NONE', #1895, 1000.000000000000000 ) ;
#11488=CIRCLE ( 'NONE', #10644, 27.69059892324149530 ) ;
#11489=DIRECTION ( 'NONE',  ( 0.000000000000000000, 0.000000000000000000, 1.000000000000000000 ) ) ;
#11492=CARTESIAN_POINT ( 'NONE',  ( 10.69994788061133129, 131.5490474681699880, -11.88030112651796877 ) ) ;
#11493=EDGE_CURVE ( 'NONE', #1489, #4216, #17113, .T. ) ;
#11494=VECTOR ( 'NONE', #2378, 1000.000000000000000 ) ;
#11496=DIRECTION ( 'NONE',  ( 1.000000000000000000, 0.000000000000000000, 0.000000000000000000 ) ) ;
#11497=DIRECTION ( 'NONE',  ( 1.000000000000000000, 0.000000000000000000, 0.000000000000000000 ) ) ;
#11498=CARTESIAN_POINT ( 'NONE',  ( 49.99999999999998579, 155.6227766016839098, -10.00000337241049309 ) ) ;
#11499=CARTESIAN_POINT ( 'NONE',  ( 28.02291439894537817, 202.2921397697441819, -16.86471387523355858 ) ) ;
#11502=CARTESIAN_POINT ( 'NONE',  ( 21.98114852961611376, 19.99999999999999645, -23.72829316725777460 ) ) ;
#11503=CARTESIAN_POINT ( 'NONE',  ( 196.0000000000000000, 179.6227766016838245, -15.00000337241049486 ) ) ;
#11504=VECTOR ( 'NONE', #15038, 1000.000000000000000 ) ;
#11507=CARTESIAN_POINT ( 'NONE',  ( 30.00000000000000355, 196.6227766016838245, -35.00200000000000244 ) ) ;
#11509=CARTESIAN_POINT ( 'NONE',  ( -100.0000000000000000, 171.6227766016838245, -27.69059892324149175 ) ) ;
#11511=PLANE ( 'NONE',  #14700 ) ;
#11512=CARTESIAN_POINT ( 'NONE',  ( -100.0000000000000000, 141.2912748254776147, -13.00000000000000000 ) ) ;
#11518=CARTESIAN_POINT ( 'NONE',  ( 32.41004031834387433, 141.1235162643941408, -17.17043012754695397 ) ) ;
#11520=CARTESIAN_POINT ( 'NONE',  ( -68.00000000000000000, 171.6227766016838245, -20.00000000000000355 ) ) ;
#11521=VERTEX_POINT ( 'NONE', #4850 ) ;
#11522=DIRECTION ( 'NONE',  ( -0.000000000000000000, -0.000000000000000000, -1.000000000000000000 ) ) ;
#11524=DIRECTION ( 'NONE',  ( -1.156482317317868274E-16, 1.000000000000000000, 0.000000000000000000 ) ) ;
#11526=ORIENTED_EDGE ( 'NONE', *, *, #17231, .T. ) ;
#11528=CIRCLE ( 'NONE', #8705, 2.500000000000002220 ) ;
#11531=AXIS2_PLACEMENT_3D ( 'NONE', #8224, #13636, #346 ) ;
#11532=( GEOMETRIC_REPRESENTATION_CONTEXT ( 3 ) GLOBAL_UNCERTAINTY_ASSIGNED_CONTEXT ( ( #3463 ) ) GLOBAL_UNIT_ASSIGNED_CONTEXT ( ( #1037, #9088, #13082 ) ) REPRESENTATION_CONTEXT ( 'NONE', 'WORKASPACE' ) );
#11536=LINE ( 'NONE', #17028, #1458 ) ;
#11538=CARTESIAN_POINT ( 'NONE',  ( -40.00000000000000000, 0.000000000000000000, -33.00000000000000711 ) ) ;
#11539=EDGE_LOOP ( 'NONE', ( #2695, #12365, #16595, #1003, #15993 ) ) ;
#11543=VERTEX_POINT ( 'NONE', #7667 ) ;
#11546=FACE_BOUND ( 'NONE', #2504, .T. ) ;
#11547=EDGE_CURVE ( 'NONE', #4330, #4930, #15561, .T. ) ;
#11554=CYLINDRICAL_SURFACE ( 'NONE', #14925, 6.000000000000001776 ) ;
#11556=ORIENTED_EDGE ( 'NONE', *, *, #5788, .F. ) ;
#11557=CARTESIAN_POINT ( 'NONE',  ( 24.93507336697353693, 29.86842105263157876, 0.000000000000000000 ) ) ;
#11560=DIRECTION ( 'NONE',  ( 0.000000000000000000, 0.000000000000000000, 1.000000000000000000 ) ) ;
#11564=FACE_BOUND ( 'NONE', #16064, .T. ) ;
#11567=CARTESIAN_POINT ( 'NONE',  ( -16.77496435665412733, 32.01311153724419967, -10.06041171812362300 ) ) ;
#11569=CIRCLE ( 'NONE', #8178, 2.500000000000000444 ) ;
#11570=AXIS2_PLACEMENT_3D ( 'NONE', #17094, #8238, #14621 ) ;
#11572=ORIENTED_EDGE ( 'NONE', *, *, #13013, .F. ) ;
#11574=ORIENTED_EDGE ( 'NONE', *, *, #6887, .T. ) ;
#11577=AXIS2_PLACEMENT_3D ( 'NONE', #14883, #12310, #16567 ) ;
#11578=DIRECTION ( 'NONE',  ( -0.000000000000000000, -0.000000000000000000, 1.000000000000000000 ) ) ;
#11579=CIRCLE ( 'NONE', #3967, 2.500000000000002220 ) ;
#11581=B_SPLINE_CURVE_WITH_KNOTS ( 'NONE', 3,
 ( #4819, #4731, #2065, #2149, #2242, #16947, #7550, #3406, #7716, #15685, #15876, #3485, #10209, #12959, #833, #6228, #3568, #2411, #9054, #10117, #13219, #11791, #17196, #11622, #16859, #8800 ),
 .UNSPECIFIED., .F., .F.,
 ( 4, 2, 2, 2, 2, 2, 2, 2, 2, 2, 2, 2, 4 ),
 ( 0.000000000000000000, 0.002066677509289960735, 0.003100016263934941754, 0.004133355018579923205, 0.006200032527869886109, 0.007233371282514866260, 0.008266710037159848146, 0.01033338754644981018, 0.01136672630109478513, 0.01240006505573976354, 0.01446674256502970997, 0.01550008131967467971, 0.01653342007431965119 ),
 .UNSPECIFIED. ) ;
#11584=CARTESIAN_POINT ( 'NONE',  ( -25.00000000000002132, 130.0000000000000000, -15.00000000000000000 ) ) ;
#11587=CARTESIAN_POINT ( 'NONE',  ( -34.99999999999999289, 130.0000000000000000, 0.000000000000000000 ) ) ;
#11588=EDGE_CURVE ( 'NONE', #13136, #12617, #3773, .T. ) ;
#11589=CARTESIAN_POINT ( 'NONE',  ( 32.97919343609721921, 201.8349995435116568, -17.67084604013262705 ) ) ;
#11591=VERTEX_POINT ( 'NONE', #17227 ) ;
#11592=CARTESIAN_POINT ( 'NONE',  ( 17.52239125723112778, 29.96525225773407186, -14.66037399604394942 ) ) ;
#11593=CIRCLE ( 'NONE', #17254, 250.0000000000000000 ) ;
#11602=CYLINDRICAL_SURFACE ( 'NONE', #6393, 2.500000000000000444 ) ;
#11603=CYLINDRICAL_SURFACE ( 'NONE', #8050, 6.000000000000005329 ) ;
#11609=ORIENTED_EDGE ( 'NONE', *, *, #8585, .F. ) ;
#11610=CARTESIAN_POINT ( 'NONE',  ( 49.99999999999998579, 167.6227766016838814, -21.92820660268601074 ) ) ;
#11611=ORIENTED_EDGE ( 'NONE', *, *, #1642, .T. ) ;
#11616=DIRECTION ( 'NONE',  ( 0.000000000000000000, 0.000000000000000000, 1.000000000000000000 ) ) ;
#11617=EDGE_CURVE ( 'NONE', #6590, #7472, #16089, .T. ) ;
#11620=EDGE_LOOP ( 'NONE', ( #3739, #15950, #2803, #10479 ) ) ;
#11621=LINE ( 'NONE', #11693, #5260 ) ;
#11622=CARTESIAN_POINT ( 'NONE',  ( -18.23240235453911140, 32.30379688028049401, -5.697301546657946858 ) ) ;
#11625=ORIENTED_EDGE ( 'NONE', *, *, #8652, .F. ) ;
#11626=DIRECTION ( 'NONE',  ( 0.000000000000000000, 0.000000000000000000, 1.000000000000000000 ) ) ;
#11628=CARTESIAN_POINT ( 'NONE',  ( -86.00000000000001421, 196.6227766016838245, -24.49489742783178770 ) ) ;
#11630=CARTESIAN_POINT ( 'NONE',  ( 28.21992570506699494, 190.8885537947572573, -29.22050223063088481 ) ) ;
#11631=CARTESIAN_POINT ( 'NONE',  ( -23.00000000000001421, 122.0000000000000284, -4.999999999999999112 ) ) ;
#11632=ORIENTED_EDGE ( 'NONE', *, *, #11923, .T. ) ;
#11633=ORIENTED_EDGE ( 'NONE', *, *, #2304, .F. ) ;
#11636=ORIENTED_EDGE ( 'NONE', *, *, #16170, .F. ) ;
#11638=CARTESIAN_POINT ( 'NONE',  ( 196.0000000000000000, 155.6227766016839098, -12.50000337241049309 ) ) ;
#11642=DIRECTION ( 'NONE',  ( -1.000000000000000000, 0.000000000000000000, 0.000000000000000000 ) ) ;
#11651=CARTESIAN_POINT ( 'NONE',  ( -85.00000000000002842, 196.6227766016838245, -35.00200000000000244 ) ) ;
#11653=ORIENTED_EDGE ( 'NONE', *, *, #13790, .T. ) ;
#11656=EDGE_LOOP ( 'NONE', ( #12184, #4279, #298, #13673, #11088 ) ) ;
#11658=LINE ( 'NONE', #4857, #2215 ) ;
#11659=DIRECTION ( 'NONE',  ( -0.000000000000000000, -0.000000000000000000, 1.000000000000000000 ) ) ;
#11662=DIRECTION ( 'NONE',  ( -0.000000000000000000, -0.000000000000000000, 1.000000000000000000 ) ) ;
#11664=CARTESIAN_POINT ( 'NONE',  ( 34.99288146128931487, 199.9683764595548610, -20.53727899274374380 ) ) ;
#11665=ORIENTED_EDGE ( 'NONE', *, *, #4504, .T. ) ;
#11666=ORIENTED_EDGE ( 'NONE', *, *, #12889, .F. ) ;
#11667=CARTESIAN_POINT ( 'NONE',  ( 17.20299680575017831, 29.96951112202298262, -14.74034971990100296 ) ) ;
#11668=CARTESIAN_POINT ( 'NONE',  ( 9.986687348566183786, 132.8041431104223307, -14.33374896416919064 ) ) ;
#11671=DIRECTION ( 'NONE',  ( 0.000000000000000000, 0.000000000000000000, 1.000000000000000000 ) ) ;
#11673=CARTESIAN_POINT ( 'NONE',  ( 48.00000000000000711, 155.6227766016839098, -12.50000337241049309 ) ) ;
#11677=DIRECTION ( 'NONE',  ( -0.000000000000000000, -0.000000000000000000, 1.000000000000000000 ) ) ;
#11680=DIRECTION ( 'NONE',  ( 0.000000000000000000, 0.000000000000000000, 1.000000000000000000 ) ) ;
#11689=EDGE_CURVE ( 'NONE', #1773, #16806, #6317, .T. ) ;
#11690=AXIS2_PLACEMENT_3D ( 'NONE', #17067, #3706, #9092 ) ;
#11693=CARTESIAN_POINT ( 'NONE',  ( 25.00000000000000711, 146.6227766016838245, -35.00200000000000244 ) ) ;
#11694=CARTESIAN_POINT ( 'NONE',  ( 24.37944869002583914, 191.6508168144186186, -26.22852547856965444 ) ) ;
#11696=CARTESIAN_POINT ( 'NONE',  ( 17.00000000000000000, 171.6227766016838245, -20.00000000000000355 ) ) ;
#11697=CARTESIAN_POINT ( 'NONE',  ( -11.48222079042285770, 17.99999999999884182, -9.976350980977374050 ) ) ;
#11698=EDGE_CURVE ( 'NONE', #13265, #12106, #16571, .T. ) ;
#11701=CARTESIAN_POINT ( 'NONE',  ( -23.00000000000000000, 120.0000000000000284, 0.000000000000000000 ) ) ;
#11703=CARTESIAN_POINT ( 'NONE',  ( 24.13852584367151266, 195.3295718346067531, -25.74952675241122080 ) ) ;
#11706=B_SPLINE_CURVE_WITH_KNOTS ( 'NONE', 3,
 ( #14868, #6735, #14784, #1334, #16128, #2658, #12136, #8049, #88, #1425, #6, #4077, #17445, #9457, #5577, #2748, #6825, #12217, #5487, #14703, #15037, #10873, #10968, #16293, #9548 ),
 .UNSPECIFIED., .F., .F.,
 ( 4, 2, 2, 1, 2, 2, 2, 2, 2, 2, 2, 2, 4 ),
 ( 0.000000000000000000, 0.003937549356687076833, 0.005906324035030613949, 0.007875098713374151932, 0.009843873391717689048, 0.01181264807006122616, 0.01575019742674830733, 0.01771897210509184445, 0.01968774678343538503, 0.02362529614012245927, 0.02559407081846599985, 0.02756284549680953697, 0.03150039485349661467 ),
 .UNSPECIFIED. ) ;
#11707=ORIENTED_EDGE ( 'NONE', *, *, #13053, .T. ) ;
#11710=EDGE_LOOP ( 'NONE', ( #9953, #10852 ) ) ;
#11711=ORIENTED_EDGE ( 'NONE', *, *, #13570, .F. ) ;
#11712=EDGE_CURVE ( 'NONE', #15641, #1170, #12615, .T. ) ;
#11713=CARTESIAN_POINT ( 'NONE',  ( -73.52759457847471936, 150.4190785964221106, -25.28784208911848452 ) ) ;
#11714=ORIENTED_EDGE ( 'NONE', *, *, #6382, .T. ) ;
#11716=CIRCLE ( 'NONE', #4109, 8.000000000000000000 ) ;
#11717=CARTESIAN_POINT ( 'NONE',  ( 28.41545104427121515, 152.4141840272156401, -29.25805444611330230 ) ) ;
#11722=CARTESIAN_POINT ( 'NONE',  ( 23.07174175064647059, 29.89240369784053897, -10.82181213433699618 ) ) ;
#11723=PLANE ( 'NONE',  #8488 ) ;
#11725=ORIENTED_EDGE ( 'NONE', *, *, #3171, .F. ) ;
#11732=ORIENTED_EDGE ( 'NONE', *, *, #3616, .F. ) ;
#11734=AXIS2_PLACEMENT_3D ( 'NONE', #11388, #14146, #6075 ) ;
#11735=DIRECTION ( 'NONE',  ( -1.000000000000000000, -0.000000000000000000, -0.000000000000000000 ) ) ;
#11736=( BOUNDED_SURFACE ( )  B_SPLINE_SURFACE ( 3, 2, ( 
 ( #3349, #7412, #7326 ),
 ( #12302, #1928, #5914 ),
 ( #606, #511, #6903 ),
 ( #2921, #8824, #8310 ),
 ( #12735, #13726, #15373 ),
 ( #16981, #10236, #6081 ),
 ( #9644, #14230, #10054 ),
 ( #11310, #3250, #16724 ),
 ( #8653, #9971, #2018 ),
 ( #6003, #4590, #1596 ),
 ( #8744, #14154, #10976 ),
 ( #3433, #11393, #4668 ),
 ( #15469, #685, #11476 ),
 ( #6999, #4763, #10150 ),
 ( #15560, #2092, #7488 ),
 ( #12900, #776, #6171 ),
 ( #11567, #4849, #15043 ),
 ( #15634, #8236, #13643 ),
 ( #1509, #4262, #5186 ),
 ( #3692, #12987, #6331 ),
 ( #1119, #17317, #3599 ),
 ( #6522, #867, #9165 ),
 ( #13075, #14571, #13250 ),
 ( #5105, #7579, #10401 ) ),
 .UNSPECIFIED., .F., .F., .F. ) 
 B_SPLINE_SURFACE_WITH_KNOTS ( ( 4, 2, 2, 2, 2, 2, 2, 2, 2, 2, 2, 4 ),
 ( 3, 3 ),
 ( 0.01427588378380419132, 0.01824401167166925936, 0.02022807561560179684, 0.02221213955953433086, 0.02618026744739940237, 0.02816433139133193639, 0.03014839533526447041, 0.03411652322312953844, 0.03610058716706207593, 0.03808465111099461342, 0.04205277899885968146, 0.04602090688672474950 ),
 ( 0.000000000000000000, 1.000000000000000000 ),
 .UNSPECIFIED. ) 
 GEOMETRIC_REPRESENTATION_ITEM ( )  RATIONAL_B_SPLINE_SURFACE ( (
 ( 1.000000000000000000, 0.7071067811865476838, 1.000000000000000000),
 ( 1.000000000000000000, 0.7013659285814082267, 1.000000000000000000),
 ( 1.000000000000000000, 0.6957352470443716186, 1.000000000000000000),
 ( 1.000000000000000000, 0.6874449304735253952, 1.000000000000000000),
 ( 1.000000000000000000, 0.6847075230359779274, 1.000000000000000000),
 ( 1.000000000000000000, 0.6792848743381553200, 1.000000000000000000),
 ( 1.000000000000000000, 0.6765866164121365767, 1.000000000000000000),
 ( 1.000000000000000000, 0.6687223666254397125, 1.000000000000000000),
 ( 1.000000000000000000, 0.6637534122518267132, 1.000000000000000000),
 ( 1.000000000000000000, 0.6567012635110727192, 1.000000000000000000),
 ( 1.000000000000000000, 0.6544178910915308123, 1.000000000000000000),
 ( 1.000000000000000000, 0.6499901663949341213, 1.000000000000000000),
 ( 1.000000000000000000, 0.6478648508491323676, 1.000000000000000000),
 ( 1.000000000000000000, 0.6418284244073564349, 1.000000000000000000),
 ( 1.000000000000000000, 0.6382188548936990058, 1.000000000000000000),
 ( 1.000000000000000000, 0.6334349500989927551, 1.000000000000000000),
 ( 1.000000000000000000, 0.6319385063094495880, 1.000000000000000000),
 ( 1.000000000000000000, 0.6292162870119188955, 1.000000000000000000),
 ( 1.000000000000000000, 0.6279881568154176419, 1.000000000000000000),
 ( 1.000000000000000000, 0.6246939197237179053, 1.000000000000000000),
 ( 1.000000000000000000, 0.6230139244305938906, 1.000000000000000000),
 ( 1.000000000000000000, 0.6207349535630983794, 1.000000000000000000),
 ( 1.000000000000000000, 0.6201739322037901347, 1.000000000000000000),
 ( 1.000000000000000000, 0.6201736729460421982, 1.000000000000000000) ) ) 
 REPRESENTATION_ITEM ( '' )  SURFACE ( )  );
#11739=CARTESIAN_POINT ( 'NONE',  ( -19.68629150101526903, 125.3137084989847807, -12.99999999999998401 ) ) ;
#11741=CARTESIAN_POINT ( 'NONE',  ( -38.00000000000000000, 2.000000000000000000, 0.000000000000000000 ) ) ;
#11743=ORIENTED_EDGE ( 'NONE', *, *, #6037, .F. ) ;
#11745=DIRECTION ( 'NONE',  ( 0.000000000000000000, 0.000000000000000000, 1.000000000000000000 ) ) ;
#11748=CARTESIAN_POINT ( 'NONE',  ( 24.00000000000000355, 196.8086972563010022, -24.30514295430832306 ) ) ;
#11749=EDGE_LOOP ( 'NONE', ( #4486, #3257, #13747, #12965, #16751 ) ) ;
#11751=VERTEX_POINT ( 'NONE', #13779 ) ;
#11752=CYLINDRICAL_SURFACE ( 'NONE', #5240, 5.000000000000004441 ) ;
#11753=EDGE_LOOP ( 'NONE', ( #5088, #3497 ) ) ;
#11754=CARTESIAN_POINT ( 'NONE',  ( 15.42236477930650906, 141.4984257577436892, -17.82510376534603580 ) ) ;
#11758=CARTESIAN_POINT ( 'NONE',  ( 196.0000000000000000, 171.6227766016838245, -10.00000337241048953 ) ) ;
#11759=CARTESIAN_POINT ( 'NONE',  ( 14.63750484765316706, 138.5418767416829837, -5.508738673615532377 ) ) ;
#11770=CARTESIAN_POINT ( 'NONE',  ( -23.00000000000000000, 120.0000000000000284, -4.999999999999999112 ) ) ;
#11771=CIRCLE ( 'NONE', #6408, 2.500000000000000444 ) ;
#11773=CARTESIAN_POINT ( 'NONE',  ( 196.0000000000000000, 167.6227766016838530, -5.571800142134975431 ) ) ;
#11774=VECTOR ( 'NONE', #11642, 1000.000000000000000 ) ;
#11780=CARTESIAN_POINT ( 'NONE',  ( -23.65835920965563233, 18.00000000000000000, -17.33937328557891533 ) ) ;
#11782=CARTESIAN_POINT ( 'NONE',  ( 48.00000000000000711, 163.6227766016838530, -12.50000337241049309 ) ) ;
#11784=DIRECTION ( 'NONE',  ( 1.000000000000000000, 0.000000000000000000, 0.000000000000000000 ) ) ;
#11786=AXIS2_PLACEMENT_3D ( 'NONE', #428, #7679, #14589 ) ;
#11788=DIRECTION ( 'NONE',  ( -0.000000000000000000, -0.000000000000000000, 1.000000000000000000 ) ) ;
#11789=CIRCLE ( 'NONE', #1070, 2.499999999999998668 ) ;
#11790=CARTESIAN_POINT ( 'NONE',  ( 22.52785494716452419, 195.8611292878214272, -22.40167687543583952 ) ) ;
#11791=CARTESIAN_POINT ( 'NONE',  ( -18.09555036921010540, 32.27673591576833445, -6.733025906873759681 ) ) ;
#11792=CARTESIAN_POINT ( 'NONE',  ( -13.23954943057894873, 31.86042443463173157, -11.05847410484002680 ) ) ;
#11796=ADVANCED_FACE ( 'NONE', ( #16446 ), #15276, .F. ) ;
#11797=CARTESIAN_POINT ( 'NONE',  ( 31.13603083703002383, 190.7269353522202664, -29.32635129980145194 ) ) ;
#11798=DIRECTION ( 'NONE',  ( 1.000000000000000000, 0.000000000000000000, 0.000000000000000000 ) ) ;
#11803=ADVANCED_FACE ( 'NONE', ( #12266 ), #9689, .T. ) ;
#11804=CARTESIAN_POINT ( 'NONE',  ( -87.50000000000004263, 146.6227766016838245, -21.54065922853802562 ) ) ;
#11806=EDGE_CURVE ( 'NONE', #8380, #6279, #15087, .T. ) ;
#11809=CYLINDRICAL_SURFACE ( 'NONE', #6521, 2.500000000000000444 ) ;
#11816=CARTESIAN_POINT ( 'NONE',  ( 30.00000000000001066, 146.6227766016838245, -35.00200000000000244 ) ) ;
#11817=CARTESIAN_POINT ( 'NONE',  ( 14.93242934743711992, 30.00000000000000000, -15.00000000000000000 ) ) ;
#11818=DIRECTION ( 'NONE',  ( -1.000000000000000000, 0.000000000000000000, 0.000000000000000000 ) ) ;
#11820=FACE_BOUND ( 'NONE', #853, .T. ) ;
#11821=EDGE_LOOP ( 'NONE', ( #3766, #10756 ) ) ;
#11825=ORIENTED_EDGE ( 'NONE', *, *, #14310, .T. ) ;
#11827=AXIS2_PLACEMENT_3D ( 'NONE', #16971, #4839, #16717 ) ;
#11834=VECTOR ( 'NONE', #7672, 1000.000000000000000 ) ;
#11836=ORIENTED_EDGE ( 'NONE', *, *, #13166, .T. ) ;
#11839=CARTESIAN_POINT ( 'NONE',  ( 50.00000000000000000, 146.6227766016838245, 0.000000000000000000 ) ) ;
#11842=CARTESIAN_POINT ( 'NONE',  ( -95.00000000000000000, 171.6227766016838245, 0.000000000000000000 ) ) ;
#11845=ORIENTED_EDGE ( 'NONE', *, *, #15009, .T. ) ;
#11847=CARTESIAN_POINT ( 'NONE',  ( 6.134011831684059501, 142.5209969267753820, -19.44444444444444642 ) ) ;
#11848=VERTEX_POINT ( 'NONE', #318 ) ;
#11849=LINE ( 'NONE', #11758, #5283 ) ;
#11850=CARTESIAN_POINT ( 'NONE',  ( 11.37136921290580460, 130.9041960856249318, -11.49611652308843901 ) ) ;
#11851=AXIS2_PLACEMENT_3D ( 'NONE', #10234, #4918, #7486 ) ;
#11854=DIRECTION ( 'NONE',  ( 0.000000000000000000, 0.000000000000000000, 1.000000000000000000 ) ) ;
#11855=CIRCLE ( 'NONE', #2546, 20.00000000000000355 ) ;
#11856=CARTESIAN_POINT ( 'NONE',  ( 24.10793207926302983, 201.2861523353439566, -14.48313018527311868 ) ) ;
#11859=CARTESIAN_POINT ( 'NONE',  ( 23.09107716886297013, 17.99999999998395239, -5.538990817933217237 ) ) ;
#11862=ADVANCED_FACE ( 'NONE', ( #5720, #5798 ), #11109, .T. ) ;
#11863=EDGE_CURVE ( 'NONE', #8522, #8669, #8459, .T. ) ;
#11864=CARTESIAN_POINT ( 'NONE',  ( 48.00000000000000711, 179.6227766016838245, -10.00000337241049309 ) ) ;
#11866=CARTESIAN_POINT ( 'NONE',  ( 32.60692063061733137, 141.2146784997055988, -17.33162689407163981 ) ) ;
#11867=VERTEX_POINT ( 'NONE', #3151 ) ;
#11868=CARTESIAN_POINT ( 'NONE',  ( -38.00000000000000000, 18.00000000000000355, 0.000000000000000000 ) ) ;
#11870=CIRCLE ( 'NONE', #4803, 2.500000000000000444 ) ;
#11874=CARTESIAN_POINT ( 'NONE',  ( -12.63167751028164965, 18.00000000000000000, -24.35243221814330994 ) ) ;
#11878=VERTEX_POINT ( 'NONE', #13610 ) ;
#11879=DIRECTION ( 'NONE',  ( 0.000000000000000000, 1.000000000000000000, 0.000000000000000000 ) ) ;
#11883=DIRECTION ( 'NONE',  ( -1.000000000000000000, 0.000000000000000000, 0.000000000000000000 ) ) ;
#11884=CARTESIAN_POINT ( 'NONE',  ( -23.00000000000000000, 120.0000000000000284, -4.999999999999999112 ) ) ;
#11885=CARTESIAN_POINT ( 'NONE',  ( -22.80699178664539772, 18.00000000000000000, -18.33022619056923119 ) ) ;
#11888=EDGE_LOOP ( 'NONE', ( #6800, #4677 ) ) ;
#11889=CARTESIAN_POINT ( 'NONE',  ( 24.22171959708801481, 194.9977432358044780, -26.05112671349591125 ) ) ;
#11890=CARTESIAN_POINT ( 'NONE',  ( -85.89206792073701990, 201.2861523353439281, -14.48313018527312046 ) ) ;
#11894=VERTEX_POINT ( 'NONE', #1815 ) ;
#11902=EDGE_CURVE ( 'NONE', #16058, #3793, #4133, .T. ) ;
#11903=CARTESIAN_POINT ( 'NONE',  ( 27.00066514940125018, 151.8237148210351108, -28.86201951371925034 ) ) ;
#11904=AXIS2_PLACEMENT_3D ( 'NONE', #17493, #5452, #4212 ) ;
#11908=LINE ( 'NONE', #6516, #8420 ) ;
#11911=DIRECTION ( 'NONE',  ( -1.000000000000000000, 0.000000000000000000, 0.000000000000000000 ) ) ;
#11923=EDGE_CURVE ( 'NONE', #4046, #4814, #17424, .T. ) ;
#11924=CARTESIAN_POINT ( 'NONE',  ( 19.14963388379466736, 18.00000000000000000, -24.55317681541934149 ) ) ;
#11926=DIRECTION ( 'NONE',  ( 2.312964634635742464E-16, 0.000000000000000000, 1.000000000000000000 ) ) ;
#11928=DIRECTION ( 'NONE',  ( 0.000000000000000000, 0.000000000000000000, 1.000000000000000000 ) ) ;
#11929=EDGE_CURVE ( 'NONE', #11970, #8095, #1999, .T. ) ;
#11934=CARTESIAN_POINT ( 'NONE',  ( 35.83620472812211943, 198.0598900292994529, -22.94241666008127822 ) ) ;
#11935=EDGE_CURVE ( 'NONE', #16184, #14270, #3000, .T. ) ;
#11940=CARTESIAN_POINT ( 'NONE',  ( -78.22656196874415002, 152.3723237521624014, -29.23070922465766941 ) ) ;
#11941=CARTESIAN_POINT ( 'NONE',  ( 18.85693063297101801, 142.3798671548016159, -15.29581099734062022 ) ) ;
#11942=EDGE_LOOP ( 'NONE', ( #9649, #7928 ) ) ;
#11943=EDGE_CURVE ( 'NONE', #14947, #8170, #11457, .T. ) ;
#11946=CARTESIAN_POINT ( 'NONE',  ( 22.50000000000000000, 196.6227766016838245, -21.54065922853802562 ) ) ;
#11952=CYLINDRICAL_SURFACE ( 'NONE', #8167, 7.500000000000007105 ) ;
#11953=FACE_OUTER_BOUND ( 'NONE', #15539, .T. ) ;
#11954=B_SPLINE_CURVE_WITH_KNOTS ( 'NONE', 3,
 ( #12942, #4879, #10268, #4961, #12850, #6471, #2392, #10355, #2051, #13198, #7786, #11866, #11518, #4800, #15671, #17274, #14355, #2221, #7617, #8784, #727, #16928, #13032, #902, #6289, #6564, #1430, #5416, #1340, #93, #4170, #8147, #14614, #7975, #12140, #13376, #1507, #9464, #3815, #2754, #6831, #14792 ),
 .UNSPECIFIED., .F., .F.,
 ( 4, 2, 2, 2, 2, 2, 2, 2, 2, 2, 2, 2, 2, 2, 2, 2, 2, 2, 2, 2, 4 ),
 ( 0.000000000000000000, 0.003174452718035283925, 0.004761679077052946921, 0.006348905436070610350, 0.007936131795088273780, 0.009523358154105937209, 0.01031697133361475678, 0.01111058451312357809, 0.01190419769263239939, 0.01230100428238680571, 0.01269781087214121203, 0.01349142405165002466, 0.01428503723115883729, 0.01507865041066764993, 0.01587226359017646082, 0.01745948994919411384, 0.01904671630821176340, 0.02063394266722941295, 0.02222116902624706250, 0.02380839538526471552, 0.02539562174428236160 ),
 .UNSPECIFIED. ) ;
#11955=FACE_OUTER_BOUND ( 'NONE', #4651, .T. ) ;
#11961=CARTESIAN_POINT ( 'NONE',  ( -10.03891356649073785, 18.00000000000000355, -24.87483525495233394 ) ) ;
#11962=ORIENTED_EDGE ( 'NONE', *, *, #11943, .F. ) ;
#11963=CARTESIAN_POINT ( 'NONE',  ( 17.00000000000000000, 204.6227766016838245, 2.020667218593133100E-15 ) ) ;
#11966=EDGE_LOOP ( 'NONE', ( #8602, #12452 ) ) ;
#11967=ADVANCED_FACE ( 'NONE', ( #16868 ), #754, .F. ) ;
#11970=VERTEX_POINT ( 'NONE', #11631 ) ;
#11974=CARTESIAN_POINT ( 'NONE',  ( -10.04118010627651181, 18.00000000000000000, -24.87462214922868142 ) ) ;
#11977=ORIENTED_EDGE ( 'NONE', *, *, #3171, .T. ) ;
#11978=CARTESIAN_POINT ( 'NONE',  ( -85.08563460989527982, 191.1044234702846722, -26.63673872167001377 ) ) ;
#11981=ORIENTED_EDGE ( 'NONE', *, *, #11929, .T. ) ;
#11984=ADVANCED_FACE ( 'NONE', ( #1907, #7398, #11288, #10131, #15356, #7304, #8725, #15536, #2249, #11546, #4650, #15618, #3493, #3328 ), #16702, .T. ) ;
#11985=CARTESIAN_POINT ( 'NONE',  ( -80.56347832044305335, 154.1240291517870276, -27.97845313684488033 ) ) ;
#11988=CARTESIAN_POINT ( 'NONE',  ( 13.65319468153969318, 138.6827642935804192, -2.302653601785663362 ) ) ;
#11989=DIRECTION ( 'NONE',  ( 1.000000000000000000, 0.000000000000000000, 0.000000000000000000 ) ) ;
#11990=CARTESIAN_POINT ( 'NONE',  ( 35.55667557412272828, 148.9132954376224802, -26.63594553516329455 ) ) ;
#11991=DIRECTION ( 'NONE',  ( 0.000000000000000000, 0.000000000000000000, 1.000000000000000000 ) ) ;
#11993=AXIS2_PLACEMENT_3D ( 'NONE', #12445, #4219, #16258 ) ;
#11995=VERTEX_POINT ( 'NONE', #16062 ) ;
#11996=CARTESIAN_POINT ( 'NONE',  ( -78.21870694796302814, 202.3573166656175317, -16.74530232247013828 ) ) ;
#12000=FACE_OUTER_BOUND ( 'NONE', #12162, .T. ) ;
#12004=EDGE_CURVE ( 'NONE', #10173, #17455, #6961, .T. ) ;
#12005=DIRECTION ( 'NONE',  ( -1.000000000000000000, -0.000000000000000000, 0.000000000000000000 ) ) ;
#12014=CARTESIAN_POINT ( 'NONE',  ( -75.92798022420988957, 142.2001748967346941, -18.96071578072434249 ) ) ;
#12017=CARTESIAN_POINT ( 'NONE',  ( 49.99999999999998579, 183.6227766016837961, -8.071800142134975431 ) ) ;
#12019=DIRECTION ( 'NONE',  ( 0.000000000000000000, 0.000000000000000000, 1.000000000000000000 ) ) ;
#12020=DIRECTION ( 'NONE',  ( 0.000000000000000000, 0.000000000000000000, 1.000000000000000000 ) ) ;
#12026=TOROIDAL_SURFACE ( 'NONE', #14291, 25.00000000000000000, 8.000000000000000000 ) ;
#12028=ORIENTED_EDGE ( 'NONE', *, *, #12113, .T. ) ;
#12029=CARTESIAN_POINT ( 'NONE',  ( -80.47498095768615656, 152.6213468612616566, -29.39295273708632550 ) ) ;
#12030=CARTESIAN_POINT ( 'NONE',  ( 14.40174056114590151, 138.5906827818587885, -4.212836247846349025 ) ) ;
#12035=EDGE_CURVE ( 'NONE', #12970, #1757, #1097, .T. ) ;
#12036=AXIS2_PLACEMENT_3D ( 'NONE', #2723, #67, #5554 ) ;
#12037=DIRECTION ( 'NONE',  ( 0.000000000000000000, 0.000000000000000000, 1.000000000000000000 ) ) ;
#12041=CARTESIAN_POINT ( 'NONE',  ( 31.20232444244219394, 18.00000000000000000, -16.65183244245019623 ) ) ;
#12043=CARTESIAN_POINT ( 'NONE',  ( -95.00000000000000000, 201.6227766016838245, -1.836970198721029589E-15 ) ) ;
#12044=CARTESIAN_POINT ( 'NONE',  ( 0.000000000000000000, 0.000000000000000000, 0.000000000000000000 ) ) ;
#12046=CARTESIAN_POINT ( 'NONE',  ( -45.00000000000000000, 122.0000000000000142, 0.000000000000000000 ) ) ;
#12047=ORIENTED_EDGE ( 'NONE', *, *, #1362, .T. ) ;
#12050=AXIS2_PLACEMENT_3D ( 'NONE', #12255, #129, #5530 ) ;
#12052=AXIS2_PLACEMENT_3D ( 'NONE', #7049, #6873, #5542 ) ;
#12056=ORIENTED_EDGE ( 'NONE', *, *, #10444, .F. ) ;
#12057=DIRECTION ( 'NONE',  ( -0.8660254037844378194, -0.5000000000000015543, -0.000000000000000000 ) ) ;
#12058=EDGE_LOOP ( 'NONE', ( #14551, #12773 ) ) ;
#12059=DIRECTION ( 'NONE',  ( 0.000000000000000000, -1.000000000000000000, 1.836970198721028701E-16 ) ) ;
#12063=CARTESIAN_POINT ( 'NONE',  ( 48.00000000000000711, 159.6227766016838814, -5.571800142134975431 ) ) ;
#12067=ORIENTED_EDGE ( 'NONE', *, *, #13974, .F. ) ;
#12073=ORIENTED_EDGE ( 'NONE', *, *, #2212, .F. ) ;
#12075=VERTEX_POINT ( 'NONE', #13057 ) ;
#12077=VECTOR ( 'NONE', #14170, 1000.000000000000000 ) ;
#12085=CARTESIAN_POINT ( 'NONE',  ( 29.07646442517566854, 152.5685199100059322, -29.35899209070759142 ) ) ;
#12102=CIRCLE ( 'NONE', #7287, 9.999999999999998224 ) ;
#12103=CARTESIAN_POINT ( 'NONE',  ( 6.134011831684053284, 134.2062027339443944, -25.00000000000000000 ) ) ;
#12106=VERTEX_POINT ( 'NONE', #15791 ) ;
#12107=CIRCLE ( 'NONE', #7850, 7.500000000000003553 ) ;
#12108=CARTESIAN_POINT ( 'NONE',  ( 27.99999999999998224, 9.999999999999998224, -13.00000000000000000 ) ) ;
#12112=CARTESIAN_POINT ( 'NONE',  ( -78.69116039514727845, 140.7623173628079485, -16.51208758287213030 ) ) ;
#12113=EDGE_CURVE ( 'NONE', #15648, #3748, #15606, .T. ) ;
#12120=VECTOR ( 'NONE', #13294, 1000.000000000000000 ) ;
#12121=AXIS2_PLACEMENT_3D ( 'NONE', #1567, #5731, #13528 ) ;
#12122=VERTEX_POINT ( 'NONE', #5079 ) ;
#12123=CARTESIAN_POINT ( 'NONE',  ( 16.35719767791491819, 136.8501131444031387, -5.449348266248646766 ) ) ;
#12125=CARTESIAN_POINT ( 'NONE',  ( -74.95697939493170736, 149.8947795965756029, -27.44208088385415323 ) ) ;
#12126=CARTESIAN_POINT ( 'NONE',  ( 22.72753210816364700, 141.1551838527312555, -12.68377836492884470 ) ) ;
#12132=AXIS2_PLACEMENT_3D ( 'NONE', #13953, #7397, #7131 ) ;
#12133=CARTESIAN_POINT ( 'NONE',  ( -80.00000000000002842, 146.6227766016838245, 1.387778780781445676E-14 ) ) ;
#12136=CARTESIAN_POINT ( 'NONE',  ( 22.61491075001043782, 18.00000000000000000, -23.50024419593056635 ) ) ;
#12137=CARTESIAN_POINT ( 'NONE',  ( 22.12396056536369215, 29.85772992373802026, -8.548742771607255264 ) ) ;
#12138=CARTESIAN_POINT ( 'NONE',  ( 30.00000000000000355, 196.6227766016838245, -16.00000000000000000 ) ) ;
#12140=CARTESIAN_POINT ( 'NONE',  ( 25.01160876918508791, 143.2703805450037180, -20.52792728560773483 ) ) ;
#12141=ORIENTED_EDGE ( 'NONE', *, *, #15281, .F. ) ;
#12142=CARTESIAN_POINT ( 'NONE',  ( 6.134011831684053284, 134.2062027339443944, -15.00000000000000000 ) ) ;
#12145=EDGE_CURVE ( 'NONE', #4581, #13903, #13401, .T. ) ;
#12147=CARTESIAN_POINT ( 'NONE',  ( 16.17028938446068764, 143.0439382767918346, -16.49999999999050360 ) ) ;
#12148=VECTOR ( 'NONE', #6127, 1000.000000000000000 ) ;
#12149=ORIENTED_EDGE ( 'NONE', *, *, #2314, .T. ) ;
#12151=AXIS2_PLACEMENT_3D ( 'NONE', #9000, #14412, #5193 ) ;
#12154=CARTESIAN_POINT ( 'NONE',  ( -74.00000000000001421, 196.6227766016838245, -24.49489742783179125 ) ) ;
#12156=DIRECTION ( 'NONE',  ( -0.000000000000000000, -0.000000000000000000, -1.000000000000000000 ) ) ;
#12157=CARTESIAN_POINT ( 'NONE',  ( 49.99999999999998579, 175.6227766016838245, -8.071800142134975431 ) ) ;
#12159=LINE ( 'NONE', #8163, #7668 ) ;
#12162=EDGE_LOOP ( 'NONE', ( #16561, #5238, #1846, #8564 ) ) ;
#12165=CARTESIAN_POINT ( 'NONE',  ( -34.99999999999999289, 120.0000000000000284, -15.00000000000000000 ) ) ;
#12166=CARTESIAN_POINT ( 'NONE',  ( 25.00000000000000000, 196.6227766016838245, 0.000000000000000000 ) ) ;
#12167=EDGE_CURVE ( 'NONE', #17455, #15648, #4033, .T. ) ;
#12168=VERTEX_POINT ( 'NONE', #8079 ) ;
#12179=DIRECTION ( 'NONE',  ( 0.000000000000000000, 0.000000000000000000, -1.000000000000000000 ) ) ;
#12180=DIRECTION ( 'NONE',  ( -1.000000000000000000, 0.000000000000000000, 0.000000000000000000 ) ) ;
#12182=CYLINDRICAL_SURFACE ( 'NONE', #11904, 33.00000000000000000 ) ;
#12184=ORIENTED_EDGE ( 'NONE', *, *, #1031, .T. ) ;
#12185=CARTESIAN_POINT ( 'NONE',  ( -80.25501005280430888, 202.6234830987601185, -16.24672887513765929 ) ) ;
#12186=CIRCLE ( 'NONE', #4553, 740.0000000000000000 ) ;
#12189=AXIS2_PLACEMENT_3D ( 'NONE', #16509, #9336, #2618 ) ;
#12192=DIRECTION ( 'NONE',  ( 1.000000000000000000, 0.000000000000000000, 0.000000000000000000 ) ) ;
#12193=VERTEX_POINT ( 'NONE', #12166 ) ;
#12194=AXIS2_PLACEMENT_3D ( 'NONE', #6600, #11991, #17396 ) ;
#12196=EDGE_CURVE ( 'NONE', #12777, #10642, #6927, .T. ) ;
#12198=CARTESIAN_POINT ( 'NONE',  ( -68.00000000000000000, 143.0439382767972347, -16.49999999999984368 ) ) ;
#12206=LINE ( 'NONE', #15025, #15556 ) ;
#12207=DIRECTION ( 'NONE',  ( -1.000000000000000000, 0.000000000000000000, 0.000000000000000000 ) ) ;
#12209=CARTESIAN_POINT ( 'NONE',  ( 24.34257225596279639, 138.6622241066778543, -11.80661878326775494 ) ) ;
#12211=DIRECTION ( 'NONE',  ( 8.673617379884037937E-17, 0.000000000000000000, 1.000000000000000000 ) ) ;
#12213=ORIENTED_EDGE ( 'NONE', *, *, #12196, .T. ) ;
#12215=CYLINDRICAL_SURFACE ( 'NONE', #11531, 2.499999999999998668 ) ;
#12217=CARTESIAN_POINT ( 'NONE',  ( 32.91012024024373517, 17.99999999999999645, -13.86436652238006673 ) ) ;
#12218=CARTESIAN_POINT ( 'NONE',  ( 21.03896850327811663, 17.99999999999885247, -10.35865908471247643 ) ) ;
#12220=FACE_OUTER_BOUND ( 'NONE', #11339, .T. ) ;
#12221=FACE_BOUND ( 'NONE', #2368, .T. ) ;
#12224=CARTESIAN_POINT ( 'NONE',  ( 11.67974368446408384, 131.7296502858855547, -13.62018484423547804 ) ) ;
#12225=VERTEX_POINT ( 'NONE', #2863 ) ;
#12226=CARTESIAN_POINT ( 'NONE',  ( 30.00000000000001066, 146.6227766016838245, -16.00000000000000000 ) ) ;
#12227=FACE_OUTER_BOUND ( 'NONE', #6148, .T. ) ;
#12228=ORIENTED_EDGE ( 'NONE', *, *, #11493, .T. ) ;
#12233=CARTESIAN_POINT ( 'NONE',  ( 35.08563460989521587, 152.1411297330830621, -26.63673872167000667 ) ) ;
#12235=CARTESIAN_POINT ( 'NONE',  ( -38.00000000000000000, 20.00000000000000000, -30.00000000000000355 ) ) ;
#12237=LINE ( 'NONE', #107, #11355 ) ;
#12240=VERTEX_POINT ( 'NONE', #7024 ) ;
#12243=CARTESIAN_POINT ( 'NONE',  ( -81.17267072074459122, 189.2094081997700528, -27.92332374485731350 ) ) ;
#12244=CARTESIAN_POINT ( 'NONE',  ( -100.0000000000000000, 100.0000000000000142, 0.000000000000000000 ) ) ;
#12245=CARTESIAN_POINT ( 'NONE',  ( -13.00560346926692645, 31.78932620563996281, -11.23370548922391521 ) ) ;
#12254=EDGE_CURVE ( 'NONE', #11543, #14137, #9667, .T. ) ;
#12255=CARTESIAN_POINT ( 'NONE',  ( 27.99999999999998224, 9.999999999999998224, -35.00200000000000244 ) ) ;
#12256=EDGE_CURVE ( 'NONE', #583, #2837, #2944, .T. ) ;
#12258=CARTESIAN_POINT ( 'NONE',  ( 22.88339857903067198, 29.84310082762161187, -6.047897139192784266 ) ) ;
#12259=DIRECTION ( 'NONE',  ( -0.000000000000000000, -0.000000000000000000, 1.000000000000000000 ) ) ;
#12260=CARTESIAN_POINT ( 'NONE',  ( 0.000000000000000000, 20.00000000000000000, -25.00000000000000000 ) ) ;
#12261=EDGE_LOOP ( 'NONE', ( #7498, #3135, #15070, #6236 ) ) ;
#12262=CARTESIAN_POINT ( 'NONE',  ( -85.73889985627347698, 198.4077499201237060, -22.53509453904544557 ) ) ;
#12264=CARTESIAN_POINT ( 'NONE',  ( 34.42405209918207731, 19.99999999999999289, -9.535225002503356251 ) ) ;
#12265=CARTESIAN_POINT ( 'NONE',  ( -27.99999999999998224, 10.00000000000000000, -30.00000000000000355 ) ) ;
#12266=FACE_OUTER_BOUND ( 'NONE', #1954, .T. ) ;
#12268=DIRECTION ( 'NONE',  ( 0.000000000000000000, 0.000000000000000000, 1.000000000000000000 ) ) ;
#12269=EDGE_LOOP ( 'NONE', ( #14801, #6358, #7146, #7588 ) ) ;
#12271=EDGE_LOOP ( 'NONE', ( #14315, #110 ) ) ;
#12272=CARTESIAN_POINT ( 'NONE',  ( 27.48361012698968864, 136.6227766016838245, -4.651049393634109604E-13 ) ) ;
#12273=VECTOR ( 'NONE', #8836, 1000.000000000000000 ) ;
#12275=CIRCLE ( 'NONE', #13697, 2.499999999999998668 ) ;
#12276=VERTEX_POINT ( 'NONE', #8336 ) ;
#12278=CARTESIAN_POINT ( 'NONE',  ( 36.00000000000002132, 146.6227766016838245, -16.00000000000000000 ) ) ;
#12280=EDGE_CURVE ( 'NONE', #7907, #14936, #5438, .T. ) ;
#12281=EDGE_CURVE ( 'NONE', #11114, #12895, #1626, .T. ) ;
#12282=ADVANCED_FACE ( 'NONE', ( #12427, #296 ), #16500, .T. ) ;
#12285=CARTESIAN_POINT ( 'NONE',  ( 17.19546515351294147, 126.2270863594749670, -7.189547039408070717 ) ) ;
#12289=DIRECTION ( 'NONE',  ( -1.000000000000000000, -0.000000000000000000, 0.000000000000000000 ) ) ;
#12290=ORIENTED_EDGE ( 'NONE', *, *, #16063, .T. ) ;
#12291=CARTESIAN_POINT ( 'NONE',  ( -74.68241007762553352, 193.8375574372276162, -27.04711750382526603 ) ) ;
#12294=DIRECTION ( 'NONE',  ( 0.000000000000000000, 1.000000000000000000, 0.000000000000000000 ) ) ;
#12296=DIRECTION ( 'NONE',  ( 0.000000000000000000, 0.000000000000000000, -1.000000000000000000 ) ) ;
#12301=ORIENTED_EDGE ( 'NONE', *, *, #14691, .F. ) ;
#12302=CARTESIAN_POINT ( 'NONE',  ( -8.091731396663927711, 30.16237610810089365, -15.00000000000000355 ) ) ;
#12305=ORIENTED_EDGE ( 'NONE', *, *, #9547, .T. ) ;
#12306=DIRECTION ( 'NONE',  ( 0.000000000000000000, 0.000000000000000000, -1.000000000000000000 ) ) ;
#12307=DIRECTION ( 'NONE',  ( 0.000000000000000000, 0.000000000000000000, -1.000000000000000000 ) ) ;
#12310=DIRECTION ( 'NONE',  ( 1.000000000000000000, -0.000000000000000000, 0.000000000000000000 ) ) ;
#12314=CARTESIAN_POINT ( 'NONE',  ( 36.80614408739177179, 149.8074533144823874, -24.76648413410754657 ) ) ;
#12317=VECTOR ( 'NONE', #5568, 1000.000000000000000 ) ;
#12320=FACE_OUTER_BOUND ( 'NONE', #16906, .T. ) ;
#12321=CYLINDRICAL_SURFACE ( 'NONE', #8524, 8.000000000000007105 ) ;
#12324=EDGE_CURVE ( 'NONE', #2857, #1757, #2480, .T. ) ;
#12326=AXIS2_PLACEMENT_3D ( 'NONE', #4472, #9857, #7803 ) ;
#12329=VECTOR ( 'NONE', #3230, 1000.000000000000000 ) ;
#12330=ORIENTED_EDGE ( 'NONE', *, *, #3121, .T. ) ;
#12331=CARTESIAN_POINT ( 'NONE',  ( -82.27956779150305522, 189.4719557769680591, -27.75644086540375000 ) ) ;
#12333=CARTESIAN_POINT ( 'NONE',  ( -16.30611068361785954, 32.76923076923075939, -5.287877769756280877 ) ) ;
#12342=ORIENTED_EDGE ( 'NONE', *, *, #13761, .T. ) ;
#12347=CARTESIAN_POINT ( 'NONE',  ( 20.22365234301270931, 29.89465715177047400, -11.02453202869212312 ) ) ;
#12348=CARTESIAN_POINT ( 'NONE',  ( -40.00000000000000000, 4.000000000000000000, -30.00000000000000711 ) ) ;
#12352=CARTESIAN_POINT ( 'NONE',  ( -86.00000000000001421, 196.6227766016838245, -24.49489742783178770 ) ) ;
#12355=DIRECTION ( 'NONE',  ( 0.000000000000000000, 0.000000000000000000, 1.000000000000000000 ) ) ;
#12360=EDGE_CURVE ( 'NONE', #6590, #11263, #13188, .T. ) ;
#12363=ORIENTED_EDGE ( 'NONE', *, *, #5442, .T. ) ;
#12365=ORIENTED_EDGE ( 'NONE', *, *, #5476, .T. ) ;
#12370=AXIS2_PLACEMENT_3D ( 'NONE', #16123, #5043, #13366 ) ;
#12371=ORIENTED_EDGE ( 'NONE', *, *, #9014, .F. ) ;
#12376=EDGE_CURVE ( 'NONE', #3419, #16407, #7809, .T. ) ;
#12377=CARTESIAN_POINT ( 'NONE',  ( 17.54349574104657705, 125.4948194589026684, -5.000000000000002665 ) ) ;
#12378=VECTOR ( 'NONE', #11452, 1000.000000000000000 ) ;
#12379=ORIENTED_EDGE ( 'NONE', *, *, #741, .F. ) ;
#12380=DIRECTION ( 'NONE',  ( -1.000000000000000000, -0.000000000000000000, -0.000000000000000000 ) ) ;
#12383=CARTESIAN_POINT ( 'NONE',  ( -80.00000000000001421, 196.6227766016838245, 0.000000000000000000 ) ) ;
#12388=EDGE_CURVE ( 'NONE', #15972, #4581, #5846, .T. ) ;
#12393=VECTOR ( 'NONE', #2838, 1000.000000000000000 ) ;
#12394=FACE_OUTER_BOUND ( 'NONE', #2187, .T. ) ;
#12399=CARTESIAN_POINT ( 'NONE',  ( 34.42312820345349422, 19.99999999999999645, -9.539278825327816236 ) ) ;
#12400=CARTESIAN_POINT ( 'NONE',  ( 15.78015847649388448, 143.0439382767918346, -16.49999999999050360 ) ) ;
#12407=VECTOR ( 'NONE', #8700, 1000.000000000000000 ) ;
#12408=CARTESIAN_POINT ( 'NONE',  ( 25.53529511534545549, 152.6548696709631372, -27.00480063125522889 ) ) ;
#12410=DIRECTION ( 'NONE',  ( -0.000000000000000000, -0.000000000000000000, 1.000000000000000000 ) ) ;
#12413=EDGE_CURVE ( 'NONE', #3299, #10402, #5220, .T. ) ;
#12416=CARTESIAN_POINT ( 'NONE',  ( 35.00000000000000000, 196.6227766016838245, -35.00200000000000244 ) ) ;
#12420=CARTESIAN_POINT ( 'NONE',  ( 12.22466323754103001, 142.0699085367067767, -18.75233045409083843 ) ) ;
#12422=CIRCLE ( 'NONE', #5650, 33.00000000000000000 ) ;
#12426=CIRCLE ( 'NONE', #13285, 2.500000000000002220 ) ;
#12427=FACE_OUTER_BOUND ( 'NONE', #7799, .T. ) ;
#12431=CYLINDRICAL_SURFACE ( 'NONE', #6064, 20.00000000000000355 ) ;
#12435=ORIENTED_EDGE ( 'NONE', *, *, #11712, .T. ) ;
#12438=CARTESIAN_POINT ( 'NONE',  ( -100.0000000000000000, 143.0439382767972347, -16.49999999999984368 ) ) ;
#12439=CARTESIAN_POINT ( 'NONE',  ( 16.75836516268004317, 29.96322345091821049, -12.79344305462037035 ) ) ;
#12444=CARTESIAN_POINT ( 'NONE',  ( -32.99999999999998579, 10.00000000000000000, 0.000000000000000000 ) ) ;
#12445=CARTESIAN_POINT ( 'NONE',  ( 30.00000000000001066, 146.6227766016838245, -16.00000000000000000 ) ) ;
#12446=DIRECTION ( 'NONE',  ( 8.673617379884037937E-17, 0.000000000000000000, 1.000000000000000000 ) ) ;
#12449=CIRCLE ( 'NONE', #11305, 10.00000000000000000 ) ;
#12452=ORIENTED_EDGE ( 'NONE', *, *, #9532, .T. ) ;
#12456=EDGE_CURVE ( 'NONE', #15728, #9063, #2445, .T. ) ;
#12457=CARTESIAN_POINT ( 'NONE',  ( 48.00000000000000711, 167.6227766016838814, -16.92820660268601429 ) ) ;
#12459=DIRECTION ( 'NONE',  ( 0.000000000000000000, 1.000000000000000000, 0.000000000000000000 ) ) ;
#12460=CARTESIAN_POINT ( 'NONE',  ( -95.00000000000000000, 199.3133755249253056, -1.695560166891042033E-15 ) ) ;
#12461=CARTESIAN_POINT ( 'NONE',  ( -45.00000000000000000, 130.0000000000000000, -15.00000000000000000 ) ) ;
#12463=CARTESIAN_POINT ( 'NONE',  ( 35.89206792073697017, 141.9594008680238062, -14.48313018527312046 ) ) ;
#12464=CIRCLE ( 'NONE', #7633, 7.500000000000000000 ) ;
#12469=CARTESIAN_POINT ( 'NONE',  ( 49.99999999999998579, 167.6227766016838814, -19.42820660268601074 ) ) ;
#12470=CARTESIAN_POINT ( 'NONE',  ( 15.82262738632537946, 137.2266821760960340, -8.447647312139547893 ) ) ;
#12471=ORIENTED_EDGE ( 'NONE', *, *, #8828, .F. ) ;
#12473=CARTESIAN_POINT ( 'NONE',  ( -75.17527926758620538, 150.2116474542519882, -27.68948087834226612 ) ) ;
#12474=DIRECTION ( 'NONE',  ( -0.000000000000000000, -0.000000000000000000, 1.000000000000000000 ) ) ;
#12476=CARTESIAN_POINT ( 'NONE',  ( -84.82038104795840638, 193.0449522123385862, -27.67906398090707754 ) ) ;
#12477=CARTESIAN_POINT ( 'NONE',  ( -91.33974596215561803, 206.6227766016838245, 0.000000000000000000 ) ) ;
#12479=DIRECTION ( 'NONE',  ( -1.000000000000000000, -6.938893903907228378E-16, -0.000000000000000000 ) ) ;
#12488=ORIENTED_EDGE ( 'NONE', *, *, #16551, .F. ) ;
#12489=ORIENTED_EDGE ( 'NONE', *, *, #17517, .T. ) ;
#12490=FACE_OUTER_BOUND ( 'NONE', #421, .T. ) ;
#12492=ADVANCED_FACE ( 'NONE', ( #9903 ), #1589, .T. ) ;
#12497=CARTESIAN_POINT ( 'NONE',  ( 23.91032892519173458, 151.0287754819114241, -25.78994361341036168 ) ) ;
#12498=DIRECTION ( 'NONE',  ( -1.000000000000000000, 0.000000000000000000, 0.000000000000000000 ) ) ;
#12499=FACE_OUTER_BOUND ( 'NONE', #12269, .T. ) ;
#12500=CARTESIAN_POINT ( 'NONE',  ( 27.99999999999998224, 9.999999999999998224, 1.387778780781445676E-14 ) ) ;
#12503=DIRECTION ( 'NONE',  ( -0.000000000000000000, -1.000000000000000000, 0.000000000000000000 ) ) ;
#12505=CARTESIAN_POINT ( 'NONE',  ( 27.44407568426044364, 136.8394969516870958, -3.888888888888887063 ) ) ;
#12509=ORIENTED_EDGE ( 'NONE', *, *, #13936, .F. ) ;
#12510=EDGE_CURVE ( 'NONE', #15648, #8600, #16022, .T. ) ;
#12512=EDGE_CURVE ( 'NONE', #4990, #5007, #15035, .T. ) ;
#12514=CARTESIAN_POINT ( 'NONE',  ( -3.000000000000000888, 171.6227766016838245, 0.000000000000000000 ) ) ;
#12527=CARTESIAN_POINT ( 'NONE',  ( 27.47046400057530846, 138.6909045376442009, -2.448381753924629756 ) ) ;
#12528=DIRECTION ( 'NONE',  ( -0.000000000000000000, -0.000000000000000000, 1.000000000000000000 ) ) ;
#12529=CARTESIAN_POINT ( 'NONE',  ( 25.51458778375578973, 19.99999999999999289, -21.98440010584615578 ) ) ;
#12530=FACE_OUTER_BOUND ( 'NONE', #7185, .T. ) ;
#12532=EDGE_LOOP ( 'NONE', ( #5235, #6067, #3417, #7821, #6219, #11962 ) ) ;
#12533=EDGE_CURVE ( 'NONE', #3871, #4327, #2163, .T. ) ;
#12534=ORIENTED_EDGE ( 'NONE', *, *, #3992, .T. ) ;
#12538=CARTESIAN_POINT ( 'NONE',  ( -27.99999999999998224, 10.00000000000000000, -16.00000000000000000 ) ) ;
#12540=DIRECTION ( 'NONE',  ( -1.000000000000000000, -0.000000000000000000, 0.000000000000000000 ) ) ;
#12544=CARTESIAN_POINT ( 'NONE',  ( 29.97257796258590901, 18.00000000000000000, -18.20111186907413980 ) ) ;
#12545=ORIENTED_EDGE ( 'NONE', *, *, #16680, .T. ) ;
#12548=LINE ( 'NONE', #7325, #15565 ) ;
#12549=EDGE_CURVE ( 'NONE', #1245, #10869, #9815, .T. ) ;
#12550=DIRECTION ( 'NONE',  ( -1.000000000000000000, 0.000000000000000000, 0.000000000000000000 ) ) ;
#12551=FACE_BOUND ( 'NONE', #8278, .T. ) ;
#12555=EDGE_LOOP ( 'NONE', ( #13624, #1149 ) ) ;
#12557=FACE_OUTER_BOUND ( 'NONE', #16825, .T. ) ;
#12558=FACE_OUTER_BOUND ( 'NONE', #8973, .T. ) ;
#12559=CARTESIAN_POINT ( 'NONE',  ( 196.0000000000000000, 163.6227766016838530, -15.00000337241049486 ) ) ;
#12561=CYLINDRICAL_SURFACE ( 'NONE', #11786, 30.00000000000000000 ) ;
#12564=EDGE_CURVE ( 'NONE', #2136, #4295, #424, .T. ) ;
#12565=FACE_BOUND ( 'NONE', #14304, .T. ) ;
#12568=AXIS2_PLACEMENT_3D ( 'NONE', #12770, #12503, #3204 ) ;
#12569=EDGE_LOOP ( 'NONE', ( #14237, #1353, #7789, #14069, #10518 ) ) ;
#12570=CARTESIAN_POINT ( 'NONE',  ( 34.26467700469002864, 19.99999999999999645, -10.17319632352553427 ) ) ;
#12572=ORIENTED_EDGE ( 'NONE', *, *, #15983, .T. ) ;
#12573=EDGE_CURVE ( 'NONE', #14342, #9691, #17439, .T. ) ;
#12575=EDGE_CURVE ( 'NONE', #11867, #5256, #15806, .T. ) ;
#12578=CARTESIAN_POINT ( 'NONE',  ( 34.26947555605809015, 152.8115259536290864, -27.11642929875283059 ) ) ;
#12582=CARTESIAN_POINT ( 'NONE',  ( -70.00000000000000000, 191.6227766016837961, 1.224646799147353454E-15 ) ) ;
#12585=CARTESIAN_POINT ( 'NONE',  ( 17.54349574104648823, 125.4948194589026684, -4.999999999999997335 ) ) ;
#12587=EDGE_LOOP ( 'NONE', ( #12832, #12305, #10312, #13479 ) ) ;
#12588=CARTESIAN_POINT ( 'NONE',  ( 10.42241938378121624, 142.2974014187406055, -19.10582184898306224 ) ) ;
#12589=ORIENTED_EDGE ( 'NONE', *, *, #10443, .F. ) ;
#12590=FACE_OUTER_BOUND ( 'NONE', #3491, .T. ) ;
#12596=CARTESIAN_POINT ( 'NONE',  ( -3.000000000000002665, 171.6227766016838245, 0.000000000000000000 ) ) ;
#12598=CARTESIAN_POINT ( 'NONE',  ( -68.00000000000000000, 171.6227766016838245, 0.000000000000000000 ) ) ;
#12601=CARTESIAN_POINT ( 'NONE',  ( -70.00000000000000000, 171.6227766016838245, 0.000000000000000000 ) ) ;
#12605=FACE_OUTER_BOUND ( 'NONE', #665, .T. ) ;
#12606=CARTESIAN_POINT ( 'NONE',  ( 27.99999999999998224, 9.999999999999998224, 1.387778780781445676E-14 ) ) ;
#12607=EDGE_CURVE ( 'NONE', #12225, #10138, #5933, .T. ) ;
#12610=ORIENTED_EDGE ( 'NONE', *, *, #305, .F. ) ;
#12612=DIRECTION ( 'NONE',  ( 1.000000000000000000, 0.000000000000000000, -8.673617379884037937E-17 ) ) ;
#12613=CYLINDRICAL_SURFACE ( 'NONE', #11993, 2.499999999999998668 ) ;
#12615=LINE ( 'NONE', #2885, #4416 ) ;
#12617=VERTEX_POINT ( 'NONE', #11325 ) ;
#12618=AXIS2_PLACEMENT_3D ( 'NONE', #10273, #8701, #4807 ) ;
#12621=VECTOR ( 'NONE', #15067, 1000.000000000000000 ) ;
#12627=EDGE_CURVE ( 'NONE', #5354, #583, #9071, .T. ) ;
#12629=DIRECTION ( 'NONE',  ( 0.000000000000000000, 1.000000000000000000, 2.312964634635742267E-15 ) ) ;
#12632=CIRCLE ( 'NONE', #16304, 11.99999999999999645 ) ;
#12633=CIRCLE ( 'NONE', #15462, 2.500000000000002220 ) ;
#12636=CARTESIAN_POINT ( 'NONE',  ( 39.99999999999998579, 0.000000000000000000, -30.00000000000001066 ) ) ;
#12637=AXIS2_PLACEMENT_3D ( 'NONE', #6988, #12479, #3001 ) ;
#12638=CYLINDRICAL_SURFACE ( 'NONE', #9897, 30.00000000000000000 ) ;
#12640=CARTESIAN_POINT ( 'NONE',  ( 196.0000000000000000, 163.6227766016838530, -12.50000337241049309 ) ) ;
#12641=AXIS2_PLACEMENT_3D ( 'NONE', #13902, #12380, #9449 ) ;
#12642=DIRECTION ( 'NONE',  ( 0.000000000000000000, 0.000000000000000000, 1.000000000000000000 ) ) ;
#12644=CARTESIAN_POINT ( 'NONE',  ( 27.48361012698969930, 136.6227766016838245, -1.296296296296295614 ) ) ;
#12647=AXIS2_PLACEMENT_3D ( 'NONE', #9460, #1591, #11059 ) ;
#12649=ORIENTED_EDGE ( 'NONE', *, *, #12954, .F. ) ;
#12650=CYLINDRICAL_SURFACE ( 'NONE', #16923, 10.00000000000000000 ) ;
#12660=CARTESIAN_POINT ( 'NONE',  ( 24.02621431236828187, 19.99999999999999645, -9.488192989094725860 ) ) ;
#12662=LINE ( 'NONE', #11503, #6407 ) ;
#12664=DIRECTION ( 'NONE',  ( 1.000000000000000000, 0.000000000000000000, 0.000000000000000000 ) ) ;
#12672=AXIS2_PLACEMENT_3D ( 'NONE', #13130, #15689, #7463 ) ;
#12676=FACE_OUTER_BOUND ( 'NONE', #15576, .T. ) ;
#12677=LINE ( 'NONE', #15057, #16737 ) ;
#12680=CARTESIAN_POINT ( 'NONE',  ( -72.56345771982930160, 145.5167101299680610, -20.20458554073935886 ) ) ;
#12684=DIRECTION ( 'NONE',  ( -1.000000000000000000, -6.938893903907228378E-16, -0.000000000000000000 ) ) ;
#12685=CARTESIAN_POINT ( 'NONE',  ( -26.89314795393037372, 18.00000000000000000, -11.55702759004479852 ) ) ;
#12698=DIRECTION ( 'NONE',  ( 0.000000000000000000, 0.000000000000000000, 1.000000000000000000 ) ) ;
#12700=AXIS2_PLACEMENT_3D ( 'NONE', #4987, #5078, #8877 ) ;
#12701=CARTESIAN_POINT ( 'NONE',  ( 22.50000000000000000, 196.6227766016838245, -35.00200000000000244 ) ) ;
#12702=EDGE_CURVE ( 'NONE', #7474, #10091, #15735, .T. ) ;
#12705=VERTEX_POINT ( 'NONE', #1156 ) ;
#12706=DIRECTION ( 'NONE',  ( 1.000000000000000000, 0.000000000000000000, -0.000000000000000000 ) ) ;
#12707=CARTESIAN_POINT ( 'NONE',  ( -95.00000000000000000, 171.6227766016838245, 0.000000000000000000 ) ) ;
#12714=AXIS2_PLACEMENT_3D ( 'NONE', #10952, #13894, #4500 ) ;
#12719=FACE_OUTER_BOUND ( 'NONE', #11291, .T. ) ;
#12722=ORIENTED_EDGE ( 'NONE', *, *, #17322, .F. ) ;
#12724=CARTESIAN_POINT ( 'NONE',  ( 49.99999999999998579, 187.6227766016837961, -10.00000337241049309 ) ) ;
#12730=VECTOR ( 'NONE', #13786, 1000.000000000000114 ) ;
#12731=AXIS2_PLACEMENT_3D ( 'NONE', #2371, #7509, #6351 ) ;
#12732=PLANE ( 'NONE',  #1681 ) ;
#12734=VECTOR ( 'NONE', #9002, 1000.000000000000000 ) ;
#12735=CARTESIAN_POINT ( 'NONE',  ( -10.16681828783789143, 30.62365918355438055, -14.67566226953583985 ) ) ;
#12740=ORIENTED_EDGE ( 'NONE', *, *, #6132, .T. ) ;
#12743=CIRCLE ( 'NONE', #9330, 2.500000000000002220 ) ;
#12744=EDGE_LOOP ( 'NONE', ( #7198, #14576 ) ) ;
#12745=CARTESIAN_POINT ( 'NONE',  ( -24.99999999999999645, 120.0000000000000284, 0.000000000000000000 ) ) ;
#12750=LINE ( 'NONE', #8838, #12077 ) ;
#12751=DIRECTION ( 'NONE',  ( -1.000000000000000000, -0.000000000000000000, -0.000000000000000000 ) ) ;
#12757=DIRECTION ( 'NONE',  ( 0.000000000000000000, 0.000000000000000000, 1.000000000000000000 ) ) ;
#12758=ORIENTED_EDGE ( 'NONE', *, *, #13498, .T. ) ;
#12759=DIRECTION ( 'NONE',  ( 0.000000000000000000, 1.000000000000000000, 2.312964634635742267E-15 ) ) ;
#12760=CARTESIAN_POINT ( 'NONE',  ( 7.535032041484082121, 144.1839557648053187, -18.33333333253072794 ) ) ;
#12761=ORIENTED_EDGE ( 'NONE', *, *, #16990, .F. ) ;
#12770=CARTESIAN_POINT ( 'NONE',  ( -15.00000000000002132, 100.0000000000000142, -4.999999999999999112 ) ) ;
#12773=ORIENTED_EDGE ( 'NONE', *, *, #9160, .F. ) ;
#12776=DIRECTION ( 'NONE',  ( -1.000000000000000000, 0.000000000000000000, 0.000000000000000000 ) ) ;
#12777=VERTEX_POINT ( 'NONE', #14207 ) ;
#12781=VERTEX_POINT ( 'NONE', #2066 ) ;
#12783=CARTESIAN_POINT ( 'NONE',  ( -15.00000000000001421, 19.99999999999995737, -13.00000000000000000 ) ) ;
#12786=DIRECTION ( 'NONE',  ( -1.000000000000000000, -0.000000000000000000, -0.000000000000000000 ) ) ;
#12788=CARTESIAN_POINT ( 'NONE',  ( 27.99999999999998224, 9.999999999999998224, -13.00000000000000000 ) ) ;
#12791=LINE ( 'NONE', #9951, #13227 ) ;
#12792=CARTESIAN_POINT ( 'NONE',  ( -16.40540729975244005, 20.00000000000000000, -23.03124090058168960 ) ) ;
#12793=VERTEX_POINT ( 'NONE', #6468 ) ;
#12794=EDGE_CURVE ( 'NONE', #12777, #668, #1894, .T. ) ;
#12795=CARTESIAN_POINT ( 'NONE',  ( -68.00000000000000000, 154.3022685259950038, -9.999999999999900524 ) ) ;
#12799=EDGE_CURVE ( 'NONE', #17253, #14627, #3486, .T. ) ;
#12804=VERTEX_POINT ( 'NONE', #10531 ) ;
#12809=CARTESIAN_POINT ( 'NONE',  ( 35.27494917608787972, 141.2912748254776147, -13.00000000000000000 ) ) ;
#12810=ORIENTED_EDGE ( 'NONE', *, *, #9529, .T. ) ;
#12814=FACE_OUTER_BOUND ( 'NONE', #17306, .T. ) ;
#12817=CARTESIAN_POINT ( 'NONE',  ( 225.0000000000000000, 89.99999999999997158, -15.00000000000000000 ) ) ;
#12818=ORIENTED_EDGE ( 'NONE', *, *, #10012, .T. ) ;
#12820=ORIENTED_EDGE ( 'NONE', *, *, #1362, .F. ) ;
#12822=LINE ( 'NONE', #16989, #3366 ) ;
#12824=ORIENTED_EDGE ( 'NONE', *, *, #9891, .T. ) ;
#12827=EDGE_CURVE ( 'NONE', #17297, #846, #1042, .T. ) ;
#12830=CARTESIAN_POINT ( 'NONE',  ( 25.93937429209274015, 201.0559264674919007, -18.94433901724532276 ) ) ;
#12831=EDGE_LOOP ( 'NONE', ( #12488, #10813, #6484, #16071 ) ) ;
#12832=ORIENTED_EDGE ( 'NONE', *, *, #1988, .T. ) ;
#12833=CARTESIAN_POINT ( 'NONE',  ( 19.38030756396766563, 20.00000000000112621, -14.02844645440659654 ) ) ;
#12834=CARTESIAN_POINT ( 'NONE',  ( 16.87754908408646415, 142.8876428028120813, -16.22928829806427942 ) ) ;
#12835=ORIENTED_EDGE ( 'NONE', *, *, #7811, .T. ) ;
#12842=AXIS2_PLACEMENT_3D ( 'NONE', #10417, #13087, #2029 ) ;
#12850=CARTESIAN_POINT ( 'NONE',  ( 35.34529388524494209, 143.8751093726684758, -21.33821933965574402 ) ) ;
#12854=CARTESIAN_POINT ( 'NONE',  ( -75.00000000000000000, 196.6227766016838245, -35.00200000000000244 ) ) ;
#12855=DIRECTION ( 'NONE',  ( 1.000000000000000000, 0.000000000000000000, 0.000000000000000000 ) ) ;
#12858=VECTOR ( 'NONE', #16153, 1000.000000000000000 ) ;
#12860=CARTESIAN_POINT ( 'NONE',  ( -73.34456489498955989, 200.1146145092350821, -16.67123533649924383 ) ) ;
#12870=ORIENTED_EDGE ( 'NONE', *, *, #937, .T. ) ;
#12871=DIRECTION ( 'NONE',  ( 0.000000000000000000, 0.000000000000000000, 1.000000000000000000 ) ) ;
#12872=VECTOR ( 'NONE', #2903, 1000.000000000000000 ) ;
#12873=CARTESIAN_POINT ( 'NONE',  ( -19.79962810613638169, 20.00000000000000355, -20.97942696524415851 ) ) ;
#12876=AXIS2_PLACEMENT_3D ( 'NONE', #15461, #11302, #11206 ) ;
#12877=DIRECTION ( 'NONE',  ( -0.000000000000000000, -0.000000000000000000, 1.000000000000000000 ) ) ;
#12880=ORIENTED_EDGE ( 'NONE', *, *, #15485, .T. ) ;
#12882=PRESENTATION_STYLE_ASSIGNMENT (( #13883 ) ) ;
#12887=DIRECTION ( 'NONE',  ( -1.000000000000000000, -0.000000000000000000, 0.000000000000000000 ) ) ;
#12888=CIRCLE ( 'NONE', #6946, 2.499999999999998668 ) ;
#12889=EDGE_CURVE ( 'NONE', #14544, #5702, #6737, .T. ) ;
#12890=LINE ( 'NONE', #14144, #13157 ) ;
#12895=VERTEX_POINT ( 'NONE', #5412 ) ;
#12897=DIRECTION ( 'NONE',  ( 0.000000000000000000, 0.000000000000000000, 1.000000000000000000 ) ) ;
#12900=CARTESIAN_POINT ( 'NONE',  ( -16.58710929330769090, 31.97525413706907216, -10.34574908881256050 ) ) ;
#12911=CIRCLE ( 'NONE', #5280, 7.500000000000003553 ) ;
#12912=DIRECTION ( 'NONE',  ( -0.000000000000000000, -0.000000000000000000, 1.000000000000000000 ) ) ;
#12913=DIRECTION ( 'NONE',  ( 8.673617379884037937E-17, 0.000000000000000000, 1.000000000000000000 ) ) ;
#12915=ORIENTED_EDGE ( 'NONE', *, *, #14451, .F. ) ;
#12919=CARTESIAN_POINT ( 'NONE',  ( 32.41901710885975518, 202.1180966153993097, -17.17743398583138870 ) ) ;
#12923=CARTESIAN_POINT ( 'NONE',  ( 18.16394926501914497, 19.99999999999999645, -14.51477632729204537 ) ) ;
#12924=VECTOR ( 'NONE', #17431, 1000.000000000000000 ) ;
#12926=AXIS2_PLACEMENT_3D ( 'NONE', #9817, #4777, #3267 ) ;
#12927=ORIENTED_EDGE ( 'NONE', *, *, #3820, .T. ) ;
#12930=AXIS2_PLACEMENT_3D ( 'NONE', #3878, #14491, #6615 ) ;
#12931=DIRECTION ( 'NONE',  ( 0.000000000000000000, 0.000000000000000000, 1.000000000000000000 ) ) ;
#12932=ORIENTED_EDGE ( 'NONE', *, *, #11421, .T. ) ;
#12933=ADVANCED_FACE ( 'NONE', ( #1427 ), #4079, .T. ) ;
#12934=CARTESIAN_POINT ( 'NONE',  ( 36.42104199761076444, 200.5259344270105260, -15.94638436093397083 ) ) ;
#12938=VECTOR ( 'NONE', #9888, 1000.000000000000000 ) ;
#12942=CARTESIAN_POINT ( 'NONE',  ( 36.00000000000002132, 146.6227766016838245, -24.49489742783179125 ) ) ;
#12944=CARTESIAN_POINT ( 'NONE',  ( -70.00000000000000000, 154.3022685259950038, -9.999999999999900524 ) ) ;
#12945=ORIENTED_EDGE ( 'NONE', *, *, #17363, .F. ) ;
#12951=EDGE_CURVE ( 'NONE', #7374, #16329, #6138, .T. ) ;
#12954=EDGE_CURVE ( 'NONE', #15922, #4370, #17454, .T. ) ;
#12956=ORIENTED_EDGE ( 'NONE', *, *, #11712, .F. ) ;
#12957=DIRECTION ( 'NONE',  ( 1.000000000000000000, 0.000000000000000000, 0.000000000000000000 ) ) ;
#12959=CARTESIAN_POINT ( 'NONE',  ( -15.37994105483213758, 31.72997864396344525, -11.82123051499886479 ) ) ;
#12962=CARTESIAN_POINT ( 'NONE',  ( -95.00000000000000000, 201.6227766016838245, -1.836970198721029589E-15 ) ) ;
#12964=CYLINDRICAL_SURFACE ( 'NONE', #5686, 6.000000000000008882 ) ;
#12965=ORIENTED_EDGE ( 'NONE', *, *, #13939, .F. ) ;
#12967=AXIS2_PLACEMENT_3D ( 'NONE', #8208, #9618, #1400 ) ;
#12969=ORIENTED_EDGE ( 'NONE', *, *, #1129, .F. ) ;
#12970=VERTEX_POINT ( 'NONE', #8141 ) ;
#12974=ORIENTED_EDGE ( 'NONE', *, *, #11030, .T. ) ;
#12977=FACE_OUTER_BOUND ( 'NONE', #15603, .T. ) ;
#12979=LINE ( 'NONE', #10228, #10042 ) ;
#12983=EDGE_LOOP ( 'NONE', ( #2247, #3555 ) ) ;
#12984=DIRECTION ( 'NONE',  ( 1.000000000000000000, 0.000000000000000000, 0.000000000000000000 ) ) ;
#12985=DIRECTION ( 'NONE',  ( 1.000000000000000000, 0.000000000000000000, 0.000000000000000000 ) ) ;
#12987=CARTESIAN_POINT ( 'NONE',  ( -15.09561842307909707, 19.99999999999307931, -7.342182892333040556 ) ) ;
#12988=DIRECTION ( 'NONE',  ( 1.000000000000000000, 0.000000000000000000, 0.000000000000000000 ) ) ;
#12990=AXIS2_PLACEMENT_3D ( 'NONE', #979, #17018, #15945 ) ;
#12991=ADVANCED_FACE ( 'NONE', ( #1504 ), #8, .F. ) ;
#12993=CARTESIAN_POINT ( 'NONE',  ( -95.00000000000000000, 171.6227766016838245, -30.00000000000000000 ) ) ;
#12994=ORIENTED_EDGE ( 'NONE', *, *, #4717, .F. ) ;
#13000=EDGE_CURVE ( 'NONE', #1173, #2136, #10969, .T. ) ;
#13001=CIRCLE ( 'NONE', #13859, 2.500000000000000000 ) ;
#13002=LINE ( 'NONE', #4934, #15790 ) ;
#13013=EDGE_CURVE ( 'NONE', #8812, #6709, #4430, .T. ) ;
#13014=CARTESIAN_POINT ( 'NONE',  ( 29.53214135918837968, 19.99999999999999645, -18.68621337608103516 ) ) ;
#13016=CIRCLE ( 'NONE', #10189, 20.00000000000000355 ) ;
#13017=CARTESIAN_POINT ( 'NONE',  ( 11.58137902169779920, 142.1604892273610687, -18.89461017025931966 ) ) ;
#13018=ORIENTED_EDGE ( 'NONE', *, *, #16538, .F. ) ;
#13019=DIRECTION ( 'NONE',  ( 0.000000000000000000, 0.000000000000000000, 1.000000000000000000 ) ) ;
#13020=AXIS2_PLACEMENT_3D ( 'NONE', #3161, #8554, #4582 ) ;
#13021=DIRECTION ( 'NONE',  ( -0.000000000000000000, -0.000000000000000000, -1.000000000000000000 ) ) ;
#13024=CARTESIAN_POINT ( 'NONE',  ( -80.00000000000002842, 146.6227766016838245, -13.00000000000000000 ) ) ;
#13025=EDGE_CURVE ( 'NONE', #7898, #16968, #3023, .T. ) ;
#13028=CARTESIAN_POINT ( 'NONE',  ( 27.99999999999998224, 9.999999999999998224, -35.00000000000000000 ) ) ;
#13030=CARTESIAN_POINT ( 'NONE',  ( -50.00000000000000000, 143.0439382767972631, -16.49999999999984013 ) ) ;
#13032=CARTESIAN_POINT ( 'NONE',  ( 29.47106614592656015, 140.6403763931701576, -16.28177936134992621 ) ) ;
#13033=ORIENTED_EDGE ( 'NONE', *, *, #12376, .F. ) ;
#13035=EDGE_CURVE ( 'NONE', #9392, #11112, #4605, .T. ) ;
#13038=DIRECTION ( 'NONE',  ( 1.000000000000000000, 1.156482317317868274E-16, 0.000000000000000000 ) ) ;
#13042=VECTOR ( 'NONE', #8869, 1000.000000000000000 ) ;
#13044=EDGE_LOOP ( 'NONE', ( #16235, #10500 ) ) ;
#13047=CARTESIAN_POINT ( 'NONE',  ( 30.00000000000001066, 146.6227766016838245, -16.00000000000000000 ) ) ;
#13048=CARTESIAN_POINT ( 'NONE',  ( -25.16839285024616402, 18.00000000000000000, -15.12082343620105540 ) ) ;
#13049=EDGE_LOOP ( 'NONE', ( #16148, #17171, #14876, #17036 ) ) ;
#13050=FACE_OUTER_BOUND ( 'NONE', #15278, .T. ) ;
#13053=EDGE_CURVE ( 'NONE', #14777, #15022, #16736, .T. ) ;
#13054=EDGE_CURVE ( 'NONE', #9101, #3454, #14081, .T. ) ;
#13056=CARTESIAN_POINT ( 'NONE',  ( 28.43487082456423209, 190.8261496651128937, -29.26147795858665290 ) ) ;
#13057=CARTESIAN_POINT ( 'NONE',  ( -40.00000000000000711, 0.000000000000000000, 0.000000000000000000 ) ) ;
#13061=CARTESIAN_POINT ( 'NONE',  ( -85.45515645957152628, 151.7936747764227334, -26.38258506112510560 ) ) ;
#13062=ORIENTED_EDGE ( 'NONE', *, *, #12702, .F. ) ;
#13066=CARTESIAN_POINT ( 'NONE',  ( 24.85999067142302010, 149.7234947166294035, -27.30319596934541693 ) ) ;
#13067=CARTESIAN_POINT ( 'NONE',  ( 15.00000000000000000, 154.3022685259950038, -9.999999999999900524 ) ) ;
#13072=EDGE_CURVE ( 'NONE', #11521, #8796, #2178, .T. ) ;
#13073=EDGE_CURVE ( 'NONE', #16820, #9959, #12750, .T. ) ;
#13075=CARTESIAN_POINT ( 'NONE',  ( -18.25212770525392614, 32.30769230766699707, -5.660855707253096725 ) ) ;
#13077=DIRECTION ( 'NONE',  ( -0.000000000000000000, -0.000000000000000000, 1.000000000000000000 ) ) ;
#13081=VERTEX_POINT ( 'NONE', #4687 ) ;
#13082=( NAMED_UNIT ( * ) SI_UNIT ( $, .STERADIAN. ) SOLID_ANGLE_UNIT ( ) );
#13084=CARTESIAN_POINT ( 'NONE',  ( 15.97577464858015617, 18.00000000000228084, -12.97048270532338243 ) ) ;
#13085=CARTESIAN_POINT ( 'NONE',  ( -81.29609393525485928, 140.7594520581393738, -16.50672721711051238 ) ) ;
#13087=DIRECTION ( 'NONE',  ( 1.000000000000000000, 0.000000000000000000, -0.000000000000000000 ) ) ;
#13091=DIRECTION ( 'NONE',  ( 0.000000000000000000, 0.000000000000000000, 1.000000000000000000 ) ) ;
#13092=CARTESIAN_POINT ( 'NONE',  ( 28.24533480114369866, 202.3655582339692103, -16.73015311598867783 ) ) ;
#13094=VERTEX_POINT ( 'NONE', #1769 ) ;
#13095=CARTESIAN_POINT ( 'NONE',  ( 14.93242934743711814, 20.00000000000000355, -15.00000000000000000 ) ) ;
#13097=ORIENTED_EDGE ( 'NONE', *, *, #8936, .F. ) ;
#13098=CARTESIAN_POINT ( 'NONE',  ( -86.00000000000002842, 146.6227766016838245, -24.49489742783179480 ) ) ;
#13099=CARTESIAN_POINT ( 'NONE',  ( 14.92136712345229554, 126.5341449364669728, -7.654582290614115436 ) ) ;
#13100=EDGE_LOOP ( 'NONE', ( #11197, #11725, #14734, #11065 ) ) ;
#13102=FACE_OUTER_BOUND ( 'NONE', #2264, .T. ) ;
#13104=LINE ( 'NONE', #3728, #4144 ) ;
#13109=ORIENTED_EDGE ( 'NONE', *, *, #6577, .F. ) ;
#13112=ORIENTED_EDGE ( 'NONE', *, *, #1387, .F. ) ;
#13113=ADVANCED_FACE ( 'NONE', ( #11406 ), #4451, .F. ) ;
#13114=FACE_OUTER_BOUND ( 'NONE', #8055, .T. ) ;
#13116=CARTESIAN_POINT ( 'NONE',  ( -11.98734322101359240, 18.00000000000000355, -24.50584837321702736 ) ) ;
#13121=B_SPLINE_CURVE_WITH_KNOTS ( 'NONE', 3,
 ( #8750, #8566, #12644, #4675 ),
 .UNSPECIFIED., .F., .F.,
 ( 4, 4 ),
 ( 0.000000000000000000, 0.003888888888888887042 ),
 .UNSPECIFIED. ) ;
#13122=AXIS2_PLACEMENT_3D ( 'NONE', #15830, #11659, #17246 ) ;
#13125=DIRECTION ( 'NONE',  ( 1.000000000000000000, 0.000000000000000000, 0.000000000000000000 ) ) ;
#13127=DIRECTION ( 'NONE',  ( -0.01578383822436034076, 0.1110972697184772484, -0.9936841888205766304 ) ) ;
#13128=CARTESIAN_POINT ( 'NONE',  ( -14.55266450408069723, 18.00000000000000000, -23.76398220081675206 ) ) ;
#13130=CARTESIAN_POINT ( 'NONE',  ( -5.000000000000000888, 171.6227766016838245, 0.000000000000000000 ) ) ;
#13132=CARTESIAN_POINT ( 'NONE',  ( 27.00061905785951666, 191.4078883217828491, -28.87216486436160423 ) ) ;
#13135=AXIS2_PLACEMENT_3D ( 'NONE', #9841, #4710, #5864 ) ;
#13136=VERTEX_POINT ( 'NONE', #794 ) ;
#13138=CARTESIAN_POINT ( 'NONE',  ( -87.34664361473880945, 148.1846496461902518, -23.23759988234784046 ) ) ;
#13142=CARTESIAN_POINT ( 'NONE',  ( 27.99999999999998224, 9.999999999999998224, 0.000000000000000000 ) ) ;
#13145=CARTESIAN_POINT ( 'NONE',  ( 31.11555797696667369, 152.5224481282687066, -29.32884290898093838 ) ) ;
#13148=AXIS2_PLACEMENT_3D ( 'NONE', #1411, #12020, #16197 ) ;
#13150=DIRECTION ( 'NONE',  ( -0.000000000000000000, -0.000000000000000000, 1.000000000000000000 ) ) ;
#13151=CARTESIAN_POINT ( 'NONE',  ( 15.59275333247216366, 29.99107914678833353, -15.00000000000000000 ) ) ;
#13152=CARTESIAN_POINT ( 'NONE',  ( -20.85786437626906675, 124.1421356237309652, -14.99999999999998401 ) ) ;
#13153=CARTESIAN_POINT ( 'NONE',  ( 39.99999999999998579, 4.000000000000000000, -30.00000000000001066 ) ) ;
#13155=ORIENTED_EDGE ( 'NONE', *, *, #1162, .T. ) ;
#13157=VECTOR ( 'NONE', #4838, 1000.000000000000000 ) ;
#13158=CYLINDRICAL_SURFACE ( 'NONE', #286, 6.000000000000005329 ) ;
#13161=CARTESIAN_POINT ( 'NONE',  ( -80.00000000000002842, 146.6227766016838245, -16.00000000000000000 ) ) ;
#13164=AXIS2_PLACEMENT_3D ( 'NONE', #14663, #2627, #7744 ) ;
#13166=EDGE_CURVE ( 'NONE', #4295, #6662, #6184, .T. ) ;
#13169=ADVANCED_FACE ( 'NONE', ( #7164 ), #12561, .T. ) ;
#13170=CARTESIAN_POINT ( 'NONE',  ( 16.75727253400481942, 18.00000000000114397, -12.82782196133976704 ) ) ;
#13171=CARTESIAN_POINT ( 'NONE',  ( -84.98839123081494051, 143.2703805450037464, -20.52792728560773838 ) ) ;
#13177=AXIS2_PLACEMENT_3D ( 'NONE', #8811, #4828, #667 ) ;
#13182=ORIENTED_EDGE ( 'NONE', *, *, #1328, .T. ) ;
#13185=CARTESIAN_POINT ( 'NONE',  ( 12.95626684960129893, 129.1819364320672321, -10.30967895453046879 ) ) ;
#13187=CARTESIAN_POINT ( 'NONE',  ( 32.99999999999998579, 9.999999999999998224, 0.000000000000000000 ) ) ;
#13188=CIRCLE ( 'NONE', #9227, 2.500000000000002220 ) ;
#13189=FACE_OUTER_BOUND ( 'NONE', #4369, .T. ) ;
#13193=DIRECTION ( 'NONE',  ( 1.000000000000000000, 0.000000000000000000, -0.000000000000000000 ) ) ;
#13195=DIRECTION ( 'NONE',  ( 1.000000000000000000, 0.000000000000000000, 0.000000000000000000 ) ) ;
#13198=CARTESIAN_POINT ( 'NONE',  ( 33.48938398233770641, 141.7273756662291930, -18.20613184929474926 ) ) ;
#13199=CIRCLE ( 'NONE', #10356, 2.500000000000000000 ) ;
#13202=ORIENTED_EDGE ( 'NONE', *, *, #15006, .T. ) ;
#13204=CIRCLE ( 'NONE', #778, 27.69059892324149175 ) ;
#13207=VERTEX_POINT ( 'NONE', #12017 ) ;
#13214=AXIS2_PLACEMENT_3D ( 'NONE', #8119, #11041, #13531 ) ;
#13217=AXIS2_PLACEMENT_3D ( 'NONE', #4579, #1912, #5901 ) ;
#13219=CARTESIAN_POINT ( 'NONE',  ( -17.86279820300995169, 32.23061541110773476, -7.751589558536285729 ) ) ;
#13220=CARTESIAN_POINT ( 'NONE',  ( -27.30244652380281778, 18.00000000000000000, -10.27378278477019080 ) ) ;
#13222=FACE_OUTER_BOUND ( 'NONE', #4686, .T. ) ;
#13224=CARTESIAN_POINT ( 'NONE',  ( 30.46084342859877836, 190.6362156748385530, -29.38520182610346509 ) ) ;
#13227=VECTOR ( 'NONE', #11284, 1000.000000000000000 ) ;
#13228=ORIENTED_EDGE ( 'NONE', *, *, #8512, .T. ) ;
#13229=ORIENTED_EDGE ( 'NONE', *, *, #8514, .T. ) ;
#13232=CARTESIAN_POINT ( 'NONE',  ( -74.54894360611541515, 151.7804781109684029, -26.36917907415269013 ) ) ;
#13233=ADVANCED_FACE ( 'NONE', ( #6271 ), #2287, .T. ) ;
#13234=ORIENTED_EDGE ( 'NONE', *, *, #17266, .F. ) ;
#13238=DIRECTION ( 'NONE',  ( -0.000000000000000000, -0.000000000000000000, 1.000000000000000000 ) ) ;
#13240=CARTESIAN_POINT ( 'NONE',  ( 29.52501904231387897, 152.6213468612617419, -29.39295273708633971 ) ) ;
#13243=AXIS2_PLACEMENT_3D ( 'NONE', #10885, #5230, #1342 ) ;
#13250=CARTESIAN_POINT ( 'NONE',  ( -27.98221281341758626, 19.99999999999999645, -6.321711414556861364 ) ) ;
#13254=EDGE_CURVE ( 'NONE', #17478, #16965, #13514, .T. ) ;
#13256=ORIENTED_EDGE ( 'NONE', *, *, #680, .T. ) ;
#13259=FACE_OUTER_BOUND ( 'NONE', #7888, .T. ) ;
#13260=ORIENTED_EDGE ( 'NONE', *, *, #16099, .T. ) ;
#13262=CARTESIAN_POINT ( 'NONE',  ( 14.93242934743710570, 30.00000000000000000, -13.00000000000000178 ) ) ;
#13263=CARTESIAN_POINT ( 'NONE',  ( -78.94173059828752059, 140.7111270992951120, -16.41570701070895311 ) ) ;
#13265=VERTEX_POINT ( 'NONE', #6349 ) ;
#13266=DIRECTION ( 'NONE',  ( 0.000000000000000000, 0.000000000000000000, 1.000000000000000000 ) ) ;
#13272=EDGE_CURVE ( 'NONE', #7418, #4419, #954, .T. ) ;
#13277=CARTESIAN_POINT ( 'NONE',  ( 12.97014296496520736, 138.3438685529228565, -12.30864880703445152 ) ) ;
#13279=CARTESIAN_POINT ( 'NONE',  ( -82.81127788294642755, 151.9278302392748685, -28.93306197017449222 ) ) ;
#13280=CARTESIAN_POINT ( 'NONE',  ( 13.53786153804126435, 143.5554826938402755, -17.35616514752890183 ) ) ;
#13282=ORIENTED_EDGE ( 'NONE', *, *, #8795, .T. ) ;
#13284=CARTESIAN_POINT ( 'NONE',  ( 30.00000000000001066, 146.6227766016838245, -16.00000000000000000 ) ) ;
#13285=AXIS2_PLACEMENT_3D ( 'NONE', #13307, #8066, #11879 ) ;
#13289=CARTESIAN_POINT ( 'NONE',  ( 22.87887136921732889, 17.99999999999999645, -6.850254086360624939 ) ) ;
#13290=CARTESIAN_POINT ( 'NONE',  ( -725.0000000000000000, 19.99999999999995737, -4.999999999999999112 ) ) ;
#13291=FACE_OUTER_BOUND ( 'NONE', #2337, .T. ) ;
#13293=ORIENTED_EDGE ( 'NONE', *, *, #10540, .T. ) ;
#13294=DIRECTION ( 'NONE',  ( -1.000000000000000000, -6.938893903907228378E-16, -0.000000000000000000 ) ) ;
#13295=AXIS2_PLACEMENT_3D ( 'NONE', #5031, #14592, #15834 ) ;
#13296=DIRECTION ( 'NONE',  ( 1.000000000000000000, 0.000000000000000000, 0.000000000000000000 ) ) ;
#13300=AXIS2_PLACEMENT_3D ( 'NONE', #13284, #1327, #10526 ) ;
#13301=B_SPLINE_CURVE_WITH_KNOTS ( 'NONE', 3,
 ( #2459, #2556, #1133, #10508, #9091, #15913, #16190, #7948, #12014, #17417, #1217, #2284, #8025, #17148, #6712, #12112, #13263, #10592, #14497, #6538, #5197, #10416, #13353, #2640, #13085, #13436, #3704, #10691, #7757, #1307, #17516, #3979, #9362, #10781, #13171, #6622, #3781, #14767, #4060, #1041, #6441, #9437 ),
 .UNSPECIFIED., .F., .F.,
 ( 4, 2, 2, 2, 2, 2, 2, 2, 2, 2, 2, 2, 2, 2, 2, 2, 2, 2, 2, 2, 4 ),
 ( 0.000000000000000000, 0.003174452718035057977, 0.004761679077052617323, 0.006348905436070176669, 0.007936131795087736016, 0.009523358154105295362, 0.01031697133361409238, 0.01111058451312288940, 0.01190419769263168642, 0.01230100428238609968, 0.01269781087214051120, 0.01349142405164937761, 0.01428503723115824228, 0.01507865041066711043, 0.01587226359017597510, 0.01745948994919370445, 0.01904671630821143033, 0.02063394266722915621, 0.02222116902624688556, 0.02380839538526460797, 0.02539562174428233732 ),
 .UNSPECIFIED. ) ;
#13302=CARTESIAN_POINT ( 'NONE',  ( 48.00000000000000711, 167.6227766016838814, -21.92820660268601074 ) ) ;
#13307=CARTESIAN_POINT ( 'NONE',  ( 48.00000000000000711, 159.6227766016838814, -5.571800142134975431 ) ) ;
#13310=AXIS2_PLACEMENT_3D ( 'NONE', #3068, #16529, #8471 ) ;
#13314=CARTESIAN_POINT ( 'NONE',  ( -15.84134677353521070, 32.63429591450738343, -7.614689697697072823 ) ) ;
#13322=VERTEX_POINT ( 'NONE', #14327 ) ;
#13323=VERTEX_POINT ( 'NONE', #10513 ) ;
#13325=CARTESIAN_POINT ( 'NONE',  ( -73.91918570238915720, 151.0194919042433241, -25.77925661938085611 ) ) ;
#13326=ORIENTED_EDGE ( 'NONE', *, *, #11163, .T. ) ;
#13328=CARTESIAN_POINT ( 'NONE',  ( 27.48361012695488981, 138.6227766016838245, -1.225897272825924533 ) ) ;
#13329=CARTESIAN_POINT ( 'NONE',  ( -80.00000000000002842, 146.6227766016838245, -13.00000000000000000 ) ) ;
#13330=CARTESIAN_POINT ( 'NONE',  ( 34.82472073241385857, 150.2116474542520166, -27.68948087834226968 ) ) ;
#13331=AXIS2_PLACEMENT_3D ( 'NONE', #6944, #12259, #1197 ) ;
#13332=FACE_BOUND ( 'NONE', #5886, .T. ) ;
#13334=EDGE_CURVE ( 'NONE', #11751, #7408, #4187, .T. ) ;
#13336=CARTESIAN_POINT ( 'NONE',  ( -79.44857787935347915, 202.6030615872001022, -16.28580987144871628 ) ) ;
#13337=CARTESIAN_POINT ( 'NONE',  ( 16.24588547270996131, 29.98230316816100327, -14.93526533897157726 ) ) ;
#13339=DIRECTION ( 'NONE',  ( 0.000000000000000000, -1.000000000000000000, 8.673617379884035472E-17 ) ) ;
#13340=CARTESIAN_POINT ( 'NONE',  ( 37.50000000000000711, 196.6227766016838245, -21.54065922853802562 ) ) ;
#13342=CARTESIAN_POINT ( 'NONE',  ( -87.50000000000004263, 146.6227766016838245, -21.54065922853802562 ) ) ;
#13347=EDGE_LOOP ( 'NONE', ( #9327, #17414, #275, #14983, #7660, #12056 ) ) ;
#13348=FACE_BOUND ( 'NONE', #11020, .T. ) ;
#13350=ORIENTED_EDGE ( 'NONE', *, *, #17288, .F. ) ;
#13353=CARTESIAN_POINT ( 'NONE',  ( -80.52893385407348603, 140.6403763931701576, -16.28177936134992976 ) ) ;
#13360=ORIENTED_EDGE ( 'NONE', *, *, #7414, .T. ) ;
#13361=CARTESIAN_POINT ( 'NONE',  ( -50.00000000000000000, 206.6227766016838245, 2.143131898507868248E-15 ) ) ;
#13363=CARTESIAN_POINT ( 'NONE',  ( -82.99933485059881377, 151.8237148210350540, -28.86201951371925389 ) ) ;
#13364=CARTESIAN_POINT ( 'NONE',  ( 9.414336857517209722, 132.5946763488762770, -12.41924194405873649 ) ) ;
#13366=DIRECTION ( 'NONE',  ( -1.000000000000000000, 0.000000000000000000, 0.000000000000000000 ) ) ;
#13368=DIRECTION ( 'NONE',  ( 1.000000000000000000, 0.000000000000000000, 0.000000000000000000 ) ) ;
#13371=CARTESIAN_POINT ( 'NONE',  ( -725.0000000000000000, 19.99999999999995737, -4.999999999999997335 ) ) ;
#13372=CARTESIAN_POINT ( 'NONE',  ( 22.81311145407750374, 18.00000000000113687, -7.108351238697862229 ) ) ;
#13373=DIRECTION ( 'NONE',  ( 0.000000000000000000, 0.000000000000000000, 1.000000000000000000 ) ) ;
#13375=DIRECTION ( 'NONE',  ( -1.000000000000000000, -0.000000000000000000, 0.000000000000000000 ) ) ;
#13376=CARTESIAN_POINT ( 'NONE',  ( 24.65551710168432109, 143.8733932267928992, -21.33602313251873639 ) ) ;
#13381=CARTESIAN_POINT ( 'NONE',  ( -19.25702671965663626, 18.00000000000000355, -21.36300512502526061 ) ) ;
#13386=PLANE ( 'NONE',  #7906 ) ;
#13388=ADVANCED_FACE ( 'NONE', ( #4146 ), #5394, .F. ) ;
#13392=LINE ( 'NONE', #6666, #4978 ) ;
#13393=CARTESIAN_POINT ( 'NONE',  ( 35.08450508553749358, 191.0841166510128062, -26.65369102675423818 ) ) ;
#13396=CARTESIAN_POINT ( 'NONE',  ( -26.11264420168958722, 18.00000000000000000, -13.35921939055965524 ) ) ;
#13399=VERTEX_POINT ( 'NONE', #6972 ) ;
#13401=LINE ( 'NONE', #5352, #6113 ) ;
#13404=ORIENTED_EDGE ( 'NONE', *, *, #8034, .F. ) ;
#13405=VECTOR ( 'NONE', #3094, 1000.000000000000000 ) ;
#13408=ORIENTED_EDGE ( 'NONE', *, *, #2716, .T. ) ;
#13410=DIRECTION ( 'NONE',  ( 0.000000000000000000, 1.000000000000000000, 0.000000000000000000 ) ) ;
#13412=CARTESIAN_POINT ( 'NONE',  ( 24.27081732008962334, 148.4136790374692509, -26.19897850971621978 ) ) ;
#13417=CARTESIAN_POINT ( 'NONE',  ( -84.78531899738449340, 200.2598589880381894, -20.12830716182790880 ) ) ;
#13423=ORIENTED_EDGE ( 'NONE', *, *, #373, .T. ) ;
#13425=LINE ( 'NONE', #9938, #10046 ) ;
#13426=DIRECTION ( 'NONE',  ( 0.000000000000000000, -1.000000000000000000, 0.000000000000000000 ) ) ;
#13430=CARTESIAN_POINT ( 'NONE',  ( 196.0000000000000000, 175.6227766016838530, -19.42820660268601074 ) ) ;
#13432=ORIENTED_EDGE ( 'NONE', *, *, #460, .F. ) ;
#13434=VECTOR ( 'NONE', #8942, 1000.000000000000000 ) ;
#13436=CARTESIAN_POINT ( 'NONE',  ( -81.76357793902667481, 140.8827219813066165, -16.73516917262795189 ) ) ;
#13442=CARTESIAN_POINT ( 'NONE',  ( -80.00000000000002842, 146.6227766016838245, 1.387778780781445676E-14 ) ) ;
#13443=CARTESIAN_POINT ( 'NONE',  ( -40.00000000000000000, 4.000000000000000000, -30.00000000000000711 ) ) ;
#13444=FACE_OUTER_BOUND ( 'NONE', #2889, .T. ) ;
#13447=CARTESIAN_POINT ( 'NONE',  ( 12.82285603306638144, 130.8395207603766153, -12.92896204370639524 ) ) ;
#13448=ORIENTED_EDGE ( 'NONE', *, *, #13272, .F. ) ;
#13449=CARTESIAN_POINT ( 'NONE',  ( -79.10703801256936174, 152.5603119736738051, -29.35342143133167170 ) ) ;
#13450=CARTESIAN_POINT ( 'NONE',  ( 11.58137902169841027, 143.8440485058968363, -17.81491816053495825 ) ) ;
#13451=ORIENTED_EDGE ( 'NONE', *, *, #4038, .T. ) ;
#13452=CARTESIAN_POINT ( 'NONE',  ( -27.98221281347037959, 19.99999999999999645, 0.000000000000000000 ) ) ;
#13458=CYLINDRICAL_SURFACE ( 'NONE', #16319, 2.499999999999998668 ) ;
#13459=ADVANCED_FACE ( 'NONE', ( #4235 ), #8693, .T. ) ;
#13461=CARTESIAN_POINT ( 'NONE',  ( 27.13959012325753406, 18.00000000000000000, -20.89788123228700556 ) ) ;
#13466=VERTEX_POINT ( 'NONE', #2982 ) ;
#13467=CARTESIAN_POINT ( 'NONE',  ( 10.11940563665161541, 132.7319563576625399, -14.29042643364863885 ) ) ;
#13470=CIRCLE ( 'NONE', #183, 5.000000000000004441 ) ;
#13471=CARTESIAN_POINT ( 'NONE',  ( -19.79962810613639945, 18.00000000000000711, -20.97942696524416206 ) ) ;
#13472=EDGE_CURVE ( 'NONE', #17412, #160, #7000, .T. ) ;
#13479=ORIENTED_EDGE ( 'NONE', *, *, #3118, .F. ) ;
#13480=LINE ( 'NONE', #9314, #15451 ) ;
#13483=CARTESIAN_POINT ( 'NONE',  ( 34.24679270737827608, 190.4349707265700715, -27.11332964807921897 ) ) ;
#13490=CARTESIAN_POINT ( 'NONE',  ( -5.000000000000000888, 204.6227766016838245, 2.020667218593133100E-15 ) ) ;
#13491=ORIENTED_EDGE ( 'NONE', *, *, #1057, .F. ) ;
#13492=CARTESIAN_POINT ( 'NONE',  ( -86.80614408739177179, 193.4380998888853185, -24.76648413410753946 ) ) ;
#13497=ORIENTED_EDGE ( 'NONE', *, *, #5737, .T. ) ;
#13498=EDGE_CURVE ( 'NONE', #10197, #16285, #15370, .T. ) ;
#13499=EDGE_LOOP ( 'NONE', ( #7073, #6681, #4905, #13956 ) ) ;
#13503=MECHANICAL_DESIGN_GEOMETRIC_PRESENTATION_REPRESENTATION('',(#1347),#9241);
#13505=SHAPE_DEFINITION_REPRESENTATION ( #7152, #7924 ) ;
#13508=CARTESIAN_POINT ( 'NONE',  ( 19.16569565073602277, 29.91542719746881929, -11.79421528189872070 ) ) ;
#13512=ORIENTED_EDGE ( 'NONE', *, *, #8022, .F. ) ;
#13513=CARTESIAN_POINT ( 'NONE',  ( -85.49405842113658593, 199.0592542586747982, -21.73717956246137106 ) ) ;
#13514=CIRCLE ( 'NONE', #211, 2.500000000000000000 ) ;
#13516=LINE ( 'NONE', #10578, #5810 ) ;
#13520=CARTESIAN_POINT ( 'NONE',  ( 35.00000000000000711, 146.6227766016838245, 0.000000000000000000 ) ) ;
#13521=VERTEX_POINT ( 'NONE', #8821 ) ;
#13523=ORIENTED_EDGE ( 'NONE', *, *, #13472, .F. ) ;
#13525=DIRECTION ( 'NONE',  ( 1.000000000000000000, 0.000000000000000000, 0.000000000000000000 ) ) ;
#13528=DIRECTION ( 'NONE',  ( -1.000000000000000000, 0.000000000000000000, 0.000000000000000000 ) ) ;
#13531=DIRECTION ( 'NONE',  ( 0.000000000000000000, 0.000000000000000000, -1.000000000000000000 ) ) ;
#13533=FACE_OUTER_BOUND ( 'NONE', #12261, .T. ) ;
#13535=CARTESIAN_POINT ( 'NONE',  ( -100.0000000000000000, 171.6227766016838245, 0.000000000000000000 ) ) ;
#13538=CARTESIAN_POINT ( 'NONE',  ( 21.38051303314620810, 139.8000659834381736, -14.57605648433057510 ) ) ;
#13544=FACE_OUTER_BOUND ( 'NONE', #7332, .T. ) ;
#13545=CYLINDRICAL_SURFACE ( 'NONE', #1371, 20.00000000000000355 ) ;
#13552=CARTESIAN_POINT ( 'NONE',  ( 33.66001102075319551, 18.00000000000000000, -12.05479157725487482 ) ) ;
#13557=CARTESIAN_POINT ( 'NONE',  ( 49.99999999999998579, 179.6227766016838245, -15.00000337241049486 ) ) ;
#13558=ORIENTED_EDGE ( 'NONE', *, *, #7811, .F. ) ;
#13559=CARTESIAN_POINT ( 'NONE',  ( 13.34250444320487361, 130.4016344817123070, -12.56142338728217744 ) ) ;
#13569=VECTOR ( 'NONE', #3699, 1000.000000000000000 ) ;
#13570=EDGE_CURVE ( 'NONE', #14296, #243, #16632, .T. ) ;
#13571=CYLINDRICAL_SURFACE ( 'NONE', #13590, 12.00000000000000000 ) ;
#13572=EDGE_LOOP ( 'NONE', ( #797, #11071, #7276, #14509 ) ) ;
#13575=DIRECTION ( 'NONE',  ( 0.000000000000000000, 0.000000000000000000, 1.000000000000000000 ) ) ;
#13576=CARTESIAN_POINT ( 'NONE',  ( 15.60228996708978855, 124.9392590763941371, -1.671781470417840199 ) ) ;
#13577=CIRCLE ( 'NONE', #3400, 27.69059892324149175 ) ;
#13579=CYLINDRICAL_SURFACE ( 'NONE', #10787, 2.500000000000000444 ) ;
#13585=DIRECTION ( 'NONE',  ( 0.000000000000000000, 1.000000000000000000, 0.000000000000000000 ) ) ;
#13588=EDGE_LOOP ( 'NONE', ( #15792, #9415, #14085, #7427, #6683, #6613, #4136, #15497 ) ) ;
#13590=AXIS2_PLACEMENT_3D ( 'NONE', #9565, #14972, #15233 ) ;
#13593=CIRCLE ( 'NONE', #15847, 2.500000000000002220 ) ;
#13594=ORIENTED_EDGE ( 'NONE', *, *, #14950, .F. ) ;
#13597=DIRECTION ( 'NONE',  ( -0.000000000000000000, -0.000000000000000000, 1.000000000000000000 ) ) ;
#13598=CARTESIAN_POINT ( 'NONE',  ( 18.93858299686282365, 29.91990340250987757, -11.93041869825017898 ) ) ;
#13604=ORIENTED_EDGE ( 'NONE', *, *, #14950, .T. ) ;
#13607=CARTESIAN_POINT ( 'NONE',  ( 15.00000000000000000, 143.1210915093834330, -16.64102305613075572 ) ) ;
#13609=DIRECTION ( 'NONE',  ( 0.000000000000000000, 0.000000000000000000, 1.000000000000000000 ) ) ;
#13610=CARTESIAN_POINT ( 'NONE',  ( 49.99999999999998579, 163.6227766016838530, -10.00000337241049309 ) ) ;
#13612=CARTESIAN_POINT ( 'NONE',  ( -100.0000000000000000, 171.6227766016838245, 0.000000000000000000 ) ) ;
#13613=ORIENTED_EDGE ( 'NONE', *, *, #13863, .T. ) ;
#13617=( NAMED_UNIT ( * ) PLANE_ANGLE_UNIT ( ) SI_UNIT ( $, .RADIAN. ) );
#13618=CARTESIAN_POINT ( 'NONE',  ( 17.58250999373982282, 125.2198453306090045, -5.979920648958140776E-13 ) ) ;
#13620=CARTESIAN_POINT ( 'NONE',  ( 27.99999999999998224, 9.999999999999998224, -16.00000000000000000 ) ) ;
#13621=EDGE_CURVE ( 'NONE', #15447, #7515, #1921, .T. ) ;
#13623=EDGE_CURVE ( 'NONE', #6848, #1517, #16336, .T. ) ;
#13624=ORIENTED_EDGE ( 'NONE', *, *, #4524, .T. ) ;
#13625=DIRECTION ( 'NONE',  ( 0.000000000000000000, 0.000000000000000000, 1.000000000000000000 ) ) ;
#13626=DIRECTION ( 'NONE',  ( 0.000000000000000000, 0.000000000000000000, -1.000000000000000000 ) ) ;
#13631=CARTESIAN_POINT ( 'NONE',  ( -74.00000000000002842, 146.6227766016838245, -24.49489742783179125 ) ) ;
#13634=CARTESIAN_POINT ( 'NONE',  ( -45.00000000000000000, 120.0000000000000142, 0.000000000000000000 ) ) ;
#13635=EDGE_CURVE ( 'NONE', #1799, #16973, #11908, .T. ) ;
#13636=DIRECTION ( 'NONE',  ( -1.000000000000000000, -0.000000000000000000, 0.000000000000000000 ) ) ;
#13638=FACE_OUTER_BOUND ( 'NONE', #14093, .T. ) ;
#13639=DIRECTION ( 'NONE',  ( 1.000000000000000000, 0.000000000000000000, -0.000000000000000000 ) ) ;
#13641=CARTESIAN_POINT ( 'NONE',  ( 15.00000000000903455, 143.2885527162398489, -16.91661185963483760 ) ) ;
#13642=EDGE_LOOP ( 'NONE', ( #6130, #16908 ) ) ;
#13643=CARTESIAN_POINT ( 'NONE',  ( -25.81900932159183526, 19.99999999999999645, -13.95463872937544991 ) ) ;
#13649=CARTESIAN_POINT ( 'NONE',  ( -74.00000000000002842, 146.6227766016838245, -16.00000000000000000 ) ) ;
#13652=CARTESIAN_POINT ( 'NONE',  ( 23.19504936680528573, 149.8103701614163015, -24.76910924193868979 ) ) ;
#13653=ADVANCED_FACE ( 'NONE', ( #17314 ), #6327, .T. ) ;
#13655=CARTESIAN_POINT ( 'NONE',  ( -21.99999999999998579, 10.00000000000000000, -30.00000000000000355 ) ) ;
#13656=PLANE ( 'NONE',  #5791 ) ;
#13657=CARTESIAN_POINT ( 'NONE',  ( -27.99999999999998224, 10.00000000000000000, -16.00000000000000000 ) ) ;
#13665=ORIENTED_EDGE ( 'NONE', *, *, #12360, .T. ) ;
#13668=ORIENTED_EDGE ( 'NONE', *, *, #7974, .T. ) ;
#13669=VERTEX_POINT ( 'NONE', #14660 ) ;
#13672=LINE ( 'NONE', #14741, #10681 ) ;
#13673=ORIENTED_EDGE ( 'NONE', *, *, #11223, .F. ) ;
#13676=DIRECTION ( 'NONE',  ( 1.000000000000000000, 0.000000000000000000, 0.000000000000000000 ) ) ;
#13680=ORIENTED_EDGE ( 'NONE', *, *, #9737, .F. ) ;
#13681=CARTESIAN_POINT ( 'NONE',  ( -77.38716036884935079, 202.0279528788175583, -17.33673759440342010 ) ) ;
#13685=CARTESIAN_POINT ( 'NONE',  ( -34.99999999999999289, 122.0000000000000284, -4.999999999999999112 ) ) ;
#13696=CARTESIAN_POINT ( 'NONE',  ( -27.98221281347037603, 18.00000000000000000, 0.000000000000000000 ) ) ;
#13697=AXIS2_PLACEMENT_3D ( 'NONE', #3969, #14020, #9671 ) ;
#13698=EDGE_LOOP ( 'NONE', ( #15969, #434, #5708, #269 ) ) ;
#13703=AXIS2_PLACEMENT_3D ( 'NONE', #17449, #5673, #13722 ) ;
#13704=CARTESIAN_POINT ( 'NONE',  ( 23.14977753070778377, 139.1449216839932319, -13.05325656350955654 ) ) ;
#13710=CARTESIAN_POINT ( 'NONE',  ( -75.69074982301630428, 150.8166157800934002, -28.14689102807276200 ) ) ;
#13711=CARTESIAN_POINT ( 'NONE',  ( 15.22098041563561388, 126.0279773824920824, -6.884464680362713196 ) ) ;
#13712=ORIENTED_EDGE ( 'NONE', *, *, #16168, .F. ) ;
#13713=CARTESIAN_POINT ( 'NONE',  ( -79.53915657140119322, 190.6362156748385530, -29.38520182610347575 ) ) ;
#13714=DIRECTION ( 'NONE',  ( 1.000000000000000000, 0.000000000000000000, -0.000000000000000000 ) ) ;
#13718=CIRCLE ( 'NONE', #15976, 7.500000000000000000 ) ;
#13719=DIRECTION ( 'NONE',  ( 0.000000000000000000, 0.000000000000000000, -1.000000000000000000 ) ) ;
#13720=CARTESIAN_POINT ( 'NONE',  ( -15.00000000000001421, 20.00000000000004263, -4.999999999999999112 ) ) ;
#13721=AXIS2_PLACEMENT_3D ( 'NONE', #13535, #10600, #6447 ) ;
#13722=DIRECTION ( 'NONE',  ( 1.000000000000000000, 0.000000000000000000, 0.000000000000000000 ) ) ;
#13723=AXIS2_PLACEMENT_3D ( 'NONE', #12226, #97, #1248 ) ;
#13726=CARTESIAN_POINT ( 'NONE',  ( -10.00647404944701258, 19.99999999999999645, -14.03129316391565951 ) ) ;
#13730=EDGE_LOOP ( 'NONE', ( #14675, #10133, #17158, #5082, #15403 ) ) ;
#13732=DIRECTION ( 'NONE',  ( 0.000000000000000000, 0.000000000000000000, 1.000000000000000000 ) ) ;
#13736=CARTESIAN_POINT ( 'NONE',  ( 30.59986690501726514, 154.1043103600818540, -27.96613953460096269 ) ) ;
#13737=AXIS2_PLACEMENT_3D ( 'NONE', #2043, #3194, #10261 ) ;
#13739=CARTESIAN_POINT ( 'NONE',  ( 0.000000000000000000, 2.000000000000000000, 0.000000000000000000 ) ) ;
#13741=LINE ( 'NONE', #12416, #6260 ) ;
#13742=ORIENTED_EDGE ( 'NONE', *, *, #741, .T. ) ;
#13743=CARTESIAN_POINT ( 'NONE',  ( -27.99999999999998224, 10.00000000000000000, -35.00200000000000244 ) ) ;
#13747=ORIENTED_EDGE ( 'NONE', *, *, #1129, .T. ) ;
#13748=CARTESIAN_POINT ( 'NONE',  ( 18.97648483518030815, 140.5725221174451747, -16.15500418213391143 ) ) ;
#13749=EDGE_CURVE ( 'NONE', #12276, #4284, #17500, .T. ) ;
#13755=CARTESIAN_POINT ( 'NONE',  ( -10.05738114656989346, 30.87167111307020306, -12.65386873594253103 ) ) ;
#13761=EDGE_CURVE ( 'NONE', #8849, #2293, #1, .T. ) ;
#13769=CIRCLE ( 'NONE', #9518, 5.999999999999998224 ) ;
#13770=CARTESIAN_POINT ( 'NONE',  ( 14.93242934743710393, 30.00000000000000000, -13.00000000000000178 ) ) ;
#13776=CARTESIAN_POINT ( 'NONE',  ( 17.55923266082603007, 19.99999999999999645, -24.87049340120105612 ) ) ;
#13779=CARTESIAN_POINT ( 'NONE',  ( 40.00000000000000711, 136.6227766016838245, 0.000000000000000000 ) ) ;
#13785=EDGE_CURVE ( 'NONE', #9691, #10464, #3146, .T. ) ;
#13786=DIRECTION ( 'NONE',  ( 0.000000000000000000, -0.8660254037844413721, -0.4999999999999953371 ) ) ;
#13790=EDGE_CURVE ( 'NONE', #5589, #1310, #14932, .T. ) ;
#13795=DIRECTION ( 'NONE',  ( 0.000000000000000000, 0.000000000000000000, -1.000000000000000000 ) ) ;
#13796=CARTESIAN_POINT ( 'NONE',  ( -27.98221281347037959, 20.00000000000000000, -4.999999999999999112 ) ) ;
#13797=AXIS2_PLACEMENT_3D ( 'NONE', #5470, #13625, #16370 ) ;
#13800=EDGE_LOOP ( 'NONE', ( #4532, #16705 ) ) ;
#13802=CARTESIAN_POINT ( 'NONE',  ( 48.00000000000000711, 151.6227766016839098, -3.071800142134974099 ) ) ;
#13803=EDGE_CURVE ( 'NONE', #4701, #13081, #11528, .T. ) ;
#13804=LINE ( 'NONE', #8743, #16136 ) ;
#13805=CARTESIAN_POINT ( 'NONE',  ( -95.00000000000000000, 143.9321776784423150, 5.086680500673126297E-15 ) ) ;
#13806=CARTESIAN_POINT ( 'NONE',  ( 16.97810798871989135, 126.5456571586929044, -7.842726245482330327 ) ) ;
#13809=DIRECTION ( 'NONE',  ( 1.000000000000000000, 0.000000000000000000, -0.000000000000000000 ) ) ;
#13812=CARTESIAN_POINT ( 'NONE',  ( 14.16484689353800697, 138.6662281288708982, -3.797024489650347334 ) ) ;
#13814=CARTESIAN_POINT ( 'NONE',  ( -74.00000000000001421, 196.6227766016838245, -24.49489742783179125 ) ) ;
#13816=DIRECTION ( 'NONE',  ( 0.000000000000000000, 0.000000000000000000, 1.000000000000000000 ) ) ;
#13821=EDGE_CURVE ( 'NONE', #2935, #539, #12791, .T. ) ;
#13822=AXIS2_PLACEMENT_3D ( 'NONE', #15416, #4630, #8601 ) ;
#13825=AXIS2_PLACEMENT_3D ( 'NONE', #13620, #8376, #4319 ) ;
#13827=ORIENTED_EDGE ( 'NONE', *, *, #12324, .T. ) ;
#13836=AXIS2_PLACEMENT_3D ( 'NONE', #1389, #13609, #4220 ) ;
#13837=CARTESIAN_POINT ( 'NONE',  ( 37.50000000000000711, 196.6227766016838245, -21.54065922853802562 ) ) ;
#13838=VECTOR ( 'NONE', #3956, 1000.000000000000000 ) ;
#13841=DIRECTION ( 'NONE',  ( -1.000000000000000000, -0.000000000000000000, -0.000000000000000000 ) ) ;
#13846=ORIENTED_EDGE ( 'NONE', *, *, #1296, .T. ) ;
#13847=FACE_BOUND ( 'NONE', #11323, .T. ) ;
#13850=ORIENTED_EDGE ( 'NONE', *, *, #6319, .F. ) ;
#13852=AXIS2_PLACEMENT_3D ( 'NONE', #7611, #16752, #896 ) ;
#13855=ORIENTED_EDGE ( 'NONE', *, *, #12360, .F. ) ;
#13856=DIRECTION ( 'NONE',  ( -0.000000000000000000, -0.000000000000000000, -1.000000000000000000 ) ) ;
#13859=AXIS2_PLACEMENT_3D ( 'NONE', #4179, #2927, #13732 ) ;
#13860=VECTOR ( 'NONE', #14790, 1000.000000000000000 ) ;
#13862=LINE ( 'NONE', #571, #5402 ) ;
#13863=EDGE_CURVE ( 'NONE', #1718, #6730, #3389, .T. ) ;
#13869=LINE ( 'NONE', #4384, #15379 ) ;
#13874=CARTESIAN_POINT ( 'NONE',  ( 48.00000000000000711, 167.6227766016838814, -19.42820660268601074 ) ) ;
#13875=DIRECTION ( 'NONE',  ( -0.000000000000000000, -0.000000000000000000, 1.000000000000000000 ) ) ;
#13876=AXIS2_PLACEMENT_3D ( 'NONE', #16450, #16183, #6799 ) ;
#13878=ORIENTED_EDGE ( 'NONE', *, *, #1296, .F. ) ;
#13879=EDGE_LOOP ( 'NONE', ( #16791, #2374 ) ) ;
#13883=SURFACE_STYLE_USAGE ( .BOTH. , #11382 ) ;
#13885=DIRECTION ( 'NONE',  ( 0.000000000000000000, 0.000000000000000000, 1.000000000000000000 ) ) ;
#13886=EDGE_CURVE ( 'NONE', #2002, #12276, #16065, .T. ) ;
#13890=DIRECTION ( 'NONE',  ( 1.000000000000000000, 0.000000000000000000, 0.000000000000000000 ) ) ;
#13891=CARTESIAN_POINT ( 'NONE',  ( 33.88365274872860766, 18.00000000000000000, -11.43011099234507277 ) ) ;
#13892=EDGE_LOOP ( 'NONE', ( #2120, #825, #9104, #8454 ) ) ;
#13894=DIRECTION ( 'NONE',  ( -1.000000000000000000, -0.000000000000000000, -0.000000000000000000 ) ) ;
#13902=CARTESIAN_POINT ( 'NONE',  ( 49.99999999999998579, 151.6227766016839098, -5.571800142134973655 ) ) ;
#13903=VERTEX_POINT ( 'NONE', #8966 ) ;
#13904=CARTESIAN_POINT ( 'NONE',  ( -78.86396916296997972, 190.7269353522202664, -29.32635129980144839 ) ) ;
#13909=FACE_OUTER_BOUND ( 'NONE', #13588, .T. ) ;
#13911=FACE_BOUND ( 'NONE', #332, .T. ) ;
#13915=CARTESIAN_POINT ( 'NONE',  ( 49.99999999999998579, 175.6227766016838530, -21.92820660268601074 ) ) ;
#13916=ORIENTED_EDGE ( 'NONE', *, *, #3678, .T. ) ;
#13920=ADVANCED_FACE ( 'NONE', ( #6231 ), #17200, .F. ) ;
#13921=FACE_OUTER_BOUND ( 'NONE', #7601, .T. ) ;
#13927=DIRECTION ( 'NONE',  ( -0.000000000000000000, -0.000000000000000000, 1.000000000000000000 ) ) ;
#13929=CARTESIAN_POINT ( 'NONE',  ( 21.93446201513734550, 139.6105936900751203, -14.17700481206107455 ) ) ;
#13932=CARTESIAN_POINT ( 'NONE',  ( -13.22984127103138796, 31.85746429949665881, -11.06592603413638898 ) ) ;
#13933=EDGE_LOOP ( 'NONE', ( #147, #4823, #3495 ) ) ;
#13935=DIRECTION ( 'NONE',  ( -1.000000000000000000, -0.000000000000000000, -0.000000000000000000 ) ) ;
#13936=EDGE_CURVE ( 'NONE', #1055, #7056, #16640, .T. ) ;
#13938=CARTESIAN_POINT ( 'NONE',  ( -45.00000000000000000, 134.2062027339443944, -15.00000000000000000 ) ) ;
#13939=EDGE_CURVE ( 'NONE', #14899, #15553, #17482, .T. ) ;
#13944=DIRECTION ( 'NONE',  ( 1.000000000000000000, 0.000000000000000000, -0.000000000000000000 ) ) ;
#13946=DIRECTION ( 'NONE',  ( -1.000000000000000000, -0.000000000000000000, 0.000000000000000000 ) ) ;
#13948=DIRECTION ( 'NONE',  ( 0.000000000000000000, 0.000000000000000000, 1.000000000000000000 ) ) ;
#13949=ORIENTED_EDGE ( 'NONE', *, *, #14249, .F. ) ;
#13953=CARTESIAN_POINT ( 'NONE',  ( 30.00000000000001066, 146.6227766016838245, -16.00000000000000000 ) ) ;
#13954=DIRECTION ( 'NONE',  ( 1.000000000000000000, 0.000000000000000000, -0.000000000000000000 ) ) ;
#13955=EDGE_LOOP ( 'NONE', ( #5207, #8074 ) ) ;
#13956=ORIENTED_EDGE ( 'NONE', *, *, #9532, .F. ) ;
#13957=EDGE_CURVE ( 'NONE', #12804, #11894, #3669, .T. ) ;
#13961=DIRECTION ( 'NONE',  ( -0.000000000000000000, -0.000000000000000000, -1.000000000000000000 ) ) ;
#13962=VERTEX_POINT ( 'NONE', #15879 ) ;
#13967=CARTESIAN_POINT ( 'NONE',  ( 36.41998248565997187, 142.7179894756440035, -15.94334347237690430 ) ) ;
#13968=ORIENTED_EDGE ( 'NONE', *, *, #3935, .F. ) ;
#13970=LINE ( 'NONE', #2817, #8754 ) ;
#13971=CYLINDRICAL_SURFACE ( 'NONE', #16976, 5.000000000000004441 ) ;
#13974=EDGE_CURVE ( 'NONE', #14597, #3017, #7815, .T. ) ;
#13975=DIRECTION ( 'NONE',  ( 0.000000000000000000, 0.000000000000000000, 1.000000000000000000 ) ) ;
#13976=ORIENTED_EDGE ( 'NONE', *, *, #1965, .F. ) ;
#13979=ORIENTED_EDGE ( 'NONE', *, *, #9700, .T. ) ;
#13983=ADVANCED_FACE ( 'NONE', ( #13222 ), #10213, .T. ) ;
#13987=DIRECTION ( 'NONE',  ( 0.000000000000000000, 0.000000000000000000, 1.000000000000000000 ) ) ;
#13999=CARTESIAN_POINT ( 'NONE',  ( 32.99999999999998579, 9.999999999999998224, -12.99999999999999822 ) ) ;
#14000=EDGE_LOOP ( 'NONE', ( #14174, #8339, #12818, #4648 ) ) ;
#14001=APPLICATION_CONTEXT ( 'automotive_design' ) ;
#14004=AXIS2_PLACEMENT_3D ( 'NONE', #8778, #16925, #15329 ) ;
#14005=CARTESIAN_POINT ( 'NONE',  ( 30.00000000000001066, 146.6227766016838245, 1.387778780781445676E-14 ) ) ;
#14009=DIRECTION ( 'NONE',  ( -0.000000000000000000, -0.000000000000000000, -1.000000000000000000 ) ) ;
#14010=CARTESIAN_POINT ( 'NONE',  ( -73.34636706823184227, 143.1278587772776518, -16.66575456205189454 ) ) ;
#14011=EDGE_LOOP ( 'NONE', ( #6356, #8390, #9975, #9643 ) ) ;
#14012=CARTESIAN_POINT ( 'NONE',  ( 25.83188736168996513, 137.9746650487458908, -9.688332914129558660 ) ) ;
#14018=CIRCLE ( 'NONE', #10045, 7.500000000000020428 ) ;
#14019=ORIENTED_EDGE ( 'NONE', *, *, #4139, .F. ) ;
#14020=DIRECTION ( 'NONE',  ( -1.000000000000000000, -0.000000000000000000, -0.000000000000000000 ) ) ;
#14028=CARTESIAN_POINT ( 'NONE',  ( -100.0000000000000000, 171.6227766016838245, 0.000000000000000000 ) ) ;
#14030=AXIS2_PLACEMENT_3D ( 'NONE', #8445, #6689, #1467 ) ;
#14035=CARTESIAN_POINT ( 'NONE',  ( -7.965954974912850872, 30.19485118722929329, -13.00000000000000178 ) ) ;
#14038=CARTESIAN_POINT ( 'NONE',  ( 48.00000000000000711, 183.6227766016837961, -5.571800142134975431 ) ) ;
#14040=ADVANCED_FACE ( 'NONE', ( #7639 ), #750, .T. ) ;
#14042=EDGE_CURVE ( 'NONE', #5702, #10995, #12107, .T. ) ;
#14043=ORIENTED_EDGE ( 'NONE', *, *, #4142, .F. ) ;
#14044=DIRECTION ( 'NONE',  ( 1.000000000000000000, 0.000000000000000000, -0.000000000000000000 ) ) ;
#14045=CARTESIAN_POINT ( 'NONE',  ( 49.99999999999998579, 175.6227766016838245, -5.571800142134975431 ) ) ;
#14053=CARTESIAN_POINT ( 'NONE',  ( -725.0000000000000000, 19.99999999999995737, 0.000000000000000000 ) ) ;
#14056=DIRECTION ( 'NONE',  ( -1.156482317317868274E-16, 1.000000000000000000, 0.000000000000000000 ) ) ;
#14058=DIRECTION ( 'NONE',  ( 0.000000000000000000, 0.000000000000000000, 1.000000000000000000 ) ) ;
#14060=VERTEX_POINT ( 'NONE', #12962 ) ;
#14069=ORIENTED_EDGE ( 'NONE', *, *, #458, .T. ) ;
#14070=DIRECTION ( 'NONE',  ( 0.000000000000000000, -1.000000000000000000, -6.123233995736762338E-17 ) ) ;
#14071=ORIENTED_EDGE ( 'NONE', *, *, #12549, .F. ) ;
#14074=CARTESIAN_POINT ( 'NONE',  ( 49.99999999999998579, 183.6227766016837961, -3.071800142134975431 ) ) ;
#14077=LINE ( 'NONE', #3358, #6178 ) ;
#14078=ADVANCED_FACE ( 'NONE', ( #13050 ), #838, .T. ) ;
#14081=LINE ( 'NONE', #1851, #8114 ) ;
#14082=FACE_OUTER_BOUND ( 'NONE', #9066, .T. ) ;
#14084=DIRECTION ( 'NONE',  ( 1.000000000000000000, 0.000000000000000000, -0.000000000000000000 ) ) ;
#14085=ORIENTED_EDGE ( 'NONE', *, *, #11030, .F. ) ;
#14087=CARTESIAN_POINT ( 'NONE',  ( 23.71167364621568652, 19.99999999999772982, -10.06760101871518032 ) ) ;
#14089=CARTESIAN_POINT ( 'NONE',  ( 18.93231600135347392, 142.3609111598534298, -15.26062816855829851 ) ) ;
#14090=ORIENTED_EDGE ( 'NONE', *, *, #496, .F. ) ;
#14091=CARTESIAN_POINT ( 'NONE',  ( 30.00000000000000355, 196.6227766016838245, 0.000000000000000000 ) ) ;
#14093=EDGE_LOOP ( 'NONE', ( #5986, #13260, #16902, #7609 ) ) ;
#14094=FACE_OUTER_BOUND ( 'NONE', #10032, .T. ) ;
#14098=EDGE_CURVE ( 'NONE', #3793, #12895, #4824, .T. ) ;
#14103=CARTESIAN_POINT ( 'NONE',  ( -72.50000000000001421, 146.0561595177563845, -20.88304578468306261 ) ) ;
#14104=VERTEX_POINT ( 'NONE', #2154 ) ;
#14105=CARTESIAN_POINT ( 'NONE',  ( 17.37251483187831624, 141.0177972567464906, -16.98271123612915545 ) ) ;
#14107=ORIENTED_EDGE ( 'NONE', *, *, #281, .F. ) ;
#14111=CARTESIAN_POINT ( 'NONE',  ( -27.98221281347037959, 18.00000000000000711, -5.670874406215274277 ) ) ;
#14117=VERTEX_POINT ( 'NONE', #8075 ) ;
#14126=AXIS2_PLACEMENT_3D ( 'NONE', #8555, #15460, #2010 ) ;
#14127=ORIENTED_EDGE ( 'NONE', *, *, #10336, .F. ) ;
#14129=CARTESIAN_POINT ( 'NONE',  ( -27.94760966554430937, 19.99999999999999645, -6.338314452217975514 ) ) ;
#14130=VERTEX_POINT ( 'NONE', #13490 ) ;
#14131=LINE ( 'NONE', #1998, #16387 ) ;
#14133=EDGE_LOOP ( 'NONE', ( #14215, #3941, #12290, #17437 ) ) ;
#14136=AXIS2_PLACEMENT_3D ( 'NONE', #7148, #6883, #413 ) ;
#14137=VERTEX_POINT ( 'NONE', #1526 ) ;
#14138=SURFACE_STYLE_FILL_AREA ( #3063 ) ;
#14140=EDGE_LOOP ( 'NONE', ( #17002, #15235, #2024, #4536 ) ) ;
#14143=CARTESIAN_POINT ( 'NONE',  ( 23.34456489498957055, 143.1309386941325101, -16.67123533649925449 ) ) ;
#14144=CARTESIAN_POINT ( 'NONE',  ( -82.50000000000001421, 196.6227766016838245, -16.00000000000000000 ) ) ;
#14146=DIRECTION ( 'NONE',  ( -1.000000000000000000, -0.000000000000000000, -0.000000000000000000 ) ) ;
#14150=CIRCLE ( 'NONE', #13295, 5.999999999999998224 ) ;
#14152=FACE_OUTER_BOUND ( 'NONE', #1600, .T. ) ;
#14153=VECTOR ( 'NONE', #3180, 1000.000000000000000 ) ;
#14154=CARTESIAN_POINT ( 'NONE',  ( -12.97728802729275088, 19.99999999999999645, -11.64645903342270827 ) ) ;
#14160=ORIENTED_EDGE ( 'NONE', *, *, #12799, .T. ) ;
#14162=EDGE_CURVE ( 'NONE', #3065, #16797, #16653, .T. ) ;
#14163=CARTESIAN_POINT ( 'NONE',  ( -74.00000000000001421, 196.6227766016838245, -35.00000000000000000 ) ) ;
#14164=ADVANCED_FACE ( 'NONE', ( #15248 ), #5613, .T. ) ;
#14166=ADVANCED_FACE ( 'NONE', ( #7372, #13847, #8430 ), #555, .F. ) ;
#14168=CARTESIAN_POINT ( 'NONE',  ( 15.56337975240373872, 125.2134999403456135, -4.999999999999997335 ) ) ;
#14169=EDGE_LOOP ( 'NONE', ( #9062, #5297, #15873, #3901 ) ) ;
#14170=DIRECTION ( 'NONE',  ( 1.000000000000000000, 0.000000000000000000, -8.673617379884037937E-17 ) ) ;
#14173=CARTESIAN_POINT ( 'NONE',  ( 26.85383255238284761, 201.7487681645689861, -17.82060658420952493 ) ) ;
#14174=ORIENTED_EDGE ( 'NONE', *, *, #8799, .F. ) ;
#14176=ORIENTED_EDGE ( 'NONE', *, *, #12456, .F. ) ;
#14177=CARTESIAN_POINT ( 'NONE',  ( 19.93228116232496205, 29.93335004877557282, -13.66730128329526650 ) ) ;
#14178=CARTESIAN_POINT ( 'NONE',  ( 26.51307711398865408, 139.5431919169737967, -7.747420853565629706 ) ) ;
#14190=LINE ( 'NONE', #1071, #13434 ) ;
#14195=FACE_OUTER_BOUND ( 'NONE', #16527, .T. ) ;
#14196=ORIENTED_EDGE ( 'NONE', *, *, #884, .F. ) ;
#14207=CARTESIAN_POINT ( 'NONE',  ( -3.000000000000002665, 144.1839557653416080, -18.33333333333336057 ) ) ;
#14208=LINE ( 'NONE', #11538, #6325 ) ;
#14209=ORIENTED_EDGE ( 'NONE', *, *, #3030, .T. ) ;
#14210=DIRECTION ( 'NONE',  ( -0.000000000000000000, -0.000000000000000000, 1.000000000000000000 ) ) ;
#14212=ORIENTED_EDGE ( 'NONE', *, *, #13749, .T. ) ;
#14215=ORIENTED_EDGE ( 'NONE', *, *, #11617, .F. ) ;
#14216=ORIENTED_EDGE ( 'NONE', *, *, #1922, .T. ) ;
#14221=CARTESIAN_POINT ( 'NONE',  ( 22.50000000000001421, 146.0571958828608672, -20.88424858573642595 ) ) ;
#14230=CARTESIAN_POINT ( 'NONE',  ( -10.87333020471588974, 20.00000000000114753, -13.51515657978521645 ) ) ;
#14232=EDGE_CURVE ( 'NONE', #4814, #4046, #5046, .T. ) ;
#14234=DIRECTION ( 'NONE',  ( -1.000000000000000000, -0.000000000000000000, 0.000000000000000000 ) ) ;
#14237=ORIENTED_EDGE ( 'NONE', *, *, #2959, .T. ) ;
#14239=DIRECTION ( 'NONE',  ( 1.000000000000000000, 0.000000000000000000, 0.000000000000000000 ) ) ;
#14243=CARTESIAN_POINT ( 'NONE',  ( -80.00000000000002842, 146.6227766016838245, -35.00000000000000000 ) ) ;
#14245=CARTESIAN_POINT ( 'NONE',  ( 31.43242313191838022, 202.4505251070389420, -16.57269434321683477 ) ) ;
#14249=EDGE_CURVE ( 'NONE', #9334, #3454, #3782, .T. ) ;
#14251=CARTESIAN_POINT ( 'NONE',  ( 25.49876332522151401, 19.99999999999999645, -21.99427390110736624 ) ) ;
#14255=CARTESIAN_POINT ( 'NONE',  ( 6.134011831684059501, 134.2062027339443944, -13.00000000000000000 ) ) ;
#14258=FACE_OUTER_BOUND ( 'NONE', #13100, .T. ) ;
#14260=DIRECTION ( 'NONE',  ( -1.000000000000000000, -0.000000000000000000, -0.000000000000000000 ) ) ;
#14262=VECTOR ( 'NONE', #6705, 1000.000000000000000 ) ;
#14264=DIRECTION ( 'NONE',  ( 0.000000000000000000, 0.000000000000000000, -1.000000000000000000 ) ) ;
#14266=DIRECTION ( 'NONE',  ( -1.000000000000000000, -0.000000000000000000, 0.000000000000000000 ) ) ;
#14269=DIRECTION ( 'NONE',  ( 0.000000000000000000, 0.000000000000000000, 1.000000000000000000 ) ) ;
#14270=VERTEX_POINT ( 'NONE', #10195 ) ;
#14273=AXIS2_PLACEMENT_3D ( 'NONE', #2133, #15768, #2311 ) ;
#14275=ORIENTED_EDGE ( 'NONE', *, *, #5544, .F. ) ;
#14278=LINE ( 'NONE', #11696, #13042 ) ;
#14280=CARTESIAN_POINT ( 'NONE',  ( -100.0000000000000000, 171.6227766016838245, 0.000000000000000000 ) ) ;
#14285=AXIS2_PLACEMENT_3D ( 'NONE', #6651, #1243, #16133 ) ;
#14288=CARTESIAN_POINT ( 'NONE',  ( 32.21490539657202845, 191.0296277843086727, -29.12775510238319399 ) ) ;
#14291=AXIS2_PLACEMENT_3D ( 'NONE', #14859, #16380, #16466 ) ;
#14294=EDGE_LOOP ( 'NONE', ( #7377, #6878, #6360, #1093 ) ) ;
#14296=VERTEX_POINT ( 'NONE', #11610 ) ;
#14299=CARTESIAN_POINT ( 'NONE',  ( -24.94987437106621542, 20.00000000000004263, -5.999999999999992895 ) ) ;
#14301=DIRECTION ( 'NONE',  ( 0.000000000000000000, -0.8660254037844413721, -0.4999999999999953371 ) ) ;
#14303=ADVANCED_FACE ( 'NONE', ( #4963 ), #15595, .F. ) ;
#14304=EDGE_LOOP ( 'NONE', ( #3607, #11029 ) ) ;
#14306=DIRECTION ( 'NONE',  ( 0.000000000000000000, 0.9938079899999066047, 0.1111111111111111188 ) ) ;
#14308=PLANE ( 'NONE',  #4214 ) ;
#14310=EDGE_CURVE ( 'NONE', #10464, #13669, #2223, .T. ) ;
#14314=DIRECTION ( 'NONE',  ( -0.000000000000000000, -0.000000000000000000, 1.000000000000000000 ) ) ;
#14315=ORIENTED_EDGE ( 'NONE', *, *, #6887, .F. ) ;
#14317=DIRECTION ( 'NONE',  ( 1.000000000000000000, 0.000000000000000000, 0.000000000000000000 ) ) ;
#14319=LINE ( 'NONE', #10067, #10742 ) ;
#14321=AXIS2_PLACEMENT_3D ( 'NONE', #6466, #14440, #9115 ) ;
#14326=ORIENTED_EDGE ( 'NONE', *, *, #12254, .F. ) ;
#14327=CARTESIAN_POINT ( 'NONE',  ( -48.00000000000000000, 204.6227766016838245, 0.000000000000000000 ) ) ;
#14330=CARTESIAN_POINT ( 'NONE',  ( 50.00000000000000000, 171.6227766016838245, 0.000000000000000000 ) ) ;
#14332=VERTEX_POINT ( 'NONE', #15673 ) ;
#14334=CARTESIAN_POINT ( 'NONE',  ( 21.03709756577793399, 29.91885446100015145, -12.94894061605241831 ) ) ;
#14336=AXIS2_PLACEMENT_3D ( 'NONE', #8304, #6898, #12296 ) ;
#14340=AXIS2_PLACEMENT_3D ( 'NONE', #8019, #5550, #4228 ) ;
#14342=VERTEX_POINT ( 'NONE', #11520 ) ;
#14343=CARTESIAN_POINT ( 'NONE',  ( 35.89213624354478327, 201.2861607625691818, -14.48320912595415422 ) ) ;
#14344=B_SPLINE_CURVE_WITH_KNOTS ( 'NONE', 3,
 ( #2684, #1358, #5244, #1448 ),
 .UNSPECIFIED., .F., .F.,
 ( 4, 4 ),
 ( 0.004999999999999983624, 0.009999999999999993269 ),
 .UNSPECIFIED. ) ;
#14346=ADVANCED_FACE ( 'NONE', ( #904 ), #9036, .T. ) ;
#14351=AXIS2_PLACEMENT_3D ( 'NONE', #2561, #9182, #11928 ) ;
#14352=CARTESIAN_POINT ( 'NONE',  ( -45.00000000000000000, 130.0000000000000000, -15.00000000000000000 ) ) ;
#14354=AXIS2_PLACEMENT_3D ( 'NONE', #3802, #8045, #14862 ) ;
#14355=CARTESIAN_POINT ( 'NONE',  ( 31.05826940171251138, 140.7111270992951404, -16.41570701070894245 ) ) ;
#14356=ORIENTED_EDGE ( 'NONE', *, *, #1727, .T. ) ;
#14358=ORIENTED_EDGE ( 'NONE', *, *, #6625, .F. ) ;
#14360=CARTESIAN_POINT ( 'NONE',  ( -27.29618490519992591, 18.00000000000000000, -10.29570512375934044 ) ) ;
#14366=AXIS2_PLACEMENT_3D ( 'NONE', #4512, #260, #9814 ) ;
#14372=DIRECTION ( 'NONE',  ( 0.000000000000000000, 0.000000000000000000, 1.000000000000000000 ) ) ;
#14373=CARTESIAN_POINT ( 'NONE',  ( 33.78675088369337942, 190.1432158455537262, -27.31345131271290327 ) ) ;
#14375=CARTESIAN_POINT ( 'NONE',  ( -27.84784281930893357, 18.00000000000000000, -7.647248539284095870 ) ) ;
#14376=ORIENTED_EDGE ( 'NONE', *, *, #15204, .F. ) ;
#14380=CARTESIAN_POINT ( 'NONE',  ( 24.00000000000001066, 196.3062978594714707, -24.81790219152271604 ) ) ;
#14381=AXIS2_PLACEMENT_3D ( 'NONE', #242, #9793, #13795 ) ;
#14382=CARTESIAN_POINT ( 'NONE',  ( -45.00000000000000000, 140.0000000000000000, -15.00000000000000000 ) ) ;
#14386=ORIENTED_EDGE ( 'NONE', *, *, #7843, .T. ) ;
#14387=ADVANCED_FACE ( 'NONE', ( #643 ), #6040, .F. ) ;
#14388=CARTESIAN_POINT ( 'NONE',  ( -82.26120111208031460, 153.7971187266995514, -27.77174765869275674 ) ) ;
#14392=CIRCLE ( 'NONE', #6480, 2.500000000000002220 ) ;
#14403=ORIENTED_EDGE ( 'NONE', *, *, #12167, .T. ) ;
#14404=CARTESIAN_POINT ( 'NONE',  ( -80.00000000000001421, 196.6227766016838245, -13.00000000000000000 ) ) ;
#14411=PLANE ( 'NONE',  #12930 ) ;
#14412=DIRECTION ( 'NONE',  ( -0.000000000000000000, -0.000000000000000000, -1.000000000000000000 ) ) ;
#14413=ORIENTED_EDGE ( 'NONE', *, *, #10509, .T. ) ;
#14416=DIRECTION ( 'NONE',  ( -1.000000000000000000, -0.000000000000000000, -0.000000000000000000 ) ) ;
#14418=EDGE_CURVE ( 'NONE', #7915, #1561, #8996, .T. ) ;
#14419=VECTOR ( 'NONE', #523, 1000.000000000000000 ) ;
#14420=LINE ( 'NONE', #4775, #1534 ) ;
#14421=EDGE_CURVE ( 'NONE', #4566, #6914, #14794, .T. ) ;
#14423=DIRECTION ( 'NONE',  ( -0.000000000000000000, -0.000000000000000000, 1.000000000000000000 ) ) ;
#14426=CARTESIAN_POINT ( 'NONE',  ( 25.68011308532417303, 200.8020376890377179, -19.33395870482234713 ) ) ;
#14429=CARTESIAN_POINT ( 'NONE',  ( 18.15033819753324806, 29.95689775512239805, -14.47405640211066213 ) ) ;
#14430=CIRCLE ( 'NONE', #17242, 5.000000000000018652 ) ;
#14433=VERTEX_POINT ( 'NONE', #10627 ) ;
#14434=CARTESIAN_POINT ( 'NONE',  ( -77.20768774440396953, 151.9379092097359489, -28.93992015514736238 ) ) ;
#14435=AXIS2_PLACEMENT_3D ( 'NONE', #16792, #15546, #3424 ) ;
#14436=CARTESIAN_POINT ( 'NONE',  ( 14.80221254542069076, 126.7206120434983490, -7.900896541359456293 ) ) ;
#14439=LINE ( 'NONE', #12783, #230 ) ;
#14440=DIRECTION ( 'NONE',  ( 0.000000000000000000, 0.000000000000000000, 1.000000000000000000 ) ) ;
#14441=FACE_OUTER_BOUND ( 'NONE', #3282, .T. ) ;
#14442=AXIS2_PLACEMENT_3D ( 'NONE', #16443, #4305, #8360 ) ;
#14444=CARTESIAN_POINT ( 'NONE',  ( -45.00000000000001421, 124.1421356237309368, -15.00000000000000355 ) ) ;
#14447=CARTESIAN_POINT ( 'NONE',  ( 7.376038361426209278, 142.5209969267753536, -19.44444444444444642 ) ) ;
#14449=CYLINDRICAL_SURFACE ( 'NONE', #14632, 7.500000000000020428 ) ;
#14450=CARTESIAN_POINT ( 'NONE',  ( -17.58288004918493996, 18.00000000000000000, -22.43027208364173575 ) ) ;
#14451=EDGE_CURVE ( 'NONE', #7474, #1173, #2091, .T. ) ;
#14456=ORIENTED_EDGE ( 'NONE', *, *, #6876, .F. ) ;
#14457=PLANE ( 'NONE',  #3566 ) ;
#14459=DIRECTION ( 'NONE',  ( -1.000000000000000000, 0.000000000000000000, 0.000000000000000000 ) ) ;
#14460=CARTESIAN_POINT ( 'NONE',  ( -16.01409026037699945, 32.68451876144969503, -7.109513113881434698 ) ) ;
#14461=ORIENTED_EDGE ( 'NONE', *, *, #5277, .F. ) ;
#14462=CARTESIAN_POINT ( 'NONE',  ( -35.49999999999998579, 10.00000000000000178, -35.00200000000000244 ) ) ;
#14464=ORIENTED_EDGE ( 'NONE', *, *, #2749, .F. ) ;
#14465=CARTESIAN_POINT ( 'NONE',  ( 25.17961895204159717, 193.0449522123385577, -27.67906398090707398 ) ) ;
#14474=CARTESIAN_POINT ( 'NONE',  ( -86.97967542706145139, 149.4008433394086808, -24.40281628369249134 ) ) ;
#14475=ORIENTED_EDGE ( 'NONE', *, *, #11902, .F. ) ;
#14478=CARTESIAN_POINT ( 'NONE',  ( 26.46257777440031944, 151.4735692324752847, -28.61877689333859465 ) ) ;
#14483=CARTESIAN_POINT ( 'NONE',  ( -100.0000000000000000, 171.6227766016838245, 0.000000000000000000 ) ) ;
#14484=CARTESIAN_POINT ( 'NONE',  ( -32.99999999999998579, 10.00000000000000000, -12.99999999999999822 ) ) ;
#14488=CARTESIAN_POINT ( 'NONE',  ( -87.05152766480232174, 144.0220640066157785, -18.10843944793621674 ) ) ;
#14491=DIRECTION ( 'NONE',  ( 8.673617379884037937E-17, 0.000000000000000000, 1.000000000000000000 ) ) ;
#14496=CARTESIAN_POINT ( 'NONE',  ( 15.45450437963097912, 29.98942126207016301, -13.00000000000000178 ) ) ;
#14497=CARTESIAN_POINT ( 'NONE',  ( -79.45873686621193599, 140.6457587561385196, -16.29186131275298877 ) ) ;
#14501=CARTESIAN_POINT ( 'NONE',  ( 27.99999999999998224, 9.999999999999998224, -13.00000000000000000 ) ) ;
#14502=EDGE_CURVE ( 'NONE', #7894, #13323, #1432, .T. ) ;
#14503=DIRECTION ( 'NONE',  ( 0.000000000000000000, 0.000000000000000000, -1.000000000000000000 ) ) ;
#14504=EDGE_CURVE ( 'NONE', #14117, #16962, #14875, .T. ) ;
#14505=CARTESIAN_POINT ( 'NONE',  ( 34.33044734696805733, 200.7908024820229969, -19.35080275744229894 ) ) ;
#14506=VERTEX_POINT ( 'NONE', #11868 ) ;
#14509=ORIENTED_EDGE ( 'NONE', *, *, #5737, .F. ) ;
#14510=CARTESIAN_POINT ( 'NONE',  ( -80.00000000000001421, 196.6227766016838245, 0.000000000000000000 ) ) ;
#14512=CARTESIAN_POINT ( 'NONE',  ( 10.09659264799822331, 132.0789811519323962, -12.16719622200489681 ) ) ;
#14518=CARTESIAN_POINT ( 'NONE',  ( 48.00000000000000711, 183.6227766016837961, -5.571800142134975431 ) ) ;
#14523=DIRECTION ( 'NONE',  ( 0.000000000000000000, 0.8660254037844413721, 0.4999999999999952816 ) ) ;
#14524=ORIENTED_EDGE ( 'NONE', *, *, #13072, .T. ) ;
#14526=CARTESIAN_POINT ( 'NONE',  ( 0.000000000000000000, 20.00000000000000000, 0.000000000000000000 ) ) ;
#14533=CARTESIAN_POINT ( 'NONE',  ( -5.000000000000000888, 206.6227766016838245, 2.143131898507868248E-15 ) ) ;
#14538=CARTESIAN_POINT ( 'NONE',  ( 24.91436539010480544, 191.1044234702846154, -26.63673872167001022 ) ) ;
#14540=ADVANCED_FACE ( 'NONE', ( #12814 ), #11736, .F. ) ;
#14541=CARTESIAN_POINT ( 'NONE',  ( -14.07899634757819385, 32.11373924370096233, -10.33209047619764753 ) ) ;
#14544=VERTEX_POINT ( 'NONE', #13340 ) ;
#14545=CARTESIAN_POINT ( 'NONE',  ( 29.55074376293165628, 190.6352453962669813, -29.38582951075080629 ) ) ;
#14547=AXIS2_PLACEMENT_3D ( 'NONE', #3203, #14009, #1878 ) ;
#14548=ORIENTED_EDGE ( 'NONE', *, *, #1030, .F. ) ;
#14549=CIRCLE ( 'NONE', #12568, 8.000000000000000000 ) ;
#14550=ORIENTED_EDGE ( 'NONE', *, *, #17042, .T. ) ;
#14551=ORIENTED_EDGE ( 'NONE', *, *, #13072, .F. ) ;
#14552=CARTESIAN_POINT ( 'NONE',  ( -84.46470488465458004, 152.6548696709631372, -27.00480063125522889 ) ) ;
#14558=AXIS2_PLACEMENT_3D ( 'NONE', #12500, #11425, #4797 ) ;
#14559=CARTESIAN_POINT ( 'NONE',  ( 33.52233917118052631, 151.4845562501470226, -28.62650789566041354 ) ) ;
#14560=ADVANCED_FACE ( 'NONE', ( #9257 ), #14308, .F. ) ;
#14566=ORIENTED_EDGE ( 'NONE', *, *, #15661, .F. ) ;
#14569=CYLINDRICAL_SURFACE ( 'NONE', #7631, 2.500000000000000444 ) ;
#14571=CARTESIAN_POINT ( 'NONE',  ( -15.33310217281973209, 19.99999999999540634, -5.462585411291382975 ) ) ;
#14572=ORIENTED_EDGE ( 'NONE', *, *, #4576, .F. ) ;
#14575=CARTESIAN_POINT ( 'NONE',  ( -15.00000000000002132, 90.00000000000000000, -15.00000000000000000 ) ) ;
#14576=ORIENTED_EDGE ( 'NONE', *, *, #3196, .F. ) ;
#14577=AXIS2_PLACEMENT_3D ( 'NONE', #12514, #5616, #1800 ) ;
#14580=FILL_AREA_STYLE ('',( #5115 ) ) ;
#14582=DIRECTION ( 'NONE',  ( 0.000000000000000000, 0.000000000000000000, 1.000000000000000000 ) ) ;
#14583=DIRECTION ( 'NONE',  ( -1.000000000000000000, -0.000000000000000000, -0.000000000000000000 ) ) ;
#14586=CIRCLE ( 'NONE', #10056, 2.500000000000002220 ) ;
#14589=DIRECTION ( 'NONE',  ( 0.000000000000000000, 0.000000000000000000, -1.000000000000000000 ) ) ;
#14591=AXIS2_PLACEMENT_3D ( 'NONE', #14382, #6150, #16960 ) ;
#14592=DIRECTION ( 'NONE',  ( 8.673617379884037937E-17, 0.000000000000000000, 1.000000000000000000 ) ) ;
#14597=VERTEX_POINT ( 'NONE', #6607 ) ;
#14598=CARTESIAN_POINT ( 'NONE',  ( -84.70257449537420769, 150.3543615375532738, -27.79730406782767105 ) ) ;
#14599=AXIS2_PLACEMENT_3D ( 'NONE', #16564, #357, #4439 ) ;
#14600=CARTESIAN_POINT ( 'NONE',  ( 11.63249183333955017, 139.6944596454877114, -10.84829254633709539 ) ) ;
#14601=CIRCLE ( 'NONE', #16871, 2.500000000000002220 ) ;
#14602=ORIENTED_EDGE ( 'NONE', *, *, #1140, .T. ) ;
#14603=FACE_OUTER_BOUND ( 'NONE', #2077, .T. ) ;
#14605=CARTESIAN_POINT ( 'NONE',  ( -5.000000000000000888, 171.6227766016838245, 0.000000000000000000 ) ) ;
#14606=EDGE_CURVE ( 'NONE', #16282, #6756, #2440, .T. ) ;
#14609=DIRECTION ( 'NONE',  ( 0.000000000000000000, 0.000000000000000000, -1.000000000000000000 ) ) ;
#14610=CARTESIAN_POINT ( 'NONE',  ( 23.03715179780268585, 17.99999999999999289, -6.069068567132035241 ) ) ;
#14614=CARTESIAN_POINT ( 'NONE',  ( 25.67867739143054706, 142.4452037501736186, -19.33642647557003613 ) ) ;
#14615=VERTEX_POINT ( 'NONE', #6428 ) ;
#14616=CARTESIAN_POINT ( 'NONE',  ( 13.59940502541562246, 130.1762661646492063, -12.36432683418100353 ) ) ;
#14617=DIRECTION ( 'NONE',  ( -0.000000000000000000, -0.000000000000000000, 1.000000000000000000 ) ) ;
#14621=DIRECTION ( 'NONE',  ( -1.000000000000000000, 0.000000000000000000, 0.000000000000000000 ) ) ;
#14622=AXIS2_PLACEMENT_3D ( 'NONE', #13161, #15726, #10502 ) ;
#14627=VERTEX_POINT ( 'NONE', #8900 ) ;
#14628=DIRECTION ( 'NONE',  ( 0.000000000000000000, -1.000000000000000000, -6.123233995736762338E-17 ) ) ;
#14629=ADVANCED_FACE ( 'NONE', ( #11820, #17225 ), #15901, .F. ) ;
#14630=EDGE_LOOP ( 'NONE', ( #11389, #8882 ) ) ;
#14632=AXIS2_PLACEMENT_3D ( 'NONE', #2316, #731, #3648 ) ;
#14634=CARTESIAN_POINT ( 'NONE',  ( 29.40013309498274552, 189.1412428432857951, -27.96613953460096980 ) ) ;
#14635=CARTESIAN_POINT ( 'NONE',  ( 27.48361012698979877, 126.6227766016837819, -9.278408830390956550E-15 ) ) ;
#14636=CARTESIAN_POINT ( 'NONE',  ( -11.61061639343520824, 17.99999999999767653, -9.781492982398956926 ) ) ;
#14638=EDGE_CURVE ( 'NONE', #3748, #8600, #16445, .T. ) ;
#14639=ORIENTED_EDGE ( 'NONE', *, *, #13957, .F. ) ;
#14643=CARTESIAN_POINT ( 'NONE',  ( -87.43654228017076946, 197.7288430733995597, -20.20458554073936597 ) ) ;
#14647=ORIENTED_EDGE ( 'NONE', *, *, #4504, .F. ) ;
#14649=CARTESIAN_POINT ( 'NONE',  ( -3.000000000000000888, 204.6227766016838245, 2.020667218593133100E-15 ) ) ;
#14655=CARTESIAN_POINT ( 'NONE',  ( 35.00000000000000711, 146.6227766016838245, -12.99999999999999822 ) ) ;
#14656=CARTESIAN_POINT ( 'NONE',  ( 196.0000000000000000, 191.6227766016837677, -5.571800142134975431 ) ) ;
#14659=ORIENTED_EDGE ( 'NONE', *, *, #13821, .T. ) ;
#14660=CARTESIAN_POINT ( 'NONE',  ( -70.00000000000000000, 143.0439382767972631, -16.49999999999984013 ) ) ;
#14661=CARTESIAN_POINT ( 'NONE',  ( 22.45772829400591419, 29.90035839190693778, -11.59610751512981253 ) ) ;
#14663=CARTESIAN_POINT ( 'NONE',  ( -95.00000000000000000, 171.6227766016838245, 0.000000000000000000 ) ) ;
#14666=CARTESIAN_POINT ( 'NONE',  ( -87.50000000000005684, 146.0571958828608388, -20.88424858573642595 ) ) ;
#14667=AXIS2_PLACEMENT_3D ( 'NONE', #13720, #2917, #9639 ) ;
#14674=CARTESIAN_POINT ( 'NONE',  ( 37.50000000000000711, 146.6227766016838245, -35.00200000000000244 ) ) ;
#14675=ORIENTED_EDGE ( 'NONE', *, *, #4139, .T. ) ;
#14685=DIRECTION ( 'NONE',  ( -0.000000000000000000, -0.000000000000000000, 1.000000000000000000 ) ) ;
#14686=VECTOR ( 'NONE', #3609, 1000.000000000000000 ) ;
#14688=CARTESIAN_POINT ( 'NONE',  ( 7.535032041485008492, 142.5209969262061804, -19.44444444359253410 ) ) ;
#14691=EDGE_CURVE ( 'NONE', #2797, #1250, #5917, .T. ) ;
#14693=CARTESIAN_POINT ( 'NONE',  ( -85.55727518495883999, 148.9119151679986999, -26.63478011418837710 ) ) ;
#14694=EDGE_CURVE ( 'NONE', #14615, #6145, #17508, .T. ) ;
#14695=CARTESIAN_POINT ( 'NONE',  ( 14.09268385650717015, 127.7503171827756034, -9.071975374176082241 ) ) ;
#14696=AXIS2_PLACEMENT_3D ( 'NONE', #1506, #1242, #16297 ) ;
#14700=AXIS2_PLACEMENT_3D ( 'NONE', #16918, #4795, #3462 ) ;
#14703=CARTESIAN_POINT ( 'NONE',  ( 33.88556156013721932, 18.00000000000000000, -11.42442012027869858 ) ) ;
#14705=CARTESIAN_POINT ( 'NONE',  ( 21.98114852961722576, 18.00000000000000000, -23.72829316725777815 ) ) ;
#14709=CYLINDRICAL_SURFACE ( 'NONE', #2123, 27.69059892324149530 ) ;
#14717=AXIS2_PLACEMENT_3D ( 'NONE', #5622, #128, #8348 ) ;
#14719=ORIENTED_EDGE ( 'NONE', *, *, #8828, .T. ) ;
#14729=LINE ( 'NONE', #6668, #7956 ) ;
#14730=CARTESIAN_POINT ( 'NONE',  ( -25.81900932159184592, 18.00000000000000000, -13.95463872937486194 ) ) ;
#14733=EDGE_CURVE ( 'NONE', #5007, #8095, #2036, .T. ) ;
#14734=ORIENTED_EDGE ( 'NONE', *, *, #15386, .F. ) ;
#14735=ADVANCED_FACE ( 'NONE', ( #10770 ), #5633, .T. ) ;
#14736=CARTESIAN_POINT ( 'NONE',  ( -77.20631483639103010, 189.6403081819231033, -27.64877209012309578 ) ) ;
#14737=CARTESIAN_POINT ( 'NONE',  ( -86.41998248565997187, 200.5275637277236171, -15.94334347237690785 ) ) ;
#14739=ORIENTED_EDGE ( 'NONE', *, *, #10708, .F. ) ;
#14741=CARTESIAN_POINT ( 'NONE',  ( 15.00000000000000000, 206.6227766016838245, 2.143131898507868248E-15 ) ) ;
#14747=CARTESIAN_POINT ( 'NONE',  ( 26.63786622865510267, 151.5968920417501806, -28.70510347301450693 ) ) ;
#14749=CARTESIAN_POINT ( 'NONE',  ( 49.99999999999998579, 175.6227766016838530, -16.92820660268601429 ) ) ;
#14751=ORIENTED_EDGE ( 'NONE', *, *, #2235, .T. ) ;
#14752=CARTESIAN_POINT ( 'NONE',  ( -85.93249065294895672, 197.5381456772451543, -23.52581655030730445 ) ) ;
#14753=CARTESIAN_POINT ( 'NONE',  ( 24.29886777166023393, 29.87658293154515832, -8.524716167024733338 ) ) ;
#14754=DIRECTION ( 'NONE',  ( 0.000000000000000000, 0.000000000000000000, 1.000000000000000000 ) ) ;
#14755=FACE_OUTER_BOUND ( 'NONE', #6335, .T. ) ;
#14756=CARTESIAN_POINT ( 'NONE',  ( -87.50000000000004263, 196.6227766016838245, -35.00200000000000244 ) ) ;
#14759=CARTESIAN_POINT ( 'NONE',  ( -48.00000000000000000, 171.6227766016838245, 0.000000000000000000 ) ) ;
#14760=CARTESIAN_POINT ( 'NONE',  ( -27.99999999999998224, 10.00000000000000000, -35.00000000000000000 ) ) ;
#14761=ORIENTED_EDGE ( 'NONE', *, *, #112, .F. ) ;
#14763=ORIENTED_EDGE ( 'NONE', *, *, #1538, .T. ) ;
#14766=DIRECTION ( 'NONE',  ( 8.673617379884037937E-17, 0.000000000000000000, 1.000000000000000000 ) ) ;
#14767=CARTESIAN_POINT ( 'NONE',  ( -85.73950972639505608, 144.8396561671642928, -22.53731575973596790 ) ) ;
#14774=CARTESIAN_POINT ( 'NONE',  ( 35.49999999999998579, 9.999999999999998224, -28.00000000000001066 ) ) ;
#14776=CARTESIAN_POINT ( 'NONE',  ( 26.76721132277178228, 137.4464968366854407, -7.553125767360616472 ) ) ;
#14777=VERTEX_POINT ( 'NONE', #3150 ) ;
#14778=CARTESIAN_POINT ( 'NONE',  ( -85.41162126782658959, 149.2402085794912807, -26.91083197558417339 ) ) ;
#14779=CARTESIAN_POINT ( 'NONE',  ( 15.12922779335904977, 126.1891464972476911, -7.145555214655046505 ) ) ;
#14780=VERTEX_POINT ( 'NONE', #4391 ) ;
#14781=PLANE ( 'NONE',  #16967 ) ;
#14784=CARTESIAN_POINT ( 'NONE',  ( 17.55923266082603007, 17.99999999999999645, -24.87049340120105612 ) ) ;
#14785=CARTESIAN_POINT ( 'NONE',  ( 34.42312820349192037, 18.00000000000000000, -9.539278825333477485 ) ) ;
#14790=DIRECTION ( 'NONE',  ( -0.000000000000000000, -0.000000000000000000, 1.000000000000000000 ) ) ;
#14792=CARTESIAN_POINT ( 'NONE',  ( 24.00000000000000355, 146.6227766016838245, -24.49489742783179480 ) ) ;
#14794=LINE ( 'NONE', #12046, #12120 ) ;
#14801=ORIENTED_EDGE ( 'NONE', *, *, #10509, .F. ) ;
#14804=ORIENTED_EDGE ( 'NONE', *, *, #8829, .F. ) ;
#14805=PLANE ( 'NONE',  #17436 ) ;
#14806=CARTESIAN_POINT ( 'NONE',  ( 15.58935537591275811, 125.0306660307430349, -3.338448778865417577 ) ) ;
#14807=DIRECTION ( 'NONE',  ( 1.000000000000000000, 0.000000000000000000, 0.000000000000000000 ) ) ;
#14809=ORIENTED_EDGE ( 'NONE', *, *, #9339, .F. ) ;
#14811=ORIENTED_EDGE ( 'NONE', *, *, #12564, .F. ) ;
#14812=CARTESIAN_POINT ( 'NONE',  ( -85.62055130997418928, 191.6508168144185902, -26.22852547856965444 ) ) ;
#14817=CIRCLE ( 'NONE', #11690, 6.000000000000001776 ) ;
#14818=DIRECTION ( 'NONE',  ( -0.000000000000000000, -0.000000000000000000, -1.000000000000000000 ) ) ;
#14820=PRODUCT_CONTEXT ( 'NONE', #14001, 'mechanical' ) ;
#14821=DIRECTION ( 'NONE',  ( -1.000000000000000000, -0.000000000000000000, 0.000000000000000000 ) ) ;
#14824=CARTESIAN_POINT ( 'NONE',  ( 22.42614717998981178, 29.85190128815754917, -7.820018500632365033 ) ) ;
#14828=CARTESIAN_POINT ( 'NONE',  ( -82.59122206075636541, 202.0384121146825862, -17.31838511551979565 ) ) ;
#14832=DIRECTION ( 'NONE',  ( 0.000000000000000000, 0.000000000000000000, -1.000000000000000000 ) ) ;
#14835=DIRECTION ( 'NONE',  ( -0.000000000000000000, -0.000000000000000000, 1.000000000000000000 ) ) ;
#14836=ORIENTED_EDGE ( 'NONE', *, *, #11806, .F. ) ;
#14837=DIRECTION ( 'NONE',  ( 0.000000000000000000, 0.000000000000000000, -1.000000000000000000 ) ) ;
#14838=CIRCLE ( 'NONE', #7205, 2.500000000000000000 ) ;
#14841=EDGE_CURVE ( 'NONE', #243, #16962, #17213, .T. ) ;
#14847=EDGE_CURVE ( 'NONE', #1902, #10173, #14131, .T. ) ;
#14849=CARTESIAN_POINT ( 'NONE',  ( -5.000000000000000888, 171.6227766016838245, -20.00000000000000355 ) ) ;
#14850=ADVANCED_FACE ( 'NONE', ( #1737 ), #15444, .F. ) ;
#14852=ADVANCED_FACE ( 'NONE', ( #12530 ), #1814, .T. ) ;
#14854=VECTOR ( 'NONE', #3165, 1000.000000000000114 ) ;
#14855=CIRCLE ( 'NONE', #13164, 30.00000000000000000 ) ;
#14856=CARTESIAN_POINT ( 'NONE',  ( 17.14535223351611748, 126.3036220646326910, -7.355580850454368047 ) ) ;
#14859=CARTESIAN_POINT ( 'NONE',  ( 40.00000000000000711, 171.6227766016838245, 0.000000000000000000 ) ) ;
#14860=ORIENTED_EDGE ( 'NONE', *, *, #12456, .T. ) ;
#14862=DIRECTION ( 'NONE',  ( 0.000000000000000000, 0.000000000000000000, -1.000000000000000000 ) ) ;
#14863=CARTESIAN_POINT ( 'NONE',  ( -83.36338409889501122, 191.6363561590498250, -28.71510896997970264 ) ) ;
#14865=CIRCLE ( 'NONE', #16857, 2.500000000000002220 ) ;
#14868=CARTESIAN_POINT ( 'NONE',  ( 14.93242934743711992, 18.00000000000000355, -25.00000000000000000 ) ) ;
#14869=CARTESIAN_POINT ( 'NONE',  ( 18.47042353409679194, 29.92915261368834479, -12.18054208566702279 ) ) ;
#14874=ORIENTED_EDGE ( 'NONE', *, *, #575, .F. ) ;
#14875=LINE ( 'NONE', #2756, #12393 ) ;
#14876=ORIENTED_EDGE ( 'NONE', *, *, #2631, .T. ) ;
#14883=CARTESIAN_POINT ( 'NONE',  ( 6.134011831684059501, 134.2062027339443944, -24.99999999999999645 ) ) ;
#14885=ORIENTED_EDGE ( 'NONE', *, *, #5052, .F. ) ;
#14889=ORIENTED_EDGE ( 'NONE', *, *, #5640, .T. ) ;
#14890=DIRECTION ( 'NONE',  ( -0.000000000000000000, -0.000000000000000000, -1.000000000000000000 ) ) ;
#14891=DIRECTION ( 'NONE',  ( 1.000000000000000000, 0.000000000000000000, 0.000000000000000000 ) ) ;
#14896=ORIENTED_EDGE ( 'NONE', *, *, #11396, .T. ) ;
#14899=VERTEX_POINT ( 'NONE', #10033 ) ;
#14900=CARTESIAN_POINT ( 'NONE',  ( -75.53529511534544838, 190.5906835324044550, -27.00480063125522889 ) ) ;
#14902=CARTESIAN_POINT ( 'NONE',  ( -14.96200682865387854, 32.37632742624003157, -9.274234733431431010 ) ) ;
#14906=EDGE_CURVE ( 'NONE', #457, #2935, #16015, .T. ) ;
#14909=ADVANCED_FACE ( 'NONE', ( #17298 ), #17115, .F. ) ;
#14911=EDGE_LOOP ( 'NONE', ( #13432, #17429 ) ) ;
#14913=CARTESIAN_POINT ( 'NONE',  ( -38.00000000000000000, 2.000000000000000000, -28.00000000000000355 ) ) ;
#14914=LINE ( 'NONE', #2703, #15529 ) ;
#14915=DIRECTION ( 'NONE',  ( -1.000000000000000000, -0.000000000000000000, 0.000000000000000000 ) ) ;
#14918=EDGE_LOOP ( 'NONE', ( #4271, #7092 ) ) ;
#14922=CARTESIAN_POINT ( 'NONE',  ( 29.98123639043839006, 19.99999999999999645, -18.19121573219640098 ) ) ;
#14925=AXIS2_PLACEMENT_3D ( 'NONE', #7475, #11198, #593 ) ;
#14928=DIRECTION ( 'NONE',  ( -0.000000000000000000, -1.000000000000000000, 0.000000000000000000 ) ) ;
#14929=VERTEX_POINT ( 'NONE', #2333 ) ;
#14931=VERTEX_POINT ( 'NONE', #6402 ) ;
#14932=CIRCLE ( 'NONE', #3342, 20.00000000000000355 ) ;
#14933=CARTESIAN_POINT ( 'NONE',  ( 17.00000000000000000, 171.6227766016838245, 0.000000000000000000 ) ) ;
#14936=VERTEX_POINT ( 'NONE', #3576 ) ;
#14939=DIRECTION ( 'NONE',  ( -0.000000000000000000, -0.000000000000000000, -1.000000000000000000 ) ) ;
#14942=AXIS2_PLACEMENT_3D ( 'NONE', #6011, #12912, #16899 ) ;
#14944=ORIENTED_EDGE ( 'NONE', *, *, #10791, .F. ) ;
#14947=VERTEX_POINT ( 'NONE', #1455 ) ;
#14948=CARTESIAN_POINT ( 'NONE',  ( -84.31671119272000681, 192.4368082929522075, -28.14105258436205403 ) ) ;
#14950=EDGE_CURVE ( 'NONE', #5744, #12793, #1528, .T. ) ;
#14952=CARTESIAN_POINT ( 'NONE',  ( -20.49999999999998224, 10.00000000000000000, -35.00200000000000244 ) ) ;
#14953=AXIS2_PLACEMENT_3D ( 'NONE', #10804, #16214, #4080 ) ;
#14958=DIRECTION ( 'NONE',  ( 0.000000000000000000, 0.000000000000000000, 1.000000000000000000 ) ) ;
#14960=CARTESIAN_POINT ( 'NONE',  ( 196.0000000000000000, 191.6227766016837677, -3.071800142134975431 ) ) ;
#14963=CARTESIAN_POINT ( 'NONE',  ( 196.0000000000000000, 155.6227766016839098, -10.00000337241049309 ) ) ;
#14967=DIRECTION ( 'NONE',  ( 0.000000000000000000, 0.000000000000000000, 1.000000000000000000 ) ) ;
#14968=AXIS2_PLACEMENT_3D ( 'NONE', #5150, #6216, #10538 ) ;
#14972=DIRECTION ( 'NONE',  ( 1.000000000000000000, 0.000000000000000000, 0.000000000000000000 ) ) ;
#14973=EDGE_LOOP ( 'NONE', ( #9237, #12545 ) ) ;
#14974=CARTESIAN_POINT ( 'NONE',  ( 23.64306072442660422, 150.6299487802827741, -25.46745035168473237 ) ) ;
#14977=DIRECTION ( 'NONE',  ( 0.000000000000000000, -1.000000000000000000, 0.000000000000000000 ) ) ;
#14981=DIRECTION ( 'NONE',  ( 1.000000000000000000, 0.000000000000000000, -0.000000000000000000 ) ) ;
#14983=ORIENTED_EDGE ( 'NONE', *, *, #13790, .F. ) ;
#14989=CARTESIAN_POINT ( 'NONE',  ( -16.22141882056480355, 32.74469488918423821, -6.141726134091478606 ) ) ;
#14990=ORIENTED_EDGE ( 'NONE', *, *, #5157, .T. ) ;
#14996=CIRCLE ( 'NONE', #14717, 10.00000000000000000 ) ;
#14997=ORIENTED_EDGE ( 'NONE', *, *, #7355, .F. ) ;
#14999=CYLINDRICAL_SURFACE ( 'NONE', #2425, 7.500000000000020428 ) ;
#15000=CARTESIAN_POINT ( 'NONE',  ( 18.47699279854304777, 29.92902263789611439, -12.17729482734268132 ) ) ;
#15002=CARTESIAN_POINT ( 'NONE',  ( 48.00000000000000711, 187.6227766016837961, -15.00000337241049486 ) ) ;
#15004=CARTESIAN_POINT ( 'NONE',  ( -76.52069396612810692, 201.5149201033276256, -18.20725769141078487 ) ) ;
#15006=EDGE_CURVE ( 'NONE', #9729, #9167, #10907, .T. ) ;
#15008=DIRECTION ( 'NONE',  ( 0.000000000000000000, 0.000000000000000000, 1.000000000000000000 ) ) ;
#15009=EDGE_CURVE ( 'NONE', #2789, #10402, #14392, .T. ) ;
#15010=DIRECTION ( 'NONE',  ( -2.312964634635742464E-16, 0.000000000000000000, -1.000000000000000000 ) ) ;
#15011=CARTESIAN_POINT ( 'NONE',  ( -43.00000000000000711, 130.0000000000000000, -12.99999999999999822 ) ) ;
#15012=DIRECTION ( 'NONE',  ( -1.000000000000000000, 0.000000000000000000, 0.000000000000000000 ) ) ;
#15020=DIRECTION ( 'NONE',  ( 0.000000000000000000, 0.000000000000000000, 1.000000000000000000 ) ) ;
#15022=VERTEX_POINT ( 'NONE', #2689 ) ;
#15025=CARTESIAN_POINT ( 'NONE',  ( 0.000000000000000000, 18.00000000000000355, 0.000000000000000000 ) ) ;
#15026=LINE ( 'NONE', #13805, #12872 ) ;
#15027=CARTESIAN_POINT ( 'NONE',  ( 17.42040306417330342, 125.8667821340875577, -6.358709916038607801 ) ) ;
#15028=ORIENTED_EDGE ( 'NONE', *, *, #6133, .F. ) ;
#15029=DIRECTION ( 'NONE',  ( 1.000000000000000000, 0.000000000000000000, 0.000000000000000000 ) ) ;
#15030=DIRECTION ( 'NONE',  ( 1.000000000000000000, 0.000000000000000000, 0.000000000000000000 ) ) ;
#15031=ORIENTED_EDGE ( 'NONE', *, *, #6577, .T. ) ;
#15032=CARTESIAN_POINT ( 'NONE',  ( -74.95488020859191636, 193.3541989604593425, -27.43934207688683813 ) ) ;
#15033=CYLINDRICAL_SURFACE ( 'NONE', #5325, 7.500000000000007105 ) ;
#15034=EDGE_CURVE ( 'NONE', #3748, #1902, #2281, .T. ) ;
#15035=LINE ( 'NONE', #263, #17149 ) ;
#15037=CARTESIAN_POINT ( 'NONE',  ( 34.26588824652853305, 18.00000000000000000, -10.16858984204336736 ) ) ;
#15038=DIRECTION ( 'NONE',  ( -1.000000000000000000, 0.000000000000000000, 0.000000000000000000 ) ) ;
#15039=CARTESIAN_POINT ( 'NONE',  ( 196.0000000000000000, 167.6227766016838530, -5.571800142134975431 ) ) ;
#15043=CARTESIAN_POINT ( 'NONE',  ( -25.16839285024614625, 19.99999999999999645, -15.12082343620048519 ) ) ;
#15044=ORIENTED_EDGE ( 'NONE', *, *, #5544, .T. ) ;
#15048=ORIENTED_EDGE ( 'NONE', *, *, #5218, .F. ) ;
#15050=DIRECTION ( 'NONE',  ( -0.000000000000000000, -0.000000000000000000, 1.000000000000000000 ) ) ;
#15053=CARTESIAN_POINT ( 'NONE',  ( 36.08081429761088543, 151.0194919042433241, -25.77925661938085611 ) ) ;
#15054=ORIENTED_EDGE ( 'NONE', *, *, #7681, .T. ) ;
#15055=EDGE_CURVE ( 'NONE', #11435, #7753, #4459, .T. ) ;
#15056=CARTESIAN_POINT ( 'NONE',  ( 35.45515645957151918, 191.4518784269448588, -26.38258506112510560 ) ) ;
#15057=CARTESIAN_POINT ( 'NONE',  ( 196.0000000000000000, 175.6227766016838245, -8.071800142134975431 ) ) ;
#15060=CARTESIAN_POINT ( 'NONE',  ( -24.99999999999999289, 90.00000000000000000, -15.00000000000000000 ) ) ;
#15061=ORIENTED_EDGE ( 'NONE', *, *, #8585, .T. ) ;
#15066=DIRECTION ( 'NONE',  ( 1.000000000000000000, 0.000000000000000000, -0.000000000000000000 ) ) ;
#15067=DIRECTION ( 'NONE',  ( -1.000000000000000000, -0.000000000000000000, 0.000000000000000000 ) ) ;
#15068=ADVANCED_FACE ( 'NONE', ( #12590 ), #4549, .F. ) ;
#15070=ORIENTED_EDGE ( 'NONE', *, *, #6679, .T. ) ;
#15072=DIRECTION ( 'NONE',  ( 0.000000000000000000, 0.000000000000000000, -1.000000000000000000 ) ) ;
#15078=CYLINDRICAL_SURFACE ( 'NONE', #12050, 7.500000000000000000 ) ;
#15079=CARTESIAN_POINT ( 'NONE',  ( 22.73104287435775461, 29.84603067649059227, -6.814483377121257845 ) ) ;
#15082=VERTEX_POINT ( 'NONE', #9846 ) ;
#15087=LINE ( 'NONE', #3056, #9503 ) ;
#15089=ORIENTED_EDGE ( 'NONE', *, *, #11203, .T. ) ;
#15091=DIRECTION ( 'NONE',  ( 1.000000000000000000, -0.000000000000000000, -0.000000000000000000 ) ) ;
#15096=CARTESIAN_POINT ( 'NONE',  ( -48.00000000000000000, 171.6227766016838245, 0.000000000000000000 ) ) ;
#15097=EDGE_CURVE ( 'NONE', #13521, #3793, #4632, .T. ) ;
#15099=CIRCLE ( 'NONE', #7468, 2.499999999999998668 ) ;
#15102=ORIENTED_EDGE ( 'NONE', *, *, #5920, .F. ) ;
#15104=FACE_OUTER_BOUND ( 'NONE', #1658, .T. ) ;
#15107=VECTOR ( 'NONE', #2050, 1000.000000000000000 ) ;
#15108=VECTOR ( 'NONE', #15180, 1000.000000000000000 ) ;
#15109=LINE ( 'NONE', #9537, #11248 ) ;
#15110=ORIENTED_EDGE ( 'NONE', *, *, #4029, .F. ) ;
#15113=ORIENTED_EDGE ( 'NONE', *, *, #5788, .T. ) ;
#15115=DIRECTION ( 'NONE',  ( 0.000000000000000000, 0.000000000000000000, 1.000000000000000000 ) ) ;
#15126=DIRECTION ( 'NONE',  ( -0.000000000000000000, -0.000000000000000000, -1.000000000000000000 ) ) ;
#15127=ORIENTED_EDGE ( 'NONE', *, *, #9480, .F. ) ;
#15128=ORIENTED_EDGE ( 'NONE', *, *, #2696, .F. ) ;
#15129=CARTESIAN_POINT ( 'NONE',  ( 22.87244304995705235, 29.89498257257996272, -11.09085247437311494 ) ) ;
#15137=AXIS2_PLACEMENT_3D ( 'NONE', #12640, #7070, #5915 ) ;
#15138=CARTESIAN_POINT ( 'NONE',  ( 22.50000000000002132, 146.8102797458443831, -21.75827460206394903 ) ) ;
#15140=DIRECTION ( 'NONE',  ( -1.000000000000000000, 0.000000000000000000, 0.000000000000000000 ) ) ;
#15141=CYLINDRICAL_SURFACE ( 'NONE', #15733, 2.500000000000000444 ) ;
#15142=FACE_BOUND ( 'NONE', #7088, .T. ) ;
#15149=CARTESIAN_POINT ( 'NONE',  ( -100.0000000000000000, 171.6227766016838245, 0.000000000000000000 ) ) ;
#15152=CARTESIAN_POINT ( 'NONE',  ( -72.65335638526123319, 195.0609035571773404, -23.23759988234784046 ) ) ;
#15153=CARTESIAN_POINT ( 'NONE',  ( -48.00000000000000000, 171.6227766016838245, -20.00000000000000355 ) ) ;
#15156=ORIENTED_EDGE ( 'NONE', *, *, #1703, .T. ) ;
#15157=EDGE_LOOP ( 'NONE', ( #9189, #1531 ) ) ;
#15159=LINE ( 'NONE', #3036, #7470 ) ;
#15160=DIRECTION ( 'NONE',  ( -1.000000000000000000, -0.000000000000000000, -0.000000000000000000 ) ) ;
#15164=CIRCLE ( 'NONE', #16305, 2.500000000000000000 ) ;
#15167=DIRECTION ( 'NONE',  ( -0.000000000000000000, -0.000000000000000000, 1.000000000000000000 ) ) ;
#15171=EDGE_CURVE ( 'NONE', #16623, #6275, #8181, .T. ) ;
#15172=AXIS2_PLACEMENT_3D ( 'NONE', #8486, #13809, #16379 ) ;
#15174=CARTESIAN_POINT ( 'NONE',  ( 48.00000000000000711, 175.6227766016838530, -16.92820660268601429 ) ) ;
#15177=VERTEX_POINT ( 'NONE', #4966 ) ;
#15178=CARTESIAN_POINT ( 'NONE',  ( -74.65276356201289332, 199.3666727680385975, -21.34312735376092718 ) ) ;
#15180=DIRECTION ( 'NONE',  ( 0.000000000000000000, 0.000000000000000000, 1.000000000000000000 ) ) ;
#15182=DIRECTION ( 'NONE',  ( 0.000000000000000000, 0.000000000000000000, 1.000000000000000000 ) ) ;
#15190=ORIENTED_EDGE ( 'NONE', *, *, #9422, .F. ) ;
#15192=LINE ( 'NONE', #2893, #2138 ) ;
#15194=CARTESIAN_POINT ( 'NONE',  ( -68.00000000000000000, 154.3022685259950038, -9.999999999999900524 ) ) ;
#15197=CARTESIAN_POINT ( 'NONE',  ( 21.87797949700605926, 29.86248177612424115, -9.008363892349379398 ) ) ;
#15198=AXIS2_PLACEMENT_3D ( 'NONE', #5619, #14818, #9414 ) ;
#15203=DIRECTION ( 'NONE',  ( 0.000000000000000000, 0.000000000000000000, -1.000000000000000000 ) ) ;
#15204=EDGE_CURVE ( 'NONE', #8060, #5440, #2225, .T. ) ;
#15207=AXIS2_PLACEMENT_3D ( 'NONE', #11816, #13150, #8897 ) ;
#15210=VECTOR ( 'NONE', #9381, 1000.000000000000000 ) ;
#15214=CARTESIAN_POINT ( 'NONE',  ( -74.38629067462862565, 194.4974200864254215, -26.49149599578361247 ) ) ;
#15221=DIRECTION ( 'NONE',  ( -1.000000000000000000, -0.000000000000000000, 0.000000000000000000 ) ) ;
#15222=AXIS2_PLACEMENT_3D ( 'NONE', #951, #14583, #7853 ) ;
#15225=ADVANCED_FACE ( 'NONE', ( #13114 ), #17186, .T. ) ;
#15226=ADVANCED_FACE ( 'NONE', ( #820 ), #14449, .T. ) ;
#15227=ORIENTED_EDGE ( 'NONE', *, *, #6071, .T. ) ;
#15230=CARTESIAN_POINT ( 'NONE',  ( -48.00000000000000000, 171.6227766016838245, 0.000000000000000000 ) ) ;
#15233=DIRECTION ( 'NONE',  ( 0.000000000000000000, 0.000000000000000000, 1.000000000000000000 ) ) ;
#15235=ORIENTED_EDGE ( 'NONE', *, *, #9480, .T. ) ;
#15237=VECTOR ( 'NONE', #6675, 1000.000000000000114 ) ;
#15238=CYLINDRICAL_SURFACE ( 'NONE', #1685, 2.499999999999998668 ) ;
#15239=AXIS2_PLACEMENT_3D ( 'NONE', #4560, #4641, #3221 ) ;
#15240=CYLINDRICAL_SURFACE ( 'NONE', #9345, 10.00000000000000178 ) ;
#15242=CARTESIAN_POINT ( 'NONE',  ( -85.00000000000002842, 196.6227766016838245, 0.000000000000000000 ) ) ;
#15246=CARTESIAN_POINT ( 'NONE',  ( -23.00000000000000000, 120.0000000000000284, -15.00000000000000000 ) ) ;
#15248=FACE_OUTER_BOUND ( 'NONE', #13892, .T. ) ;
#15250=ORIENTED_EDGE ( 'NONE', *, *, #3532, .F. ) ;
#15252=CIRCLE ( 'NONE', #3093, 2.500000000000000444 ) ;
#15255=VERTEX_POINT ( 'NONE', #10361 ) ;
#15256=LINE ( 'NONE', #8609, #8311 ) ;
#15259=VECTOR ( 'NONE', #278, 1000.000000000000000 ) ;
#15264=CARTESIAN_POINT ( 'NONE',  ( -80.00000000000002842, 146.6227766016838245, -16.00000000000000000 ) ) ;
#15267=EDGE_CURVE ( 'NONE', #16797, #15922, #2397, .T. ) ;
#15271=ORIENTED_EDGE ( 'NONE', *, *, #10444, .T. ) ;
#15272=CARTESIAN_POINT ( 'NONE',  ( -74.00000000000002842, 196.9987679943318142, -24.11115281963768453 ) ) ;
#15273=CARTESIAN_POINT ( 'NONE',  ( 25.49999999999998579, 9.999999999999998224, 1.387778780781445676E-14 ) ) ;
#15276=CYLINDRICAL_SURFACE ( 'NONE', #12052, 2.500000000000002220 ) ;
#15277=CIRCLE ( 'NONE', #6806, 2.500000000000000444 ) ;
#15278=EDGE_LOOP ( 'NONE', ( #1948, #6056, #3896, #14456 ) ) ;
#15279=EDGE_LOOP ( 'NONE', ( #14209, #15654 ) ) ;
#15280=AXIS2_PLACEMENT_3D ( 'NONE', #13142, #17392, #6509 ) ;
#15281=EDGE_CURVE ( 'NONE', #6709, #15643, #3952, .T. ) ;
#15284=CARTESIAN_POINT ( 'NONE',  ( -80.00000000000002842, 146.6227766016838245, -12.99999999999999822 ) ) ;
#15290=CIRCLE ( 'NONE', #9061, 7.500000000000003553 ) ;
#15292=CIRCLE ( 'NONE', #876, 8.000000000000000000 ) ;
#15303=ORIENTED_EDGE ( 'NONE', *, *, #17219, .T. ) ;
#15308=DIRECTION ( 'NONE',  ( -0.000000000000000000, -0.000000000000000000, -1.000000000000000000 ) ) ;
#15313=DIRECTION ( 'NONE',  ( -0.000000000000000000, -0.000000000000000000, 1.000000000000000000 ) ) ;
#15314=CARTESIAN_POINT ( 'NONE',  ( 48.00000000000000000, 171.6227766016838245, 0.000000000000000000 ) ) ;
#15317=CARTESIAN_POINT ( 'NONE',  ( 32.29171157738787912, 19.99999999999999645, -15.02090973094133375 ) ) ;
#15322=ORIENTED_EDGE ( 'NONE', *, *, #17160, .T. ) ;
#15323=CARTESIAN_POINT ( 'NONE',  ( 34.88846745512547187, 152.3168652870157018, -26.76420670456569084 ) ) ;
#15329=DIRECTION ( 'NONE',  ( -1.000000000000000000, 0.000000000000000000, 0.000000000000000000 ) ) ;
#15334=DIRECTION ( 'NONE',  ( -1.000000000000000000, -0.000000000000000000, -0.000000000000000000 ) ) ;
#15335=ORIENTED_EDGE ( 'NONE', *, *, #2237, .F. ) ;
#15336=CARTESIAN_POINT ( 'NONE',  ( -72.74938895237542624, 194.6575378623844870, -23.63707964515041482 ) ) ;
#15340=DIRECTION ( 'NONE',  ( -1.000000000000000000, -0.000000000000000000, 0.000000000000000000 ) ) ;
#15342=B_SPLINE_CURVE_WITH_KNOTS ( 'NONE', 3,
 ( #7184, #451, #4545, #8599, #14010, #10004, #7275, #12680, #14103, #553 ),
 .UNSPECIFIED., .F., .F.,
 ( 4, 2, 2, 2, 4 ),
 ( 1.908195823574487804E-17, 0.002588446031580681969, 0.005176892063161340519, 0.007765338094741998202, 0.01035378412632265675 ),
 .UNSPECIFIED. ) ;
#15345=FACE_OUTER_BOUND ( 'NONE', #4693, .T. ) ;
#15346=CYLINDRICAL_SURFACE ( 'NONE', #15239, 6.000000000000008882 ) ;
#15352=CARTESIAN_POINT ( 'NONE',  ( 27.48361012698968864, 138.6227766016838245, -1.063447695028166570E-14 ) ) ;
#15356=FACE_BOUND ( 'NONE', #9750, .T. ) ;
#15359=DIRECTION ( 'NONE',  ( -0.000000000000000000, -0.000000000000000000, 1.000000000000000000 ) ) ;
#15362=CYLINDRICAL_SURFACE ( 'NONE', #13217, 20.00000000000000355 ) ;
#15363=ORIENTED_EDGE ( 'NONE', *, *, #6526, .F. ) ;
#15369=EDGE_CURVE ( 'NONE', #14777, #6195, #11295, .T. ) ;
#15370=LINE ( 'NONE', #9798, #11237 ) ;
#15373=CARTESIAN_POINT ( 'NONE',  ( -12.63609539511577218, 19.99999999999999645, -24.35132453916816431 ) ) ;
#15374=DIRECTION ( 'NONE',  ( 1.000000000000000000, 0.000000000000000000, 0.000000000000000000 ) ) ;
#15378=LINE ( 'NONE', #7496, #7813 ) ;
#15379=VECTOR ( 'NONE', #11926, 1000.000000000000000 ) ;
#15380=ORIENTED_EDGE ( 'NONE', *, *, #10556, .F. ) ;
#15382=CARTESIAN_POINT ( 'NONE',  ( -85.55670654414588228, 194.3322840258869064, -26.63593000238177666 ) ) ;
#15383=EDGE_LOOP ( 'NONE', ( #6911, #14196, #11981, #2594 ) ) ;
#15386=EDGE_CURVE ( 'NONE', #4348, #2857, #16039, .T. ) ;
#15388=EDGE_CURVE ( 'NONE', #12276, #2002, #9026, .T. ) ;
#15389=ORIENTED_EDGE ( 'NONE', *, *, #17098, .F. ) ;
#15392=CARTESIAN_POINT ( 'NONE',  ( 24.93507336697364707, 29.86842105263157876, -15.00000000000000000 ) ) ;
#15393=FACE_BOUND ( 'NONE', #13955, .T. ) ;
#15395=ORIENTED_EDGE ( 'NONE', *, *, #16990, .T. ) ;
#15398=CARTESIAN_POINT ( 'NONE',  ( 33.88365274872861477, 19.99999999999999645, -11.43011099234506212 ) ) ;
#15402=LINE ( 'NONE', #894, #8359 ) ;
#15403=ORIENTED_EDGE ( 'NONE', *, *, #497, .F. ) ;
#15405=B_SPLINE_CURVE_WITH_KNOTS ( 'NONE', 3,
 ( #3411, #10031, #14129, #4825, #15691, #11454, #3574, #839, #2155, #2491, #1166, #7887, #7395, #2071, #7555, #12873, #10628, #17032, #12792, #10288, #6567, #15615, #4899, #15533, #15442, #10215 ),
 .UNSPECIFIED., .F., .F.,
 ( 4, 2, 2, 2, 2, 2, 2, 2, 2, 2, 2, 2, 4 ),
 ( 0.000000000000000000, 0.002002783134349993537, 0.004005566268699987074, 0.008011132537399970679, 0.01001391567174996812, 0.01201669880609996383, 0.01602226507479994830, 0.01802504820914994227, 0.02002783134349994318, 0.02403339761219993459, 0.02603618074654993550, 0.02803896388089993641, 0.03204453014959993129 ),
 .UNSPECIFIED. ) ;
#15406=VECTOR ( 'NONE', #1876, 1000.000000000000000 ) ;
#15410=DIRECTION ( 'NONE',  ( -1.000000000000000000, -0.000000000000000000, -0.000000000000000000 ) ) ;
#15414=LINE ( 'NONE', #1712, #11438 ) ;
#15415=VERTEX_POINT ( 'NONE', #8151 ) ;
#15416=CARTESIAN_POINT ( 'NONE',  ( 49.99999999999998579, 175.6227766016838245, -5.571800142134975431 ) ) ;
#15420=AXIS2_PLACEMENT_3D ( 'NONE', #16530, #10854, #16189 ) ;
#15422=CYLINDRICAL_SURFACE ( 'NONE', #11478, 35.00000000000000000 ) ;
#15426=ORIENTED_EDGE ( 'NONE', *, *, #14694, .T. ) ;
#15427=CARTESIAN_POINT ( 'NONE',  ( 37.50000000000000711, 146.6227766016838245, -13.00000000000000000 ) ) ;
#15431=ORIENTED_EDGE ( 'NONE', *, *, #7889, .F. ) ;
#15433=DIRECTION ( 'NONE',  ( -0.000000000000000000, -1.000000000000000000, -0.000000000000000000 ) ) ;
#15438=AXIS2_PLACEMENT_3D ( 'NONE', #4572, #9060, #7723 ) ;
#15439=CARTESIAN_POINT ( 'NONE',  ( -8.509631953695096840, 18.00000000000455103, -12.55445085332768151 ) ) ;
#15441=CARTESIAN_POINT ( 'NONE',  ( -74.00000000000001421, 196.6227766016838245, -24.49489742783179125 ) ) ;
#15442=CARTESIAN_POINT ( 'NONE',  ( -8.719536044788661400, 19.99999999999999645, -24.99999999999999645 ) ) ;
#15444=CYLINDRICAL_SURFACE ( 'NONE', #12132, 2.499999999999998668 ) ;
#15447=VERTEX_POINT ( 'NONE', #1346 ) ;
#15451=VECTOR ( 'NONE', #12156, 1000.000000000000000 ) ;
#15458=CARTESIAN_POINT ( 'NONE',  ( 24.72505082391213804, 141.2912748254776147, -13.00000000000000000 ) ) ;
#15460=DIRECTION ( 'NONE',  ( -0.000000000000000000, -0.000000000000000000, 1.000000000000000000 ) ) ;
#15461=CARTESIAN_POINT ( 'NONE',  ( 30.00000000000001066, 146.6227766016838245, -35.00200000000000244 ) ) ;
#15462=AXIS2_PLACEMENT_3D ( 'NONE', #14518, #13193, #12294 ) ;
#15466=AXIS2_PLACEMENT_3D ( 'NONE', #9637, #13639, #16556 ) ;
#15467=CARTESIAN_POINT ( 'NONE',  ( 27.99999999999998224, 9.999999999999998224, -35.00200000000000244 ) ) ;
#15469=CARTESIAN_POINT ( 'NONE',  ( -14.77653433949313744, 31.60550367499664759, -12.35354907637233701 ) ) ;
#15471=AXIS2_PLACEMENT_3D ( 'NONE', #16265, #6801, #2636 ) ;
#15475=ORIENTED_EDGE ( 'NONE', *, *, #6808, .F. ) ;
#15480=DIRECTION ( 'NONE',  ( -1.000000000000000000, -0.000000000000000000, -0.000000000000000000 ) ) ;
#15481=ORIENTED_EDGE ( 'NONE', *, *, #16579, .F. ) ;
#15482=CARTESIAN_POINT ( 'NONE',  ( 32.50000000000000000, 196.6227766016838245, -16.00000000000000000 ) ) ;
#15484=CARTESIAN_POINT ( 'NONE',  ( 7.655193733048226257, 144.1839557653416080, -18.33333333333333925 ) ) ;
#15485=EDGE_CURVE ( 'NONE', #10357, #152, #1683, .T. ) ;
#15486=CARTESIAN_POINT ( 'NONE',  ( 29.48010637980168269, 202.6059057426778622, -16.28038605903246605 ) ) ;
#15487=ORIENTED_EDGE ( 'NONE', *, *, #13013, .T. ) ;
#15489=CARTESIAN_POINT ( 'NONE',  ( 29.97257796258477569, 19.99999999999999645, -18.20111186907413270 ) ) ;
#15491=CARTESIAN_POINT ( 'NONE',  ( 26.92745052348471546, 139.3035600351462904, -6.678622460562388952 ) ) ;
#15494=FACE_BOUND ( 'NONE', #12555, .T. ) ;
#15497=ORIENTED_EDGE ( 'NONE', *, *, #15701, .F. ) ;
#15501=AXIS2_PLACEMENT_3D ( 'NONE', #6586, #15334, #8698 ) ;
#15507=CARTESIAN_POINT ( 'NONE',  ( 35.27494917608787972, 201.9542783778900059, -13.00000000000000000 ) ) ;
#15508=ORIENTED_EDGE ( 'NONE', *, *, #240, .T. ) ;
#15512=CARTESIAN_POINT ( 'NONE',  ( -24.80114670877659222, 18.00000000000000000, -15.70637264050927051 ) ) ;
#15515=DIRECTION ( 'NONE',  ( -0.000000000000000000, -0.000000000000000000, -1.000000000000000000 ) ) ;
#15516=AXIS2_PLACEMENT_3D ( 'NONE', #3446, #11578, #14239 ) ;
#15520=EDGE_LOOP ( 'NONE', ( #14860, #5211 ) ) ;
#15522=FACE_OUTER_BOUND ( 'NONE', #4312, .T. ) ;
#15523=VECTOR ( 'NONE', #11497, 1000.000000000000000 ) ;
#15525=ADVANCED_FACE ( 'NONE', ( #9468 ), #16303, .F. ) ;
#15529=VECTOR ( 'NONE', #8353, 1000.000000000000000 ) ;
#15531=DIRECTION ( 'NONE',  ( 1.000000000000000000, 0.000000000000000000, 0.000000000000000000 ) ) ;
#15533=CARTESIAN_POINT ( 'NONE',  ( -10.03891356649071653, 19.99999999999999289, -24.87483525495232328 ) ) ;
#15534=ORIENTED_EDGE ( 'NONE', *, *, #7473, .T. ) ;
#15536=FACE_BOUND ( 'NONE', #4174, .T. ) ;
#15537=ORIENTED_EDGE ( 'NONE', *, *, #1922, .F. ) ;
#15539=EDGE_LOOP ( 'NONE', ( #14763, #11146, #6937, #5972 ) ) ;
#15540=CIRCLE ( 'NONE', #11851, 2.500000000000000000 ) ;
#15543=VECTOR ( 'NONE', #14628, 1000.000000000000000 ) ;
#15546=DIRECTION ( 'NONE',  ( -1.000000000000000000, -0.000000000000000000, -0.000000000000000000 ) ) ;
#15552=ADVANCED_FACE ( 'NONE', ( #11066 ), #16746, .T. ) ;
#15553=VERTEX_POINT ( 'NONE', #1775 ) ;
#15556=VECTOR ( 'NONE', #73, 1000.000000000000000 ) ;
#15557=LINE ( 'NONE', #12636, #3663 ) ;
#15558=DIRECTION ( 'NONE',  ( 1.000000000000000000, 0.000000000000000000, -0.000000000000000000 ) ) ;
#15560=CARTESIAN_POINT ( 'NONE',  ( -15.98664213571245440, 31.85373729401663212, -11.16351695777366082 ) ) ;
#15561=LINE ( 'NONE', #11651, #7508 ) ;
#15562=LINE ( 'NONE', #7238, #4812 ) ;
#15565=VECTOR ( 'NONE', #6002, 1000.000000000000000 ) ;
#15566=EDGE_LOOP ( 'NONE', ( #2909, #10959 ) ) ;
#15568=CIRCLE ( 'NONE', #11039, 33.00000000000000000 ) ;
#15570=CARTESIAN_POINT ( 'NONE',  ( 14.79728876016037198, 126.7368160533725643, -7.941237055946955614 ) ) ;
#15574=LINE ( 'NONE', #1047, #16413 ) ;
#15575=CARTESIAN_POINT ( 'NONE',  ( 24.06750934705105749, 197.5381456772451827, -23.52581655030730445 ) ) ;
#15576=EDGE_LOOP ( 'NONE', ( #1997, #14659, #12489, #13878 ) ) ;
#15577=VECTOR ( 'NONE', #12612, 1000.000000000000000 ) ;
#15579=CARTESIAN_POINT ( 'NONE',  ( 22.23358001889399205, 29.90326853444953059, -11.84310668804517697 ) ) ;
#15583=CARTESIAN_POINT ( 'NONE',  ( 34.93420767853316988, 30.00000000000000000, 0.000000000000000000 ) ) ;
#15584=ORIENTED_EDGE ( 'NONE', *, *, #4524, .F. ) ;
#15588=CIRCLE ( 'NONE', #13331, 5.000000000000004441 ) ;
#15589=CARTESIAN_POINT ( 'NONE',  ( 32.50000000000000711, 146.6227766016838245, -16.00000000000000000 ) ) ;
#15592=CARTESIAN_POINT ( 'NONE',  ( 27.99999999999998224, 9.999999999999998224, -35.00200000000000244 ) ) ;
#15595=CYLINDRICAL_SURFACE ( 'NONE', #17496, 2.500000000000000444 ) ;
#15596=EDGE_LOOP ( 'NONE', ( #2114, #11836, #8837, #1072 ) ) ;
#15598=CARTESIAN_POINT ( 'NONE',  ( -27.70723240392776887, 18.00000000000000000, -8.328409877367404235 ) ) ;
#15599=ORIENTED_EDGE ( 'NONE', *, *, #11689, .F. ) ;
#15603=EDGE_LOOP ( 'NONE', ( #6378, #2112 ) ) ;
#15605=DIRECTION ( 'NONE',  ( 0.000000000000000000, 0.000000000000000000, -1.000000000000000000 ) ) ;
#15606=B_SPLINE_CURVE_WITH_KNOTS ( 'NONE', 3,
 ( #6498, #9142, #11890, #14737, #17299, #17480, #9410, #14643, #2516, #6403 ),
 .UNSPECIFIED., .F., .F.,
 ( 4, 2, 2, 2, 4 ),
 ( 1.908195823574487804E-17, 0.002588446031580678066, 0.005176892063161337050, 0.007765338094741995600, 0.01035378412632265502 ),
 .UNSPECIFIED. ) ;
#15607=ADVANCED_FACE ( 'NONE', ( #12490 ), #2611, .F. ) ;
#15610=DIRECTION ( 'NONE',  ( 1.000000000000000000, 0.000000000000000000, -0.000000000000000000 ) ) ;
#15611=ADVANCED_FACE ( 'NONE', ( #6357 ), #11752, .T. ) ;
#15612=ADVANCED_FACE ( 'NONE', ( #1665 ), #11120, .T. ) ;
#15614=CARTESIAN_POINT ( 'NONE',  ( -96.00000000000001421, 171.6227766016838245, 0.000000000000000000 ) ) ;
#15615=CARTESIAN_POINT ( 'NONE',  ( -12.63167751028161589, 20.00000000000000355, -24.35243221814332060 ) ) ;
#15617=CARTESIAN_POINT ( 'NONE',  ( 35.31758992237445938, 193.8375574372276162, -27.04711750382526603 ) ) ;
#15618=FACE_BOUND ( 'NONE', #12983, .T. ) ;
#15619=ORIENTED_EDGE ( 'NONE', *, *, #9482, .F. ) ;
#15620=VERTEX_POINT ( 'NONE', #10049 ) ;
#15622=ORIENTED_EDGE ( 'NONE', *, *, #13957, .T. ) ;
#15623=CARTESIAN_POINT ( 'NONE',  ( -78.82732927925546562, 154.0361450035975395, -27.92332374485730639 ) ) ;
#15625=LINE ( 'NONE', #10141, #8210 ) ;
#15627=CARTESIAN_POINT ( 'NONE',  ( -91.33974596215563224, 136.6227766016838245, 0.000000000000000000 ) ) ;
#15634=CARTESIAN_POINT ( 'NONE',  ( -17.11671918504270451, 32.08177433558115865, -9.477319364664337442 ) ) ;
#15638=EDGE_CURVE ( 'NONE', #7583, #12193, #4585, .T. ) ;
#15639=EDGE_CURVE ( 'NONE', #11894, #11114, #8474, .T. ) ;
#15640=ADVANCED_FACE ( 'NONE', ( #4497 ), #5998, .T. ) ;
#15641=VERTEX_POINT ( 'NONE', #7407 ) ;
#15643=VERTEX_POINT ( 'NONE', #13796 ) ;
#15645=LINE ( 'NONE', #7242, #14419 ) ;
#15647=CARTESIAN_POINT ( 'NONE',  ( 13.91851620013868995, 127.9827558526829563, -9.294367823883964874 ) ) ;
#15648=VERTEX_POINT ( 'NONE', #4409 ) ;
#15651=DIRECTION ( 'NONE',  ( 0.000000000000000000, 0.000000000000000000, 1.000000000000000000 ) ) ;
#15652=CARTESIAN_POINT ( 'NONE',  ( 32.61283963115067053, 202.0279528788176151, -17.33673759440343076 ) ) ;
#15654=ORIENTED_EDGE ( 'NONE', *, *, #16261, .T. ) ;
#15655=CARTESIAN_POINT ( 'NONE',  ( 17.04731744882672828, 19.99999999999885247, -14.80421929169553685 ) ) ;
#15661=EDGE_CURVE ( 'NONE', #9691, #2967, #9794, .T. ) ;
#15670=CARTESIAN_POINT ( 'NONE',  ( 25.00000000000000000, 196.6227766016838245, -12.99999999999999822 ) ) ;
#15671=CARTESIAN_POINT ( 'NONE',  ( 31.77450688729555139, 140.8861252344925106, -16.74142298344134616 ) ) ;
#15672=ORIENTED_EDGE ( 'NONE', *, *, #1387, .T. ) ;
#15673=CARTESIAN_POINT ( 'NONE',  ( 40.00000000000000711, 204.6227766016838245, 2.020667218593133100E-15 ) ) ;
#15678=ORIENTED_EDGE ( 'NONE', *, *, #4273, .F. ) ;
#15682=ORIENTED_EDGE ( 'NONE', *, *, #10954, .F. ) ;
#15684=CARTESIAN_POINT ( 'NONE',  ( 0.000000000000000000, 0.000000000000000000, 0.000000000000000000 ) ) ;
#15685=CARTESIAN_POINT ( 'NONE',  ( -13.49179905494335507, 31.33781166378165395, -13.29076615231557490 ) ) ;
#15686=CARTESIAN_POINT ( 'NONE',  ( -14.94236098988382722, 32.37030496448370798, -9.276599271047366813 ) ) ;
#15687=VECTOR ( 'NONE', #309, 1000.000000000000000 ) ;
#15689=DIRECTION ( 'NONE',  ( 1.000000000000000000, 0.000000000000000000, -0.000000000000000000 ) ) ;
#15690=B_SPLINE_CURVE_WITH_KNOTS ( 'NONE', 3,
 ( #13641, #16394, #4259, #2918, #267, #4339, #15484, #7166 ),
 .UNSPECIFIED., .F., .F.,
 ( 4, 2, 2, 4 ),
 ( 0.01981773175714084123, 0.02208185334846130693, 0.02434597493978176916, 0.02887421812242269709 ),
 .UNSPECIFIED. ) ;
#15691=CARTESIAN_POINT ( 'NONE',  ( -27.70723240392776532, 19.99999999999999289, -8.328409877367407788 ) ) ;
#15693=EDGE_CURVE ( 'NONE', #4419, #4489, #3006, .T. ) ;
#15694=CARTESIAN_POINT ( 'NONE',  ( 24.86101889991104485, 193.5203449394524853, -27.30457132278911558 ) ) ;
#15698=EDGE_LOOP ( 'NONE', ( #2880, #6024, #829, #4461 ) ) ;
#15699=ORIENTED_EDGE ( 'NONE', *, *, #2749, .T. ) ;
#15701=EDGE_CURVE ( 'NONE', #14936, #13466, #3831, .T. ) ;
#15702=EDGE_CURVE ( 'NONE', #11848, #4295, #16535, .T. ) ;
#15703=CARTESIAN_POINT ( 'NONE',  ( -73.19385591260828505, 149.8074533144823590, -24.76648413410753591 ) ) ;
#15705=AXIS2_PLACEMENT_3D ( 'NONE', #4817, #13944, #574 ) ;
#15708=CARTESIAN_POINT ( 'NONE',  ( 13.66341101665266677, 138.6227766016838245, -1.000341871676679184E-14 ) ) ;
#15711=CARTESIAN_POINT ( 'NONE',  ( 24.00000000000000355, 146.6227766016838245, -24.49489742783179480 ) ) ;
#15714=ORIENTED_EDGE ( 'NONE', *, *, #1385, .F. ) ;
#15716=DIRECTION ( 'NONE',  ( 1.000000000000000000, 0.000000000000000000, 0.000000000000000000 ) ) ;
#15726=DIRECTION ( 'NONE',  ( 0.000000000000000000, 0.000000000000000000, 1.000000000000000000 ) ) ;
#15727=CARTESIAN_POINT ( 'NONE',  ( 225.0000000000000000, 89.99999999999997158, -4.999999999999999112 ) ) ;
#15728=VERTEX_POINT ( 'NONE', #600 ) ;
#15731=CIRCLE ( 'NONE', #4709, 20.00000000000000355 ) ;
#15733=AXIS2_PLACEMENT_3D ( 'NONE', #10095, #3020, #7270 ) ;
#15734=DIRECTION ( 'NONE',  ( 0.000000000000000000, 0.000000000000000000, 1.000000000000000000 ) ) ;
#15735=CIRCLE ( 'NONE', #5281, 750.0000000000000000 ) ;
#15737=LINE ( 'NONE', #10167, #12273 ) ;
#15738=AXIS2_PLACEMENT_3D ( 'NONE', #6818, #12211, #80 ) ;
#15741=CARTESIAN_POINT ( 'NONE',  ( 48.00000000000000711, 151.6227766016839098, -8.071800142134973655 ) ) ;
#15742=EDGE_CURVE ( 'NONE', #9093, #489, #1856, .T. ) ;
#15743=DIRECTION ( 'NONE',  ( -1.000000000000000000, -0.000000000000000000, -0.000000000000000000 ) ) ;
#15744=CARTESIAN_POINT ( 'NONE',  ( 24.00862450121832126, 196.9927911392394151, -24.11293157882131410 ) ) ;
#15747=CARTESIAN_POINT ( 'NONE',  ( 15.58496356726128873, 29.99118438505512430, -15.00000000000000000 ) ) ;
#15750=ORIENTED_EDGE ( 'NONE', *, *, #10951, .F. ) ;
#15752=CARTESIAN_POINT ( 'NONE',  ( -86.00000000000002842, 146.6227766016838245, -35.00000000000000000 ) ) ;
#15754=CARTESIAN_POINT ( 'NONE',  ( 13.64704021889961361, 139.0043329719002259, -8.527746218696755420 ) ) ;
#15755=ORIENTED_EDGE ( 'NONE', *, *, #6132, .F. ) ;
#15757=CYLINDRICAL_SURFACE ( 'NONE', #16365, 2.500000000000000444 ) ;
#15766=EDGE_CURVE ( 'NONE', #16968, #7898, #3547, .T. ) ;
#15767=EDGE_CURVE ( 'NONE', #7515, #15447, #10604, .T. ) ;
#15768=DIRECTION ( 'NONE',  ( -0.000000000000000000, -0.000000000000000000, 1.000000000000000000 ) ) ;
#15769=VERTEX_POINT ( 'NONE', #17047 ) ;
#15776=CARTESIAN_POINT ( 'NONE',  ( -20.49999999999998224, 10.00000000000000000, -13.00000000000000000 ) ) ;
#15782=CARTESIAN_POINT ( 'NONE',  ( 28.54584381417872763, 189.2596037578064738, -27.89172594985640075 ) ) ;
#15784=CARTESIAN_POINT ( 'NONE',  ( -12.80328004468503167, 17.99999999998165734, -5.290760321145399736 ) ) ;
#15790=VECTOR ( 'NONE', #17065, 1000.000000000000000 ) ;
#15791=CARTESIAN_POINT ( 'NONE',  ( 34.93420767853316988, 18.00000000000000355, 0.000000000000000000 ) ) ;
#15792=ORIENTED_EDGE ( 'NONE', *, *, #7490, .F. ) ;
#15794=ORIENTED_EDGE ( 'NONE', *, *, #10336, .T. ) ;
#15796=CARTESIAN_POINT ( 'NONE',  ( -79.40013309498280591, 154.1043103600818256, -27.96613953460096624 ) ) ;
#15805=CARTESIAN_POINT ( 'NONE',  ( 27.78002739833986112, 152.2013812635046008, -29.11730325185375534 ) ) ;
#15806=LINE ( 'NONE', #13067, #185 ) ;
#15810=FACE_OUTER_BOUND ( 'NONE', #6401, .T. ) ;
#15811=DIRECTION ( 'NONE',  ( -0.000000000000000000, -0.000000000000000000, -1.000000000000000000 ) ) ;
#15822=LINE ( 'NONE', #14674, #11834 ) ;
#15823=ORIENTED_EDGE ( 'NONE', *, *, #13939, .T. ) ;
#15825=CARTESIAN_POINT ( 'NONE',  ( 225.0000000000000000, 89.99999999999997158, -4.999999999999999112 ) ) ;
#15826=AXIS2_PLACEMENT_3D ( 'NONE', #10062, #8748, #3436 ) ;
#15830=CARTESIAN_POINT ( 'NONE',  ( 30.00000000000000355, 196.6227766016838245, 0.000000000000000000 ) ) ;
#15834=DIRECTION ( 'NONE',  ( 1.000000000000000000, 0.000000000000000000, 0.000000000000000000 ) ) ;
#15840=ORIENTED_EDGE ( 'NONE', *, *, #7681, .F. ) ;
#15842=VECTOR ( 'NONE', #16406, 1000.000000000000000 ) ;
#15844=CARTESIAN_POINT ( 'NONE',  ( 13.88882648224844907, 138.0291231684843751, -11.40862608215692831 ) ) ;
#15846=CARTESIAN_POINT ( 'NONE',  ( -85.89531307607238375, 147.7508872708765750, -25.59654897292657694 ) ) ;
#15847=AXIS2_PLACEMENT_3D ( 'NONE', #7057, #8111, #12459 ) ;
#15848=CARTESIAN_POINT ( 'NONE',  ( 10.61972500670372277, 131.6239249143206393, -11.92364046234351527 ) ) ;
#15849=VERTEX_POINT ( 'NONE', #3765 ) ;
#15851=CARTESIAN_POINT ( 'NONE',  ( 49.99999999999998579, 159.6227766016838814, -8.071800142134975431 ) ) ;
#15852=LINE ( 'NONE', #3903, #852 ) ;
#15853=CARTESIAN_POINT ( 'NONE',  ( 24.40218896425084338, 201.6348411963793126, -13.74530841833676220 ) ) ;
#15861=ORIENTED_EDGE ( 'NONE', *, *, #4335, .F. ) ;
#15862=CARTESIAN_POINT ( 'NONE',  ( -27.98221281347036893, 30.00000000000000355, -4.999999999999999112 ) ) ;
#15863=LINE ( 'NONE', #16043, #10069 ) ;
#15865=VERTEX_POINT ( 'NONE', #936 ) ;
#15866=CARTESIAN_POINT ( 'NONE',  ( 50.00000000000000000, 196.6227766016838245, 0.000000000000000000 ) ) ;
#15868=VECTOR ( 'NONE', #11447, 1000.000000000000000 ) ;
#15871=LINE ( 'NONE', #2599, #561 ) ;
#15873=ORIENTED_EDGE ( 'NONE', *, *, #15034, .F. ) ;
#15875=CARTESIAN_POINT ( 'NONE',  ( 23.65095110843940063, 192.6231533511310943, -25.45681811525070870 ) ) ;
#15876=CARTESIAN_POINT ( 'NONE',  ( -13.77790586189935951, 31.39781009804136502, -13.10675149387370197 ) ) ;
#15877=CARTESIAN_POINT ( 'NONE',  ( -11.99122994684827503, 18.00000000000000000, -24.50500383881282573 ) ) ;
#15879=CARTESIAN_POINT ( 'NONE',  ( -15.00000000000001421, 130.0000000000000000, -13.00000000000000000 ) ) ;
#15881=CARTESIAN_POINT ( 'NONE',  ( 27.79815362222807806, 191.0369151440704343, -29.12214185324409854 ) ) ;
#15883=VERTEX_POINT ( 'NONE', #1286 ) ;
#15884=ORIENTED_EDGE ( 'NONE', *, *, #11547, .T. ) ;
#15885=EDGE_LOOP ( 'NONE', ( #16762, #13018, #5172, #5607, #17141, #16744, #14572, #2435, #6123 ) ) ;
#15887=CARTESIAN_POINT ( 'NONE',  ( 196.0000000000000000, 159.6227766016838814, -8.071800142134975431 ) ) ;
#15893=DIRECTION ( 'NONE',  ( -1.000000000000000000, 0.000000000000000000, 0.000000000000000000 ) ) ;
#15896=EDGE_LOOP ( 'NONE', ( #5841, #203, #17432, #988 ) ) ;
#15898=CARTESIAN_POINT ( 'NONE',  ( 22.23780067492955936, 29.90321370453013117, -11.83858959072850858 ) ) ;
#15901=PLANE ( 'NONE',  #10986 ) ;
#15902=ORIENTED_EDGE ( 'NONE', *, *, #4283, .T. ) ;
#15905=LINE ( 'NONE', #14575, #5388 ) ;
#15906=EDGE_LOOP ( 'NONE', ( #7770, #12534, #8944, #16745 ) ) ;
#15907=FACE_BOUND ( 'NONE', #12744, .T. ) ;
#15912=DIRECTION ( 'NONE',  ( 1.000000000000000000, 6.217248937900877415E-15, 0.000000000000000000 ) ) ;
#15913=CARTESIAN_POINT ( 'NONE',  ( -75.00938694728593248, 143.2738031352136829, -20.53261660472919559 ) ) ;
#15914=DIRECTION ( 'NONE',  ( -1.000000000000000000, -0.000000000000000000, 0.000000000000000000 ) ) ;
#15920=VERTEX_POINT ( 'NONE', #6867 ) ;
#15921=EDGE_CURVE ( 'NONE', #5946, #11995, #16345, .T. ) ;
#15922=VERTEX_POINT ( 'NONE', #15002 ) ;
#15925=PLANE ( 'NONE',  #16600 ) ;
#15926=CARTESIAN_POINT ( 'NONE',  ( 9.276452510677492214, 132.6951329324795381, -12.46699917133672741 ) ) ;
#15927=EDGE_CURVE ( 'NONE', #11033, #16523, #5533, .T. ) ;
#15932=ADVANCED_FACE ( 'NONE', ( #15979 ), #7927, .F. ) ;
#15933=CARTESIAN_POINT ( 'NONE',  ( 22.49999999999999645, 197.1893936856111793, -20.88304578468305905 ) ) ;
#15940=CARTESIAN_POINT ( 'NONE',  ( -68.00000000000000000, 191.6227766016837961, 1.224646799147353454E-15 ) ) ;
#15943=CARTESIAN_POINT ( 'NONE',  ( 12.53348921593948972, 131.0729685438566605, -13.11561688552428784 ) ) ;
#15945=DIRECTION ( 'NONE',  ( 1.000000000000000000, 0.000000000000000000, 0.000000000000000000 ) ) ;
#15946=CARTESIAN_POINT ( 'NONE',  ( -21.35874126517689220, 18.00000000000000355, -19.71585776365615317 ) ) ;
#15947=ORIENTED_EDGE ( 'NONE', *, *, #13803, .F. ) ;
#15948=LINE ( 'NONE', #3824, #3795 ) ;
#15950=ORIENTED_EDGE ( 'NONE', *, *, #7693, .T. ) ;
#15953=ORIENTED_EDGE ( 'NONE', *, *, #1918, .T. ) ;
#15956=CARTESIAN_POINT ( 'NONE',  ( 28.82732927925544431, 189.2094081997701096, -27.92332374485732061 ) ) ;
#15957=LINE ( 'NONE', #8250, #10488 ) ;
#15958=CARTESIAN_POINT ( 'NONE',  ( -16.24840885328083928, 32.75254598042347709, -6.058899415740283345 ) ) ;
#15959=ORIENTED_EDGE ( 'NONE', *, *, #497, .T. ) ;
#15961=EDGE_CURVE ( 'NONE', #489, #9093, #12275, .T. ) ;
#15964=CARTESIAN_POINT ( 'NONE',  ( 30.23477484661547621, 190.6230697630494433, -29.39368741583861322 ) ) ;
#15969=ORIENTED_EDGE ( 'NONE', *, *, #13623, .F. ) ;
#15972=VERTEX_POINT ( 'NONE', #300 ) ;
#15974=FACE_OUTER_BOUND ( 'NONE', #1971, .T. ) ;
#15975=LINE ( 'NONE', #17215, #6095 ) ;
#15976=AXIS2_PLACEMENT_3D ( 'NONE', #8023, #14766, #2639 ) ;
#15979=FACE_OUTER_BOUND ( 'NONE', #16938, .T. ) ;
#15982=CARTESIAN_POINT ( 'NONE',  ( 24.41053355130577884, 29.87514852601161763, -8.212591972297857978 ) ) ;
#15983=EDGE_CURVE ( 'NONE', #12777, #17253, #10856, .T. ) ;
#15984=EDGE_CURVE ( 'NONE', #10334, #11543, #2949, .T. ) ;
#15986=ADVANCED_FACE ( 'NONE', ( #5705 ), #12431, .F. ) ;
#15987=DIRECTION ( 'NONE',  ( 1.000000000000000000, 0.000000000000000000, 0.000000000000000000 ) ) ;
#15989=ORIENTED_EDGE ( 'NONE', *, *, #2779, .T. ) ;
#15992=AXIS2_PLACEMENT_3D ( 'NONE', #8561, #16373, #12550 ) ;
#15993=ORIENTED_EDGE ( 'NONE', *, *, #14418, .F. ) ;
#16000=ADVANCED_FACE ( 'NONE', ( #2633 ), #2948, .F. ) ;
#16004=ORIENTED_EDGE ( 'NONE', *, *, #10059, .F. ) ;
#16008=DIRECTION ( 'NONE',  ( -1.000000000000000000, -0.000000000000000000, -0.000000000000000000 ) ) ;
#16010=CARTESIAN_POINT ( 'NONE',  ( 36.00000000000000711, 196.6227766016838245, -24.49489742783179125 ) ) ;
#16011=VECTOR ( 'NONE', #12289, 1000.000000000000000 ) ;
#16015=B_SPLINE_CURVE_WITH_KNOTS ( 'NONE', 3,
 ( #922, #7911, #17034, #7817, #3751, #6310, #15617, #8969, #4827, #9141, #2418, #6237, #10378, #14288, #2248, #11797, #4901, #13224, #15964, #5168, #14545, #7722, #10217, #13056, #11630, #15881, #16959, #13132, #9233, #3492, #10290, #3671, #14465, #1000, #15694, #1095, #7641, #6497, #11889, #11703, #3844, #6149, #14380, #17203 ),
 .UNSPECIFIED., .F., .F.,
 ( 4, 2, 2, 2, 2, 2, 2, 2, 2, 2, 2, 2, 2, 2, 2, 2, 2, 2, 2, 2, 2, 4 ),
 ( 0.000000000000000000, 0.002715240924237344918, 0.003394051155296696869, 0.004072861386356049253, 0.005430481848474700245, 0.006788102310593352971, 0.008145722772712003096, 0.009503343234830655822, 0.01018215346588999259, 0.01086096369694932937, 0.01153977392800866614, 0.01221858415906799944, 0.01289739439012733795, 0.01357620462118667472, 0.01493382508330533785, 0.01629144554542400272, 0.01697025577648333602, 0.01764906600754266586, 0.01900668646966133246, 0.01968549670072063801, 0.02036430693177994009, 0.02172192739389855118 ),
 .UNSPECIFIED. ) ;
#16017=CARTESIAN_POINT ( 'NONE',  ( -81.58454895572883458, 152.4141840272156116, -29.25805444611330586 ) ) ;
#16018=CARTESIAN_POINT ( 'NONE',  ( 13.23724818701971984, 139.1606502921264905, -9.139539437136660283 ) ) ;
#16021=CARTESIAN_POINT ( 'NONE',  ( -43.00000000000000000, 144.1839557653416080, -18.33333333333335702 ) ) ;
#16022=CIRCLE ( 'NONE', #8103, 7.500000000000020428 ) ;
#16024=CARTESIAN_POINT ( 'NONE',  ( -3.000000000000000888, 171.6227766016838245, 0.000000000000000000 ) ) ;
#16025=DIRECTION ( 'NONE',  ( -0.000000000000000000, -0.000000000000000000, -1.000000000000000000 ) ) ;
#16027=CARTESIAN_POINT ( 'NONE',  ( 30.00000000000001066, 146.6227766016838245, -13.00000000000000000 ) ) ;
#16028=CARTESIAN_POINT ( 'NONE',  ( 21.54590827305403877, 18.00000000000000000, -9.735228713654757726 ) ) ;
#16030=DIRECTION ( 'NONE',  ( 1.000000000000000000, 1.156482317317868274E-16, 0.000000000000000000 ) ) ;
#16033=ORIENTED_EDGE ( 'NONE', *, *, #9107, .F. ) ;
#16034=CARTESIAN_POINT ( 'NONE',  ( 7.674484246658608733, 133.8653086123773903, -14.91481465347803415 ) ) ;
#16036=VECTOR ( 'NONE', #13719, 1000.000000000000000 ) ;
#16037=ORIENTED_EDGE ( 'NONE', *, *, #9137, .F. ) ;
#16038=EDGE_CURVE ( 'NONE', #11342, #8547, #379, .T. ) ;
#16039=LINE ( 'NONE', #10724, #3665 ) ;
#16040=EDGE_CURVE ( 'NONE', #12106, #7374, #4291, .T. ) ;
#16043=CARTESIAN_POINT ( 'NONE',  ( -75.00000000000002842, 146.6227766016838245, -35.00200000000000244 ) ) ;
#16047=EDGE_CURVE ( 'NONE', #10334, #15865, #13425, .T. ) ;
#16052=PRODUCT_DEFINITION_FORMATION_WITH_SPECIFIED_SOURCE ( 'ANY', '', #7438, .NOT_KNOWN. ) ;
#16053=DIRECTION ( 'NONE',  ( 1.000000000000000000, 0.000000000000000000, -0.000000000000000000 ) ) ;
#16054=CIRCLE ( 'NONE', #15198, 2.499999999999998668 ) ;
#16055=CARTESIAN_POINT ( 'NONE',  ( 32.26120111208032171, 189.4484344766680692, -27.77174765869275319 ) ) ;
#16056=DIRECTION ( 'NONE',  ( 0.000000000000000000, 1.000000000000000000, 0.000000000000000000 ) ) ;
#16057=CARTESIAN_POINT ( 'NONE',  ( -9.925381735234191538, 18.00000000000231992, -11.63955885304398130 ) ) ;
#16058=VERTEX_POINT ( 'NONE', #11005 ) ;
#16061=CARTESIAN_POINT ( 'NONE',  ( -84.26947555605805462, 190.4340272497385342, -27.11642929875283414 ) ) ;
#16062=CARTESIAN_POINT ( 'NONE',  ( -7.379000772444994638, 20.00000000000000000, -25.00000000000000000 ) ) ;
#16063=EDGE_CURVE ( 'NONE', #11263, #2271, #7029, .T. ) ;
#16064=EDGE_LOOP ( 'NONE', ( #17111, #13665 ) ) ;
#16065=CIRCLE ( 'NONE', #799, 2.500000000000002220 ) ;
#16066=ORIENTED_EDGE ( 'NONE', *, *, #9868, .F. ) ;
#16067=ORIENTED_EDGE ( 'NONE', *, *, #14606, .F. ) ;
#16071=ORIENTED_EDGE ( 'NONE', *, *, #3325, .F. ) ;
#16074=CARTESIAN_POINT ( 'NONE',  ( 13.63270490666629975, 138.8028880870465969, -3.449993069226409581 ) ) ;
#16076=CARTESIAN_POINT ( 'NONE',  ( 32.98178886359406903, 151.8338245663404393, -28.86895077895843897 ) ) ;
#16084=CARTESIAN_POINT ( 'NONE',  ( 24.67988836892261872, 29.87169161469932277, -7.267893787782148785 ) ) ;
#16085=CARTESIAN_POINT ( 'NONE',  ( 15.00000000000000000, 143.0344144757318929, -16.50549856913627877 ) ) ;
#16089=LINE ( 'NONE', #1121, #998 ) ;
#16091=CIRCLE ( 'NONE', #5916, 2.500000000000000444 ) ;
#16097=EDGE_LOOP ( 'NONE', ( #13558, #14885, #5999, #9844 ) ) ;
#16099=EDGE_CURVE ( 'NONE', #8531, #17520, #15159, .T. ) ;
#16100=LINE ( 'NONE', #5290, #5087 ) ;
#16101=EDGE_CURVE ( 'NONE', #7175, #17476, #15256, .T. ) ;
#16102=CARTESIAN_POINT ( 'NONE',  ( 20.42763382733058108, 18.00000000000000000, -24.23318166603144164 ) ) ;
#16105=EDGE_CURVE ( 'NONE', #1310, #11867, #8597, .T. ) ;
#16112=DIRECTION ( 'NONE',  ( -0.000000000000000000, -0.000000000000000000, -1.000000000000000000 ) ) ;
#16116=ORIENTED_EDGE ( 'NONE', *, *, #16261, .F. ) ;
#16117=CARTESIAN_POINT ( 'NONE',  ( 10.45945364060320237, 139.0001874602887995, -13.88305366436908272 ) ) ;
#16118=ORIENTED_EDGE ( 'NONE', *, *, #3707, .T. ) ;
#16119=CARTESIAN_POINT ( 'NONE',  ( -85.72918267991042285, 148.4136790374692509, -26.19897850971620912 ) ) ;
#16120=CARTESIAN_POINT ( 'NONE',  ( 10.22516481506617581, 140.0471213951830407, -11.75777818883246617 ) ) ;
#16123=CARTESIAN_POINT ( 'NONE',  ( -15.00000000000001421, 20.00000000000004263, -4.999999999999999112 ) ) ;
#16128=CARTESIAN_POINT ( 'NONE',  ( 20.13757169487763576, 18.00000000000000000, -24.32197800972832624 ) ) ;
#16129=CARTESIAN_POINT ( 'NONE',  ( 32.29171157743327569, 18.00000000000000000, -15.02090973096405158 ) ) ;
#16130=CARTESIAN_POINT ( 'NONE',  ( -3.000000000000002665, 134.2062027339443944, -25.00000000000000000 ) ) ;
#16132=CARTESIAN_POINT ( 'NONE',  ( 49.99999999999998579, 187.6227766016837961, -12.50000337241049309 ) ) ;
#16133=DIRECTION ( 'NONE',  ( 0.000000000000000000, 0.000000000000000000, -1.000000000000000000 ) ) ;
#16136=VECTOR ( 'NONE', #10053, 1000.000000000000000 ) ;
#16142=ADVANCED_FACE ( 'NONE', ( #16939 ), #3397, .F. ) ;
#16148=ORIENTED_EDGE ( 'NONE', *, *, #16099, .F. ) ;
#16150=DIRECTION ( 'NONE',  ( 1.000000000000000000, 0.000000000000000000, -0.000000000000000000 ) ) ;
#16153=DIRECTION ( 'NONE',  ( 0.000000000000000000, 0.000000000000000000, 1.000000000000000000 ) ) ;
#16157=CARTESIAN_POINT ( 'NONE',  ( -82.81385839426211248, 189.6648409365396333, -27.63145166803556663 ) ) ;
#16160=ORIENTED_EDGE ( 'NONE', *, *, #14638, .F. ) ;
#16168=EDGE_CURVE ( 'NONE', #4330, #8060, #4088, .T. ) ;
#16169=CYLINDRICAL_SURFACE ( 'NONE', #166, 2.499999999999998668 ) ;
#16170=EDGE_CURVE ( 'NONE', #17487, #8812, #6329, .T. ) ;
#16171=CARTESIAN_POINT ( 'NONE',  ( 22.93524650466160963, 29.84210526315773748, -4.999999999999999112 ) ) ;
#16175=ORIENTED_EDGE ( 'NONE', *, *, #15485, .F. ) ;
#16177=CARTESIAN_POINT ( 'NONE',  ( 21.54624641763228254, 29.91220938647573391, -12.53033468027509478 ) ) ;
#16179=DIRECTION ( 'NONE',  ( 0.000000000000000000, 0.000000000000000000, 1.000000000000000000 ) ) ;
#16181=CARTESIAN_POINT ( 'NONE',  ( -86.65543510501046853, 143.1309386941324817, -16.67123533649923317 ) ) ;
#16183=DIRECTION ( 'NONE',  ( -1.000000000000000000, -0.000000000000000000, 0.000000000000000000 ) ) ;
#16184=VERTEX_POINT ( 'NONE', #15427 ) ;
#16187=SURFACE_STYLE_USAGE ( .BOTH. , #16362 ) ;
#16188=DIRECTION ( 'NONE',  ( 1.000000000000000000, 0.000000000000000000, 0.000000000000000000 ) ) ;
#16189=DIRECTION ( 'NONE',  ( 0.000000000000000000, 1.387778780781445676E-14, 1.000000000000000000 ) ) ;
#16190=CARTESIAN_POINT ( 'NONE',  ( -75.21194266656338812, 142.9896906294144969, -20.13387259562454190 ) ) ;
#16197=DIRECTION ( 'NONE',  ( 1.000000000000000000, 0.000000000000000000, -0.000000000000000000 ) ) ;
#16204=CARTESIAN_POINT ( 'NONE',  ( -75.98251204892453359, 151.0988115558745051, -28.35253695364550097 ) ) ;
#16210=DIRECTION ( 'NONE',  ( -1.000000000000000000, -0.000000000000000000, 0.000000000000000000 ) ) ;
#16212=CARTESIAN_POINT ( 'NONE',  ( 20.21973759693270267, 29.89473369120481294, -11.02800485953945930 ) ) ;
#16214=DIRECTION ( 'NONE',  ( -0.000000000000000000, -0.000000000000000000, 1.000000000000000000 ) ) ;
#16215=DIRECTION ( 'NONE',  ( 0.000000000000000000, 0.000000000000000000, 1.000000000000000000 ) ) ;
#16225=DIRECTION ( 'NONE',  ( -0.000000000000000000, -0.000000000000000000, -1.000000000000000000 ) ) ;
#16227=ORIENTED_EDGE ( 'NONE', *, *, #6019, .T. ) ;
#16229=ORIENTED_EDGE ( 'NONE', *, *, #1278, .T. ) ;
#16231=CARTESIAN_POINT ( 'NONE',  ( 36.35693927557340999, 192.6156044230849034, -25.46745035168473947 ) ) ;
#16233=DIRECTION ( 'NONE',  ( 0.000000000000000000, 0.8660254037844413721, 0.4999999999999952816 ) ) ;
#16234=ADVANCED_FACE ( 'NONE', ( #17281 ), #9396, .F. ) ;
#16235=ORIENTED_EDGE ( 'NONE', *, *, #4147, .T. ) ;
#16237=ORIENTED_EDGE ( 'NONE', *, *, #16101, .T. ) ;
#16238=CARTESIAN_POINT ( 'NONE',  ( -82.00760546193471612, 189.3908747183072592, -27.80828541846620183 ) ) ;
#16240=ORIENTED_EDGE ( 'NONE', *, *, #13000, .F. ) ;
#16241=ORIENTED_EDGE ( 'NONE', *, *, #12281, .F. ) ;
#16244=VECTOR ( 'NONE', #16684, 1000.000000000000000 ) ;
#16254=VECTOR ( 'NONE', #16836, 1000.000000000000000 ) ;
#16256=CARTESIAN_POINT ( 'NONE',  ( -85.83427352782426567, 198.0686797691926415, -22.93241811017416154 ) ) ;
#16258=DIRECTION ( 'NONE',  ( -1.000000000000000000, 0.000000000000000000, 0.000000000000000000 ) ) ;
#16261=EDGE_CURVE ( 'NONE', #102, #10869, #1535, .T. ) ;
#16263=DIRECTION ( 'NONE',  ( -0.8660254037844378194, -0.5000000000000015543, -0.000000000000000000 ) ) ;
#16264=ORIENTED_EDGE ( 'NONE', *, *, #11617, .T. ) ;
#16265=CARTESIAN_POINT ( 'NONE',  ( -70.00000000000000000, 171.6227766016838245, 0.000000000000000000 ) ) ;
#16267=VERTEX_POINT ( 'NONE', #1079 ) ;
#16271=DIRECTION ( 'NONE',  ( 8.673617379884037937E-17, 0.000000000000000000, 1.000000000000000000 ) ) ;
#16275=DIRECTION ( 'NONE',  ( 0.000000000000000000, -0.8660254037844413721, -0.4999999999999953371 ) ) ;
#16276=DIRECTION ( 'NONE',  ( -0.000000000000000000, -0.000000000000000000, 1.000000000000000000 ) ) ;
#16280=VECTOR ( 'NONE', #16628, 1000.000000000000000 ) ;
#16281=CARTESIAN_POINT ( 'NONE',  ( 15.33542211484438056, 137.4551579351490318, -9.454295640945616697 ) ) ;
#16282=VERTEX_POINT ( 'NONE', #11963 ) ;
#16283=DIRECTION ( 'NONE',  ( 0.000000000000000000, 0.000000000000000000, 1.000000000000000000 ) ) ;
#16284=LINE ( 'NONE', #2826, #12317 ) ;
#16285=VERTEX_POINT ( 'NONE', #15866 ) ;
#16286=DIRECTION ( 'NONE',  ( -1.000000000000000000, -0.000000000000000000, -0.000000000000000000 ) ) ;
#16288=CIRCLE ( 'NONE', #1008, 10.00000000000000178 ) ;
#16290=EDGE_CURVE ( 'NONE', #14342, #209, #15948, .T. ) ;
#16293=CARTESIAN_POINT ( 'NONE',  ( 34.93420767853314146, 18.00000000000000355, -6.320602137672510779 ) ) ;
#16294=CARTESIAN_POINT ( 'NONE',  ( 17.77234289100693232, 17.99999999999999289, -12.54415977683811256 ) ) ;
#16296=DIRECTION ( 'NONE',  ( -1.156482317317868274E-16, 1.000000000000000000, 0.000000000000000000 ) ) ;
#16297=DIRECTION ( 'NONE',  ( 1.000000000000000000, 0.000000000000000000, -0.000000000000000000 ) ) ;
#16299=B_SPLINE_CURVE_WITH_KNOTS ( 'NONE', 3,
 ( #13098, #3797, #10608, #15846, #6636, #9376, #16119, #14693, #14778, #9193, #7868, #10433, #14598, #2474, #2573, #5308, #9020, #13363, #13279, #7960, #3720, #1146, #16017, #6549, #12029, #2650, #8041, #13449, #1320, #11940, #17342, #14434, #2298, #964, #16465, #16204, #13710, #12473, #12125, #340, #8130, #5479, #1676, #13631 ),
 .UNSPECIFIED., .F., .F.,
 ( 4, 2, 2, 2, 2, 2, 2, 2, 2, 2, 2, 2, 2, 2, 2, 2, 2, 2, 2, 2, 2, 4 ),
 ( 0.02539562174428233732, 0.02674754696500270326, 0.02742350957536288450, 0.02809947218572306574, 0.02945139740644348719, 0.03012736001680369619, 0.03080332262716390171, 0.03215524784788428847, 0.03283121045824447665, 0.03350717306860466482, 0.03418313567896484606, 0.03485909828932503424, 0.03621102351004540365, 0.03688698612040561264, 0.03756294873076582164, 0.03891487395148625350, 0.03959083656184648331, 0.04026679917220671312, 0.04161872439292722825, 0.04297064961364774338, 0.04432257483436825851, 0.04702642527580928183 ),
 .UNSPECIFIED. ) ;
#16301=CARTESIAN_POINT ( 'NONE',  ( 27.99999999999998224, 9.999999999999998224, -30.00000000000001066 ) ) ;
#16302=ORIENTED_EDGE ( 'NONE', *, *, #3440, .F. ) ;
#16303=CYLINDRICAL_SURFACE ( 'NONE', #8343, 2.500000000000000444 ) ;
#16304=AXIS2_PLACEMENT_3D ( 'NONE', #9990, #12757, #3191 ) ;
#16305=AXIS2_PLACEMENT_3D ( 'NONE', #16754, #15410, #4705 ) ;
#16307=AXIS2_PLACEMENT_3D ( 'NONE', #9456, #16025, #9382 ) ;
#16309=CARTESIAN_POINT ( 'NONE',  ( 15.00000000000000000, 204.6227766016838245, 2.020667218593133100E-15 ) ) ;
#16310=AXIS2_PLACEMENT_3D ( 'NONE', #7356, #4789, #7264 ) ;
#16311=CARTESIAN_POINT ( 'NONE',  ( -5.000000000000004441, 144.1839557653416080, -18.33333333333336057 ) ) ;
#16313=CARTESIAN_POINT ( 'NONE',  ( 29.43652167955699994, 154.1240291517870276, -27.97845313684488033 ) ) ;
#16319=AXIS2_PLACEMENT_3D ( 'NONE', #4165, #4255, #10801 ) ;
#16320=FACE_OUTER_BOUND ( 'NONE', #2159, .T. ) ;
#16324=FACE_OUTER_BOUND ( 'NONE', #5758, .T. ) ;
#16326=VECTOR ( 'NONE', #3630, 1000.000000000000000 ) ;
#16327=ORIENTED_EDGE ( 'NONE', *, *, #9482, .T. ) ;
#16329=VERTEX_POINT ( 'NONE', #6838 ) ;
#16334=ORIENTED_EDGE ( 'NONE', *, *, #15961, .T. ) ;
#16336=CIRCLE ( 'NONE', #1054, 2.500000000000000444 ) ;
#16338=AXIS2_PLACEMENT_3D ( 'NONE', #8998, #6336, #1209 ) ;
#16339=VERTEX_POINT ( 'NONE', #16309 ) ;
#16343=CARTESIAN_POINT ( 'NONE',  ( -23.00000000000000000, 122.0000000000000284, 0.000000000000000000 ) ) ;
#16344=FACE_OUTER_BOUND ( 'NONE', #7689, .T. ) ;
#16345=LINE ( 'NONE', #12260, #5536 ) ;
#16348=CARTESIAN_POINT ( 'NONE',  ( -77.58098289114030877, 202.1180966153993097, -17.17743398583135672 ) ) ;
#16351=CARTESIAN_POINT ( 'NONE',  ( 34.93420767853316988, 20.00000000000000000, -4.999999999999999112 ) ) ;
#16352=DIRECTION ( 'NONE',  ( 1.000000000000000000, 0.000000000000000000, 0.000000000000000000 ) ) ;
#16354=AXIS2_PLACEMENT_3D ( 'NONE', #9109, #6731, #1060 ) ;
#16356=DIRECTION ( 'NONE',  ( 0.000000000000000000, 0.000000000000000000, 1.000000000000000000 ) ) ;
#16362=SURFACE_SIDE_STYLE ('',( #3779 ) ) ;
#16365=AXIS2_PLACEMENT_3D ( 'NONE', #1726, #9029, #8533 ) ;
#16366=CARTESIAN_POINT ( 'NONE',  ( 0.000000000000000000, 20.00000000000000000, 0.000000000000000000 ) ) ;
#16369=ORIENTED_EDGE ( 'NONE', *, *, #4762, .F. ) ;
#16370=DIRECTION ( 'NONE',  ( -1.000000000000000000, 0.000000000000000000, 0.000000000000000000 ) ) ;
#16371=CARTESIAN_POINT ( 'NONE',  ( -70.00000000000000000, 154.3022685259950038, -9.999999999999900524 ) ) ;
#16372=CYLINDRICAL_SURFACE ( 'NONE', #11038, 5.000000000000018652 ) ;
#16373=DIRECTION ( 'NONE',  ( -0.000000000000000000, -0.000000000000000000, 1.000000000000000000 ) ) ;
#16376=CARTESIAN_POINT ( 'NONE',  ( 16.30283403932978459, 136.8379281265527254, -4.993081733805620814 ) ) ;
#16379=DIRECTION ( 'NONE',  ( 0.000000000000000000, 1.000000000000000000, 0.000000000000000000 ) ) ;
#16380=DIRECTION ( 'NONE',  ( 1.000000000000000000, 0.000000000000000000, 0.000000000000000000 ) ) ;
#16387=VECTOR ( 'NONE', #584, 1000.000000000000000 ) ;
#16389=EDGE_CURVE ( 'NONE', #13669, #8380, #158, .T. ) ;
#16392=EDGE_CURVE ( 'NONE', #7907, #14433, #4162, .T. ) ;
#16393=CARTESIAN_POINT ( 'NONE',  ( -45.00000000000000000, 134.2062027339443944, -15.00000000000000000 ) ) ;
#16394=CARTESIAN_POINT ( 'NONE',  ( 14.29542716350633214, 143.4273548044023698, -17.14909632368674508 ) ) ;
#16396=EDGE_LOOP ( 'NONE', ( #1499, #1624 ) ) ;
#16399=CARTESIAN_POINT ( 'NONE',  ( 24.99836435517920918, 19.99999999999999289, -6.327826241642252825 ) ) ;
#16400=AXIS2_PLACEMENT_3D ( 'NONE', #13442, #6812, #7761 ) ;
#16401=CARTESIAN_POINT ( 'NONE',  ( 15.00000000000000000, 143.0344144757318929, -16.50549856913627877 ) ) ;
#16406=DIRECTION ( 'NONE',  ( -0.000000000000000000, -0.000000000000000000, 1.000000000000000000 ) ) ;
#16407=VERTEX_POINT ( 'NONE', #8587 ) ;
#16408=CARTESIAN_POINT ( 'NONE',  ( 37.50000000000000711, 146.6227766016838245, -21.54065922853802562 ) ) ;
#16409=ORIENTED_EDGE ( 'NONE', *, *, #5277, .T. ) ;
#16411=CARTESIAN_POINT ( 'NONE',  ( 17.00000000000000000, 171.6227766016838245, 0.000000000000000000 ) ) ;
#16413=VECTOR ( 'NONE', #3788, 1000.000000000000000 ) ;
#16419=CARTESIAN_POINT ( 'NONE',  ( 19.49215236471922807, 140.4173771131980857, -15.85404464849102268 ) ) ;
#16420=ORIENTED_EDGE ( 'NONE', *, *, #12512, .T. ) ;
#16421=CARTESIAN_POINT ( 'NONE',  ( -77.73879888791972803, 189.4484344766680977, -27.77174765869276030 ) ) ;
#16426=ADVANCED_FACE ( 'NONE', ( #15494, #2042 ), #17003, .F. ) ;
#16429=ORIENTED_EDGE ( 'NONE', *, *, #2079, .T. ) ;
#16430=DIRECTION ( 'NONE',  ( -0.000000000000000000, -0.000000000000000000, -1.000000000000000000 ) ) ;
#16431=CARTESIAN_POINT ( 'NONE',  ( -72.56315672547016504, 197.7246901893026347, -20.20962120078075586 ) ) ;
#16437=CARTESIAN_POINT ( 'NONE',  ( 15.00000000000000000, 191.6227766016837961, 1.224646799147353454E-15 ) ) ;
#16438=CARTESIAN_POINT ( 'NONE',  ( 40.00000000000000711, 0.000000000000000000, 0.000000000000000000 ) ) ;
#16439=CARTESIAN_POINT ( 'NONE',  ( -5.000000000000000888, 171.6227766016838245, 0.000000000000000000 ) ) ;
#16442=CARTESIAN_POINT ( 'NONE',  ( -81.28398610579327510, 202.4851391218124945, -16.50809708901795148 ) ) ;
#16443=CARTESIAN_POINT ( 'NONE',  ( 196.0000000000000000, 191.6227766016837677, -5.571800142134975431 ) ) ;
#16445=LINE ( 'NONE', #14756, #10971 ) ;
#16446=FACE_OUTER_BOUND ( 'NONE', #7168, .T. ) ;
#16447=ORIENTED_EDGE ( 'NONE', *, *, #5475, .T. ) ;
#16448=ADVANCED_FACE ( 'NONE', ( #7435 ), #3193, .T. ) ;
#16450=CARTESIAN_POINT ( 'NONE',  ( -68.00000000000000000, 171.6227766016838245, 0.000000000000000000 ) ) ;
#16451=ORIENTED_EDGE ( 'NONE', *, *, #15693, .F. ) ;
#16453=CIRCLE ( 'NONE', #10776, 8.000000000000000000 ) ;
#16454=ORIENTED_EDGE ( 'NONE', *, *, #16392, .T. ) ;
#16457=ORIENTED_EDGE ( 'NONE', *, *, #5640, .F. ) ;
#16463=CARTESIAN_POINT ( 'NONE',  ( 13.38958197704232056, 130.3612470323695902, -12.52688079436099144 ) ) ;
#16465=CARTESIAN_POINT ( 'NONE',  ( -76.47766082881949501, 151.4845562501469942, -28.62650789566041709 ) ) ;
#16466=DIRECTION ( 'NONE',  ( 0.000000000000000000, 0.000000000000000000, 1.000000000000000000 ) ) ;
#16470=FACE_OUTER_BOUND ( 'NONE', #10751, .T. ) ;
#16472=DIRECTION ( 'NONE',  ( -0.000000000000000000, -0.000000000000000000, 1.000000000000000000 ) ) ;
#16474=CYLINDRICAL_SURFACE ( 'NONE', #3939, 2.500000000000000444 ) ;
#16478=ORIENTED_EDGE ( 'NONE', *, *, #9014, .T. ) ;
#16479=EDGE_LOOP ( 'NONE', ( #1924, #13326, #7647, #11714 ) ) ;
#16480=CARTESIAN_POINT ( 'NONE',  ( 23.06881488990584472, 29.89244155294396066, -10.82591622123929653 ) ) ;
#16482=CARTESIAN_POINT ( 'NONE',  ( 34.93420767853316988, 30.00000000000000000, -15.00000000000000000 ) ) ;
#16483=ORIENTED_EDGE ( 'NONE', *, *, #16038, .T. ) ;
#16484=ADVANCED_FACE ( 'NONE', ( #16826 ), #4698, .F. ) ;
#16489=CARTESIAN_POINT ( 'NONE',  ( 35.93543503013834339, 151.2142461003564335, -25.93356563065114528 ) ) ;
#16490=CARTESIAN_POINT ( 'NONE',  ( -72.50000000000002842, 146.6227766016838245, -21.54065922853802562 ) ) ;
#16491=LINE ( 'NONE', #3548, #6970 ) ;
#16492=CARTESIAN_POINT ( 'NONE',  ( 40.00000000000000000, 20.00000000000000000, 0.000000000000000000 ) ) ;
#16494=DIRECTION ( 'NONE',  ( 0.000000000000000000, -0.4999999999999952816, 0.8660254037844413721 ) ) ;
#16499=CARTESIAN_POINT ( 'NONE',  ( -22.99999999999999289, 90.00000000000000000, -15.00000000000000000 ) ) ;
#16500=PLANE ( 'NONE',  #2743 ) ;
#16502=ORIENTED_EDGE ( 'NONE', *, *, #12951, .F. ) ;
#16509=CARTESIAN_POINT ( 'NONE',  ( -27.99999999999998224, 10.00000000000000000, 1.387778780781445676E-14 ) ) ;
#16510=LINE ( 'NONE', #12438, #10327 ) ;
#16511=CARTESIAN_POINT ( 'NONE',  ( -80.00000000000002842, 146.6227766016838245, -13.00000000000000000 ) ) ;
#16515=ORIENTED_EDGE ( 'NONE', *, *, #937, .F. ) ;
#16516=CARTESIAN_POINT ( 'NONE',  ( -75.00711853871067092, 199.9683764595549178, -20.53727899274374025 ) ) ;
#16517=FACE_OUTER_BOUND ( 'NONE', #11749, .T. ) ;
#16518=CARTESIAN_POINT ( 'NONE',  ( 22.61491075001043782, 19.99999999999999645, -23.50024419593056635 ) ) ;
#16523=VERTEX_POINT ( 'NONE', #17433 ) ;
#16527=EDGE_LOOP ( 'NONE', ( #1558, #2971, #12371, #10135 ) ) ;
#16529=DIRECTION ( 'NONE',  ( 0.000000000000000000, 0.000000000000000000, 1.000000000000000000 ) ) ;
#16530=CARTESIAN_POINT ( 'NONE',  ( -5.000000000000004441, 134.2062027339443944, -25.00000000000000000 ) ) ;
#16533=ADVANCED_FACE ( 'NONE', ( #3898, #5212 ), #15925, .T. ) ;
#16534=EDGE_CURVE ( 'NONE', #15849, #2797, #10703, .T. ) ;
#16535=LINE ( 'NONE', #503, #4406 ) ;
#16538=EDGE_CURVE ( 'NONE', #3758, #11751, #5134, .T. ) ;
#16539=VERTEX_POINT ( 'NONE', #17257 ) ;
#16543=FACE_OUTER_BOUND ( 'NONE', #10065, .T. ) ;
#16544=CARTESIAN_POINT ( 'NONE',  ( 17.03671980602049985, 126.4628225884666932, -7.681944018317823364 ) ) ;
#16545=VECTOR ( 'NONE', #17222, 1000.000000000000000 ) ;
#16550=CARTESIAN_POINT ( 'NONE',  ( -85.13898110008898357, 193.5203449394525137, -27.30457132278912624 ) ) ;
#16551=EDGE_CURVE ( 'NONE', #6848, #11049, #11849, .T. ) ;
#16556=DIRECTION ( 'NONE',  ( 0.000000000000000000, 1.000000000000000000, 0.000000000000000000 ) ) ;
#16557=CARTESIAN_POINT ( 'NONE',  ( -3.000000000000000888, 191.6227766016837961, 1.224646799147353454E-15 ) ) ;
#16561=ORIENTED_EDGE ( 'NONE', *, *, #16038, .F. ) ;
#16564=CARTESIAN_POINT ( 'NONE',  ( -27.99999999999998224, 10.00000000000000000, -28.00000000000000355 ) ) ;
#16567=DIRECTION ( 'NONE',  ( 0.000000000000000000, 0.000000000000000000, -1.000000000000000000 ) ) ;
#16568=VECTOR ( 'NONE', #2812, 1000.000000000000000 ) ;
#16571=CIRCLE ( 'NONE', #5250, 12.00000000000000000 ) ;
#16572=CARTESIAN_POINT ( 'NONE',  ( 37.05152766480231463, 199.2234891967518706, -18.10843944793624516 ) ) ;
#16579=EDGE_CURVE ( 'NONE', #15849, #12705, #16299, .T. ) ;
#16581=TOROIDAL_SURFACE ( 'NONE', #8930, 740.0000000000000000, 10.00000000000000000 ) ;
#16582=ORIENTED_EDGE ( 'NONE', *, *, #17290, .T. ) ;
#16583=CARTESIAN_POINT ( 'NONE',  ( 17.91514137517177474, 140.8731888928338094, -16.72020691847105667 ) ) ;
#16586=CARTESIAN_POINT ( 'NONE',  ( -72.50000000000000000, 196.4352734575233228, -21.75827460206395614 ) ) ;
#16589=ORIENTED_EDGE ( 'NONE', *, *, #12510, .T. ) ;
#16591=CARTESIAN_POINT ( 'NONE',  ( -38.00000000000000000, 20.00000000000000000, -28.00000000000000355 ) ) ;
#16594=VECTOR ( 'NONE', #7014, 1000.000000000000000 ) ;
#16595=ORIENTED_EDGE ( 'NONE', *, *, #13025, .T. ) ;
#16596=DIRECTION ( 'NONE',  ( -0.000000000000000000, -0.000000000000000000, -1.000000000000000000 ) ) ;
#16600=AXIS2_PLACEMENT_3D ( 'NONE', #14510, #6361, #9105 ) ;
#16605=EDGE_CURVE ( 'NONE', #1820, #874, #13769, .T. ) ;
#16606=EDGE_LOOP ( 'NONE', ( #14127, #7505, #9788, #7434, #2380 ) ) ;
#16607=CARTESIAN_POINT ( 'NONE',  ( -75.92662808041686162, 201.0442424278814713, -18.96251499051319556 ) ) ;
#16608=CARTESIAN_POINT ( 'NONE',  ( -90.33974596215564645, 171.6227766016838245, 0.000000000000000000 ) ) ;
#16609=CARTESIAN_POINT ( 'NONE',  ( 32.29638371061065527, 20.00000000000000355, -15.01265034258821096 ) ) ;
#16613=ORIENTED_EDGE ( 'NONE', *, *, #9265, .T. ) ;
#16617=COLOUR_RGB ( '', 0.08235294, 0.09019608, 0.10196078) ;
#16621=DIRECTION ( 'NONE',  ( 1.000000000000000000, 0.000000000000000000, 0.000000000000000000 ) ) ;
#16623=VERTEX_POINT ( 'NONE', #5567 ) ;
#16624=CARTESIAN_POINT ( 'NONE',  ( 21.99999999999998224, 9.999999999999998224, -30.00000000000001066 ) ) ;
#16627=B_SPLINE_CURVE_WITH_KNOTS ( 'NONE', 3,
 ( #3127, #8338, #376, #1530, #13755, #1717, #7025, #7110, #8525, #12245, #13932, #1795, #5869, #14902, #5521, #10909, #4198, #9585, #14989, #6929, #12333, #5612 ),
 .UNSPECIFIED., .F., .F.,
 ( 4, 2, 2, 2, 2, 2, 2, 2, 2, 2, 4 ),
 ( 0.000000000000000000, 0.001700754388868652408, 0.003401508777737304815, 0.005102263166605957440, 0.005952640361040282234, 0.006803017555474607028, 0.008503771944343253147, 0.01020452633321189927, 0.01190528072208054712, 0.01275565791651486931, 0.01360603511094918977 ),
 .UNSPECIFIED. ) ;
#16628=DIRECTION ( 'NONE',  ( 0.000000000000000000, 0.000000000000000000, 1.000000000000000000 ) ) ;
#16629=DIRECTION ( 'NONE',  ( 0.000000000000000000, 0.000000000000000000, 1.000000000000000000 ) ) ;
#16632=LINE ( 'NONE', #4499, #12938 ) ;
#16634=DIRECTION ( 'NONE',  ( -0.000000000000000000, -0.000000000000000000, 1.000000000000000000 ) ) ;
#16640=CIRCLE ( 'NONE', #2782, 5.000000000000000888 ) ;
#16641=ADVANCED_FACE ( 'NONE', ( #3085 ), #9810, .T. ) ;
#16642=ORIENTED_EDGE ( 'NONE', *, *, #12573, .F. ) ;
#16643=DIRECTION ( 'NONE',  ( 1.000000000000000000, 0.000000000000000000, 0.000000000000000000 ) ) ;
#16646=ORIENTED_EDGE ( 'NONE', *, *, #15921, .F. ) ;
#16653=CIRCLE ( 'NONE', #15501, 2.500000000000000444 ) ;
#16655=AXIS2_PLACEMENT_3D ( 'NONE', #5646, #16271, #4141 ) ;
#16659=CARTESIAN_POINT ( 'NONE',  ( 25.06493225413665016, 20.00000000000000000, -5.000000000000004441 ) ) ;
#16660=CARTESIAN_POINT ( 'NONE',  ( 26.01985846803728464, 139.8002605074728990, -8.764508151440994155 ) ) ;
#16661=ORIENTED_EDGE ( 'NONE', *, *, #9137, .T. ) ;
#16663=DIRECTION ( 'NONE',  ( -1.000000000000000000, -0.000000000000000000, -0.000000000000000000 ) ) ;
#16667=CARTESIAN_POINT ( 'NONE',  ( 27.73879888791969961, 153.7971187266995230, -27.77174765869275319 ) ) ;
#16672=CARTESIAN_POINT ( 'NONE',  ( -68.00000000000000000, 154.3022685259950038, -9.999999999999900524 ) ) ;
#16680=EDGE_CURVE ( 'NONE', #4370, #15922, #1896, .T. ) ;
#16682=FACE_OUTER_BOUND ( 'NONE', #9024, .T. ) ;
#16683=ORIENTED_EDGE ( 'NONE', *, *, #13974, .T. ) ;
#16684=DIRECTION ( 'NONE',  ( 0.000000000000000000, -1.000000000000000000, 0.000000000000000000 ) ) ;
#16687=CIRCLE ( 'NONE', #10454, 5.000000000000000888 ) ;
#16689=DIRECTION ( 'NONE',  ( -1.000000000000000000, 0.000000000000000000, 0.000000000000000000 ) ) ;
#16691=DIRECTION ( 'NONE',  ( -0.000000000000000000, -0.000000000000000000, -1.000000000000000000 ) ) ;
#16695=CARTESIAN_POINT ( 'NONE',  ( -7.379000772444995526, 18.00000000000000355, -12.99999999999999822 ) ) ;
#16696=ORIENTED_EDGE ( 'NONE', *, *, #9111, .F. ) ;
#16697=CARTESIAN_POINT ( 'NONE',  ( 27.44407568426044008, 138.8271129316868837, -3.666666666666658081 ) ) ;
#16698=CARTESIAN_POINT ( 'NONE',  ( -48.00000000000000000, 206.6227766016838245, 2.143131898507868248E-15 ) ) ;
#16700=EDGE_CURVE ( 'NONE', #8437, #12225, #2745, .T. ) ;
#16702=PLANE ( 'NONE',  #15438 ) ;
#16703=AXIS2_PLACEMENT_3D ( 'NONE', #9692, #14928, #16356 ) ;
#16705=ORIENTED_EDGE ( 'NONE', *, *, #4333, .T. ) ;
#16706=EDGE_LOOP ( 'NONE', ( #14376, #13712, #15884, #13491 ) ) ;
#16711=EDGE_CURVE ( 'NONE', #6145, #11303, #7539, .T. ) ;
#16717=DIRECTION ( 'NONE',  ( 0.000000000000000000, 0.000000000000000000, 1.000000000000000000 ) ) ;
#16718=VECTOR ( 'NONE', #1996, 1000.000000000000000 ) ;
#16719=CARTESIAN_POINT ( 'NONE',  ( 35.59781103574917438, 141.6107120069883365, -13.74530841833676931 ) ) ;
#16722=DIRECTION ( 'NONE',  ( -1.000000000000000000, -0.000000000000000000, -0.000000000000000000 ) ) ;
#16723=DIRECTION ( 'NONE',  ( 0.000000000000000000, 0.000000000000000000, -1.000000000000000000 ) ) ;
#16724=CARTESIAN_POINT ( 'NONE',  ( -16.41264213764281976, 19.99999999999999645, -23.02790928165778794 ) ) ;
#16726=AXIS2_PLACEMENT_3D ( 'NONE', #16439, #5532, #10923 ) ;
#16732=ORIENTED_EDGE ( 'NONE', *, *, #12549, .T. ) ;
#16733=CARTESIAN_POINT ( 'NONE',  ( -95.00000000000000000, 199.3133755249253056, -1.695560166891042033E-15 ) ) ;
#16735=ORIENTED_EDGE ( 'NONE', *, *, #13863, .F. ) ;
#16736=LINE ( 'NONE', #15482, #17166 ) ;
#16737=VECTOR ( 'NONE', #3202, 1000.000000000000000 ) ;
#16739=EDGE_CURVE ( 'NONE', #7107, #919, #15378, .T. ) ;
#16743=FACE_BOUND ( 'NONE', #11753, .T. ) ;
#16744=ORIENTED_EDGE ( 'NONE', *, *, #10406, .T. ) ;
#16745=ORIENTED_EDGE ( 'NONE', *, *, #1918, .F. ) ;
#16746=CYLINDRICAL_SURFACE ( 'NONE', #10895, 5.000000000000000888 ) ;
#16747=CARTESIAN_POINT ( 'NONE',  ( 22.64347415271929265, 141.1870565414818941, -12.76399958404563684 ) ) ;
#16750=CARTESIAN_POINT ( 'NONE',  ( 33.99999999999998579, 9.999999999999998224, -30.00000000000001066 ) ) ;
#16751=ORIENTED_EDGE ( 'NONE', *, *, #5854, .F. ) ;
#16752=DIRECTION ( 'NONE',  ( 0.000000000000000000, 0.000000000000000000, 1.000000000000000000 ) ) ;
#16753=CARTESIAN_POINT ( 'NONE',  ( 48.00000000000000000, 196.6227766016838245, 0.000000000000000000 ) ) ;
#16754=CARTESIAN_POINT ( 'NONE',  ( 49.99999999999998579, 159.6227766016838814, -5.571800142134975431 ) ) ;
#16755=DIRECTION ( 'NONE',  ( -1.000000000000000000, 0.000000000000000000, 0.000000000000000000 ) ) ;
#16759=CARTESIAN_POINT ( 'NONE',  ( 14.93242934743710393, 30.00000000000000000, -25.00000000000000000 ) ) ;
#16761=CARTESIAN_POINT ( 'NONE',  ( -80.00000000000001421, 196.6227766016838245, -16.00000000000000000 ) ) ;
#16762=ORIENTED_EDGE ( 'NONE', *, *, #13334, .F. ) ;
#16767=ORIENTED_EDGE ( 'NONE', *, *, #14847, .F. ) ;
#16769=CARTESIAN_POINT ( 'NONE',  ( -74.10786375645523094, 201.2861607625692102, -14.48320912595414889 ) ) ;
#16771=ORIENTED_EDGE ( 'NONE', *, *, #4335, .T. ) ;
#16777=CARTESIAN_POINT ( 'NONE',  ( 48.00000000000000711, 175.6227766016838245, -3.071800142134975431 ) ) ;
#16781=DIRECTION ( 'NONE',  ( -1.000000000000000000, -0.000000000000000000, -0.000000000000000000 ) ) ;
#16782=DIRECTION ( 'NONE',  ( 0.000000000000000000, 0.000000000000000000, -1.000000000000000000 ) ) ;
#16791=ORIENTED_EDGE ( 'NONE', *, *, #4924, .T. ) ;
#16792=CARTESIAN_POINT ( 'NONE',  ( -3.000000000000000888, 171.6227766016838245, 0.000000000000000000 ) ) ;
#16797=VERTEX_POINT ( 'NONE', #6007 ) ;
#16804=EDGE_CURVE ( 'NONE', #4853, #1445, #8905, .T. ) ;
#16805=DIRECTION ( 'NONE',  ( -0.000000000000000000, -0.000000000000000000, 1.000000000000000000 ) ) ;
#16806=VERTEX_POINT ( 'NONE', #10158 ) ;
#16807=CARTESIAN_POINT ( 'NONE',  ( -38.00000000000000000, 18.00000000000000355, -28.00000000000000355 ) ) ;
#16810=DIRECTION ( 'NONE',  ( -1.156482317317868274E-16, 1.000000000000000000, 0.000000000000000000 ) ) ;
#16812=DIRECTION ( 'NONE',  ( 1.000000000000000000, 0.000000000000000000, 0.000000000000000000 ) ) ;
#16817=CARTESIAN_POINT ( 'NONE',  ( -24.94987437106622252, 120.0000000000000284, -6.000000000000001776 ) ) ;
#16818=CARTESIAN_POINT ( 'NONE',  ( 25.00907797400832777, 199.9711820797445512, -20.53336423377503195 ) ) ;
#16820=VERTEX_POINT ( 'NONE', #16807 ) ;
#16823=CARTESIAN_POINT ( 'NONE',  ( 21.36708699129162881, 19.99999999999999645, -23.94811280430947420 ) ) ;
#16824=CARTESIAN_POINT ( 'NONE',  ( 27.32038637416026816, 139.0270950805171424, -5.204462201318943215 ) ) ;
#16825=EDGE_LOOP ( 'NONE', ( #9782, #9412, #11732, #6126 ) ) ;
#16826=FACE_OUTER_BOUND ( 'NONE', #2519, .T. ) ;
#16827=CARTESIAN_POINT ( 'NONE',  ( 8.147273376221958685, 133.4207317082267537, -12.78321197947435728 ) ) ;
#16829=EDGE_CURVE ( 'NONE', #9334, #3758, #13121, .T. ) ;
#16832=AXIS2_PLACEMENT_3D ( 'NONE', #5939, #15126, #9727 ) ;
#16834=CARTESIAN_POINT ( 'NONE',  ( -43.00000000000000000, 130.0000000000000000, 0.000000000000000000 ) ) ;
#16836=DIRECTION ( 'NONE',  ( 1.000000000000000000, 0.000000000000000000, 0.000000000000000000 ) ) ;
#16843=FACE_BOUND ( 'NONE', #15157, .T. ) ;
#16846=CARTESIAN_POINT ( 'NONE',  ( -100.0000000000000000, 134.2062027339443944, -25.00000000000000000 ) ) ;
#16848=EDGE_CURVE ( 'NONE', #1445, #583, #13204, .T. ) ;
#16852=CARTESIAN_POINT ( 'NONE',  ( 196.0000000000000000, 175.6227766016838530, -16.92820660268601429 ) ) ;
#16853=ORIENTED_EDGE ( 'NONE', *, *, #8803, .F. ) ;
#16855=CYLINDRICAL_SURFACE ( 'NONE', #5822, 2.500000000000002220 ) ;
#16856=CLOSED_SHELL ( 'NONE', ( #11796, #5680, #14850, #2023, #6557, #16920, #1053, #933, #4994, #4656, #10132, #9907, #5575, #8351, #3212, #219, #13653, #11803, #5988, #5668, #2330, #15640, #14040, #3755, #6953, #16641, #15226, #5670, #1743, #8387, #11006, #1032, #16000, #3380, #11104, #16484, #9970, #12991, #2677, #2128, #8550, #6235, #4622, #6343, #15932, #15525, #9786, #6889, #3053, #10882, #9139, #10668, #14166, #4746, #5272, #14560, #8462, #7812, #13983, #11967, #15068, #173, #11312, #125, #7017, #11984, #8917, #2898, #1195, #7664, #1764, #13459, #2182, #12492, #16142, #17450, #721, #14164, #5993, #14540, #15607, #3920, #6203, #1777, #6050, #10148, #11367, #2273, #14735, #9806, #1315, #11166, #4674, #3261, #13233, #470, #1673, #8776, #16921, #4782, #9679, #2656, #9962, #1575, #392, #13113, #7153, #5155, #1253, #9549, #3533, #8682, #14909, #17463, #3252, #11420, #3860, #16957, #13388, #14303, #779, #7523, #4873, #14346, #4031, #3168, #2496, #13920, #7269, #3697, #14852, #6016, #14387, #17106, #7917, #12933, #8029, #15986, #1768, #10442, #4790, #6474, #13169, #11110, #8804, #7717, #4602, #11862, #15612, #2385, #9774, #12282, #16448, #7491, #10243, #15225, #11275, #16533, #8228, #4948, #15552, #10560, #15611, #16426, #14078, #3213, #8226, #14629, #7177, #4039, #7279, #3474, #16916, #8814, #9405, #17161, #2350, #4998, #2456, #10955, #865, #2300, #3458, #5656, #1817, #16234, #910 ) ) ;
#16857=AXIS2_PLACEMENT_3D ( 'NONE', #914, #6390, #5161 ) ;
#16859=CARTESIAN_POINT ( 'NONE',  ( -18.25212770525996930, 32.30769230769229949, -5.349717987761776428 ) ) ;
#16862=DIRECTION ( 'NONE',  ( -1.000000000000000000, -0.000000000000000000, -0.000000000000000000 ) ) ;
#16863=ORIENTED_EDGE ( 'NONE', *, *, #7151, .T. ) ;
#16868=FACE_OUTER_BOUND ( 'NONE', #9157, .T. ) ;
#16870=ORIENTED_EDGE ( 'NONE', *, *, #3798, .T. ) ;
#16871=AXIS2_PLACEMENT_3D ( 'NONE', #4874, #897, #10529 ) ;
#16873=EDGE_LOOP ( 'NONE', ( #14043, #15481 ) ) ;
#16874=( NAMED_UNIT ( * ) PLANE_ANGLE_UNIT ( ) SI_UNIT ( $, .RADIAN. ) );
#16875=AXIS2_PLACEMENT_3D ( 'NONE', #8847, #12759, #8928 ) ;
#16882=ORIENTED_EDGE ( 'NONE', *, *, #9111, .T. ) ;
#16884=DIRECTION ( 'NONE',  ( 0.000000000000000000, 0.000000000000000000, 1.000000000000000000 ) ) ;
#16891=DIRECTION ( 'NONE',  ( 0.000000000000000000, 0.000000000000000000, -1.000000000000000000 ) ) ;
#16899=DIRECTION ( 'NONE',  ( 1.000000000000000000, 0.000000000000000000, 0.000000000000000000 ) ) ;
#16901=CARTESIAN_POINT ( 'NONE',  ( 6.471945315774715546, 134.1315750335306518, -12.99999999999999822 ) ) ;
#16902=ORIENTED_EDGE ( 'NONE', *, *, #6233, .T. ) ;
#16906=EDGE_LOOP ( 'NONE', ( #4832, #12435, #3429, #5851, #5522, #1882, #362 ) ) ;
#16907=VECTOR ( 'NONE', #10474, 1000.000000000000000 ) ;
#16908=ORIENTED_EDGE ( 'NONE', *, *, #3325, .T. ) ;
#16910=CARTESIAN_POINT ( 'NONE',  ( 20.21654089865888437, 29.92961455958988637, -13.49713695059922891 ) ) ;
#16911=CIRCLE ( 'NONE', #14366, 2.499999999999998668 ) ;
#16912=DIRECTION ( 'NONE',  ( -1.000000000000000000, -0.000000000000000000, -0.000000000000000000 ) ) ;
#16916=ADVANCED_FACE ( 'NONE', ( #13348, #5192 ), #2359, .F. ) ;
#16918=CARTESIAN_POINT ( 'NONE',  ( 27.99999999999998224, 9.999999999999998224, -16.00000000000000000 ) ) ;
#16920=ADVANCED_FACE ( 'NONE', ( #3608 ), #3698, .F. ) ;
#16921=ADVANCED_FACE ( 'NONE', ( #7585, #15907, #10584 ), #14411, .T. ) ;
#16923=AXIS2_PLACEMENT_3D ( 'NONE', #525, #16812, #4774 ) ;
#16925=DIRECTION ( 'NONE',  ( 0.000000000000000000, -0.000000000000000000, 1.000000000000000000 ) ) ;
#16927=FACE_OUTER_BOUND ( 'NONE', #3855, .T. ) ;
#16928=CARTESIAN_POINT ( 'NONE',  ( 29.73563295595405975, 140.6225526278764733, -16.24764948572449796 ) ) ;
#16936=CARTESIAN_POINT ( 'NONE',  ( 225.0000000000000000, 89.99999999999997158, -13.00000000000000000 ) ) ;
#16937=VECTOR ( 'NONE', #3031, 1000.000000000000000 ) ;
#16938=EDGE_LOOP ( 'NONE', ( #6354, #12835, #7111, #633 ) ) ;
#16939=FACE_OUTER_BOUND ( 'NONE', #15896, .T. ) ;
#16940=VECTOR ( 'NONE', #17373, 1000.000000000000000 ) ;
#16943=DIRECTION ( 'NONE',  ( 8.673617379884037937E-17, 0.000000000000000000, 1.000000000000000000 ) ) ;
#16945=CIRCLE ( 'NONE', #11577, 12.00000000000000000 ) ;
#16947=CARTESIAN_POINT ( 'NONE',  ( -10.71009414332545973, 30.74249144840758063, -14.53036023671900168 ) ) ;
#16948=DIRECTION ( 'NONE',  ( 0.000000000000000000, -1.000000000000000000, -6.123233995736762338E-17 ) ) ;
#16950=DIRECTION ( 'NONE',  ( 1.000000000000000000, 0.000000000000000000, 0.000000000000000000 ) ) ;
#16953=DIRECTION ( 'NONE',  ( -0.000000000000000000, -0.000000000000000000, 1.000000000000000000 ) ) ;
#16956=FACE_OUTER_BOUND ( 'NONE', #16997, .T. ) ;
#16957=ADVANCED_FACE ( 'NONE', ( #8371 ), #1395, .F. ) ;
#16959=CARTESIAN_POINT ( 'NONE',  ( 27.59167911046515087, 191.1229741556853128, -29.06467671913508966 ) ) ;
#16960=DIRECTION ( 'NONE',  ( 0.000000000000000000, 0.000000000000000000, 1.000000000000000000 ) ) ;
#16961=ORIENTED_EDGE ( 'NONE', *, *, #11698, .F. ) ;
#16962=VERTEX_POINT ( 'NONE', #12457 ) ;
#16963=CIRCLE ( 'NONE', #1134, 25.00000000000000000 ) ;
#16965=VERTEX_POINT ( 'NONE', #4135 ) ;
#16967=AXIS2_PLACEMENT_3D ( 'NONE', #6461, #2654, #11854 ) ;
#16968=VERTEX_POINT ( 'NONE', #17510 ) ;
#16969=CARTESIAN_POINT ( 'NONE',  ( 27.99999999999998224, 9.999999999999998224, -28.00000000000001066 ) ) ;
#16971=CARTESIAN_POINT ( 'NONE',  ( 40.00000000000000711, 171.6227766016838245, 0.000000000000000000 ) ) ;
#16973=VERTEX_POINT ( 'NONE', #9523 ) ;
#16975=VECTOR ( 'NONE', #7939, 1000.000000000000000 ) ;
#16976=AXIS2_PLACEMENT_3D ( 'NONE', #15467, #1834, #510 ) ;
#16977=CARTESIAN_POINT ( 'NONE',  ( 49.99999999999998579, 155.6227766016839098, -12.50000337241049309 ) ) ;
#16979=CARTESIAN_POINT ( 'NONE',  ( -25.00000000000000000, 120.0000000000000426, -10.85786437626905077 ) ) ;
#16981=CARTESIAN_POINT ( 'NONE',  ( -10.84365596476886395, 30.77158821550125722, -14.49076147631418721 ) ) ;
#16985=AXIS2_PLACEMENT_3D ( 'NONE', #10840, #9599, #9248 ) ;
#16987=DIRECTION ( 'NONE',  ( 0.000000000000000000, -1.000000000000000000, -7.341990890863118602E-16 ) ) ;
#16989=CARTESIAN_POINT ( 'NONE',  ( 22.50000000000001421, 146.6227766016838245, -35.00200000000000244 ) ) ;
#16990=EDGE_CURVE ( 'NONE', #209, #10464, #9813, .T. ) ;
#16991=CARTESIAN_POINT ( 'NONE',  ( 14.23753691287610579, 127.5498911642838635, -8.870798623635511859 ) ) ;
#16993=CARTESIAN_POINT ( 'NONE',  ( -80.00000000000001421, 196.6227766016838245, -16.00000000000000000 ) ) ;
#16996=CARTESIAN_POINT ( 'NONE',  ( 33.15164470903668104, 201.7321575960915254, -17.84571802696398279 ) ) ;
#16997=EDGE_LOOP ( 'NONE', ( #486, #11665, #15061, #12880 ) ) ;
#17000=CARTESIAN_POINT ( 'NONE',  ( 17.20984524040877872, 19.99999999999999645, -14.76996962246643896 ) ) ;
#17002=ORIENTED_EDGE ( 'NONE', *, *, #17322, .T. ) ;
#17003=PLANE ( 'NONE',  #9229 ) ;
#17006=DIRECTION ( 'NONE',  ( 0.000000000000000000, 1.000000000000000000, 0.000000000000000000 ) ) ;
#17007=CIRCLE ( 'NONE', #12194, 6.000000000000005329 ) ;
#17013=CARTESIAN_POINT ( 'NONE',  ( 17.00000000000000000, 154.3022685259950038, -9.999999999999900524 ) ) ;
#17018=DIRECTION ( 'NONE',  ( 0.000000000000000000, 0.000000000000000000, 1.000000000000000000 ) ) ;
#17025=B_SPLINE_CURVE_WITH_KNOTS ( 'NONE', 3,
 ( #13814, #8395, #4074, #15214, #84, #8490, #12291, #15032, #422, #8134, #2911, #164, #5573, #344, #8300, #13904, #5829, #13713, #1584, #10870, #259, #6985, #4160, #5663, #1679, #1762, #11053, #7079, #14863, #7159, #14948, #4331, #12476, #11131, #16550, #9453, #15382, #6010, #614, #10161, #697, #6266, #1937, #4599 ),
 .UNSPECIFIED., .F., .F.,
 ( 4, 2, 2, 2, 2, 2, 2, 2, 2, 2, 2, 2, 2, 2, 2, 2, 2, 2, 2, 2, 2, 4 ),
 ( 0.000000000000000000, 0.002715240924237333209, 0.003394051155296675618, 0.004072861386356018028, 0.005430481848474658611, 0.006788102310593301797, 0.008145722772711942380, 0.009503343234830586433, 0.01018215346588990759, 0.01086096369694922875, 0.01153977392800854991, 0.01221858415906786934, 0.01289739439012719223, 0.01357620462118651339, 0.01493382508330519561, 0.01629144554542387782, 0.01697025577648323194, 0.01764906600754258606, 0.01900668646966127348, 0.01968549670072059291, 0.02036430693177990886, 0.02172192739389853383 ),
 .UNSPECIFIED. ) ;
#17028=CARTESIAN_POINT ( 'NONE',  ( 196.0000000000000000, 151.6227766016839098, -3.071800142134974099 ) ) ;
#17029=CARTESIAN_POINT ( 'NONE',  ( -9.392228533940972568, 30.65825049985634010, -12.80200153553487752 ) ) ;
#17031=DIRECTION ( 'NONE',  ( -1.000000000000000000, 0.000000000000000000, 0.000000000000000000 ) ) ;
#17032=CARTESIAN_POINT ( 'NONE',  ( -17.58288004918492931, 20.00000000000000355, -22.43027208364174285 ) ) ;
#17033=ORIENTED_EDGE ( 'NONE', *, *, #11009, .F. ) ;
#17034=CARTESIAN_POINT ( 'NONE',  ( 35.90059120242804624, 195.3277913626825466, -25.76530748039452590 ) ) ;
#17036=ORIENTED_EDGE ( 'NONE', *, *, #4250, .T. ) ;
#17039=CARTESIAN_POINT ( 'NONE',  ( -72.50000000000002842, 146.6227766016838245, -21.54065922853802562 ) ) ;
#17042=EDGE_CURVE ( 'NONE', #1250, #2797, #6431, .T. ) ;
#17043=DIRECTION ( 'NONE',  ( -1.000000000000000000, -0.000000000000000000, 0.000000000000000000 ) ) ;
#17044=LINE ( 'NONE', #4911, #6941 ) ;
#17045=CARTESIAN_POINT ( 'NONE',  ( 35.27494917608787972, 141.2912748254776147, -13.00000000000000000 ) ) ;
#17047=CARTESIAN_POINT ( 'NONE',  ( 35.49999999999998579, 9.999999999999998224, -13.00000000000000000 ) ) ;
#17065=DIRECTION ( 'NONE',  ( 0.000000000000000000, 1.000000000000000000, 0.000000000000000000 ) ) ;
#17066=MANIFOLD_SOLID_BREP ( '<Left Housing Shell>-<Boss-Extrude6>', #16856 ) ;
#17067=CARTESIAN_POINT ( 'NONE',  ( 30.00000000000000355, 196.6227766016838245, -16.00000000000000000 ) ) ;
#17070=DIRECTION ( 'NONE',  ( 1.000000000000000000, 0.000000000000000000, 0.000000000000000000 ) ) ;
#17072=ORIENTED_EDGE ( 'NONE', *, *, #10012, .F. ) ;
#17075=CARTESIAN_POINT ( 'NONE',  ( 16.23563086566769442, 20.00000000000456879, -14.95434718295347665 ) ) ;
#17077=CARTESIAN_POINT ( 'NONE',  ( 11.08062248138317685, 138.8595139650515193, -13.56485289975001862 ) ) ;
#17078=ORIENTED_EDGE ( 'NONE', *, *, #9845, .T. ) ;
#17082=EDGE_LOOP ( 'NONE', ( #14107, #749, #16229, #17333 ) ) ;
#17083=CARTESIAN_POINT ( 'NONE',  ( 30.00000000000000355, 196.6227766016838245, -35.00200000000000244 ) ) ;
#17088=AXIS2_PLACEMENT_3D ( 'NONE', #3644, #17090, #3552 ) ;
#17090=DIRECTION ( 'NONE',  ( -1.000000000000000000, -0.000000000000000000, 0.000000000000000000 ) ) ;
#17094=CARTESIAN_POINT ( 'NONE',  ( 30.00000000000000355, 196.6227766016838245, 1.387778780781445676E-14 ) ) ;
#17097=ORIENTED_EDGE ( 'NONE', *, *, #10920, .F. ) ;
#17098=EDGE_CURVE ( 'NONE', #9987, #2414, #11789, .T. ) ;
#17100=DIRECTION ( 'NONE',  ( 0.000000000000000000, 0.000000000000000000, 1.000000000000000000 ) ) ;
#17104=ORIENTED_EDGE ( 'NONE', *, *, #7097, .T. ) ;
#17105=DIRECTION ( 'NONE',  ( 0.000000000000000000, 0.000000000000000000, 1.000000000000000000 ) ) ;
#17106=ADVANCED_FACE ( 'NONE', ( #4490 ), #15362, .F. ) ;
#17107=CARTESIAN_POINT ( 'NONE',  ( 27.18614160573789817, 189.6648409365396049, -27.63145166803555242 ) ) ;
#17108=CARTESIAN_POINT ( 'NONE',  ( 20.49999999999998224, 10.00000000000000000, -28.00000000000001066 ) ) ;
#17109=CARTESIAN_POINT ( 'NONE',  ( -19.26597175465492739, 18.00000000000000000, -21.35691006828201566 ) ) ;
#17111=ORIENTED_EDGE ( 'NONE', *, *, #10282, .T. ) ;
#17112=DIRECTION ( 'NONE',  ( 1.000000000000000000, 0.000000000000000000, 0.000000000000000000 ) ) ;
#17113=CIRCLE ( 'NONE', #17411, 5.000000000000004441 ) ;
#17114=ORIENTED_EDGE ( 'NONE', *, *, #624, .F. ) ;
#17115=CYLINDRICAL_SURFACE ( 'NONE', #12700, 2.500000000000000444 ) ;
#17118=ORIENTED_EDGE ( 'NONE', *, *, #8606, .F. ) ;
#17120=CARTESIAN_POINT ( 'NONE',  ( -77.18614160573793015, 153.5807122668280442, -27.63145166803555952 ) ) ;
#17133=CARTESIAN_POINT ( 'NONE',  ( 125.0000000000000000, 0.000000000000000000, 0.000000000000000000 ) ) ;
#17137=AXIS2_PLACEMENT_3D ( 'NONE', #9936, #4633, #12776 ) ;
#17139=VECTOR ( 'NONE', #2778, 1000.000000000000000 ) ;
#17141=ORIENTED_EDGE ( 'NONE', *, *, #13054, .F. ) ;
#17145=LINE ( 'NONE', #10506, #12734 ) ;
#17146=CIRCLE ( 'NONE', #467, 7.499999999999996447 ) ;
#17148=CARTESIAN_POINT ( 'NONE',  ( -78.00663513009409655, 140.9591509882842786, -16.87514788462641491 ) ) ;
#17149=VECTOR ( 'NONE', #15308, 1000.000000000000000 ) ;
#17151=CARTESIAN_POINT ( 'NONE',  ( 15.04007972439966956, 126.3543340278276190, -7.435061541642935978 ) ) ;
#17152=AXIS2_PLACEMENT_3D ( 'NONE', #1759, #8296, #15029 ) ;
#17153=ORIENTED_EDGE ( 'NONE', *, *, #1226, .F. ) ;
#17157=CARTESIAN_POINT ( 'NONE',  ( 28.71601389420674622, 202.4851391218125798, -16.50809708901796213 ) ) ;
#17158=ORIENTED_EDGE ( 'NONE', *, *, #5353, .T. ) ;
#17160=EDGE_CURVE ( 'NONE', #7936, #13265, #10961, .T. ) ;
#17161=ADVANCED_FACE ( 'NONE', ( #12719 ), #11554, .F. ) ;
#17163=CARTESIAN_POINT ( 'NONE',  ( -80.00000000000002842, 146.6227766016838245, -35.00200000000000244 ) ) ;
#17165=CARTESIAN_POINT ( 'NONE',  ( 11.61835878478676598, 131.7755375868723320, -13.65455057792075877 ) ) ;
#17166=VECTOR ( 'NONE', #9983, 1000.000000000000000 ) ;
#17169=AXIS2_PLACEMENT_3D ( 'NONE', #13430, #9433, #14837 ) ;
#17170=CARTESIAN_POINT ( 'NONE',  ( 26.46962346220079709, 139.5657242622003480, -7.835998493359402239 ) ) ;
#17171=ORIENTED_EDGE ( 'NONE', *, *, #4924, .F. ) ;
#17173=DIRECTION ( 'NONE',  ( -1.000000000000000000, -0.000000000000000000, -0.000000000000000000 ) ) ;
#17174=CARTESIAN_POINT ( 'NONE',  ( 22.79003115184357497, 198.7539484232960945, -18.80562413441370850 ) ) ;
#17185=ORIENTED_EDGE ( 'NONE', *, *, #11902, .T. ) ;
#17186=CYLINDRICAL_SURFACE ( 'NONE', #12990, 7.500000000000000000 ) ;
#17188=EDGE_LOOP ( 'NONE', ( #10081, #2007, #10849, #12073 ) ) ;
#17191=VECTOR ( 'NONE', #4984, 1000.000000000000000 ) ;
#17194=CARTESIAN_POINT ( 'NONE',  ( 14.93242934743711992, 20.00000000000000000, -25.00000000000000000 ) ) ;
#17195=CARTESIAN_POINT ( 'NONE',  ( 23.01962815379005178, 193.8465113367682591, -24.40116746791568758 ) ) ;
#17196=CARTESIAN_POINT ( 'NONE',  ( -18.15427578192114666, 32.28835078156378557, -6.388283290543781412 ) ) ;
#17197=CARTESIAN_POINT ( 'NONE',  ( -12.35971836118926959, 18.00000000000000000, -8.238707107740440350 ) ) ;
#17198=EDGE_CURVE ( 'NONE', #7583, #1100, #788, .T. ) ;
#17199=EDGE_LOOP ( 'NONE', ( #9809, #12228 ) ) ;
#17200=PLANE ( 'NONE',  #12672 ) ;
#17203=CARTESIAN_POINT ( 'NONE',  ( 24.00000000000000000, 196.6227766016838245, -24.49489742783178770 ) ) ;
#17204=CIRCLE ( 'NONE', #9569, 2.500000000000000000 ) ;
#17207=ORIENTED_EDGE ( 'NONE', *, *, #6293, .F. ) ;
#17210=VECTOR ( 'NONE', #16663, 1000.000000000000000 ) ;
#17213=CIRCLE ( 'NONE', #3081, 2.500000000000002220 ) ;
#17215=CARTESIAN_POINT ( 'NONE',  ( 27.50000000000000355, 196.6227766016838245, -16.00000000000000000 ) ) ;
#17216=CARTESIAN_POINT ( 'NONE',  ( 34.01748795107550905, 151.0988115558745051, -28.35253695364550452 ) ) ;
#17219=EDGE_CURVE ( 'NONE', #6275, #16623, #10385, .T. ) ;
#17222=DIRECTION ( 'NONE',  ( -0.000000000000000000, -0.000000000000000000, -1.000000000000000000 ) ) ;
#17223=FACE_OUTER_BOUND ( 'NONE', #12532, .T. ) ;
#17225=FACE_OUTER_BOUND ( 'NONE', #14918, .T. ) ;
#17227=CARTESIAN_POINT ( 'NONE',  ( 24.72505082391212028, 201.9542783778900059, -13.00000000000000000 ) ) ;
#17231=EDGE_CURVE ( 'NONE', #8971, #1773, #1306, .T. ) ;
#17235=ORIENTED_EDGE ( 'NONE', *, *, #3820, .F. ) ;
#17241=CARTESIAN_POINT ( 'NONE',  ( -23.00000000000001421, 122.0000000000000284, -4.999999999999999112 ) ) ;
#17242=AXIS2_PLACEMENT_3D ( 'NONE', #10773, #14835, #1299 ) ;
#17246=DIRECTION ( 'NONE',  ( 1.000000000000000000, 0.000000000000000000, 0.000000000000000000 ) ) ;
#17253=VERTEX_POINT ( 'NONE', #14649 ) ;
#17254=AXIS2_PLACEMENT_3D ( 'NONE', #10400, #15811, #9076 ) ;
#17255=CARTESIAN_POINT ( 'NONE',  ( 13.85534145189689248, 141.7971685630157879, -18.31519266891907094 ) ) ;
#17257=CARTESIAN_POINT ( 'NONE',  ( 24.00000000000000355, 146.6227766016838245, -24.49489742783179480 ) ) ;
#17259=CARTESIAN_POINT ( 'NONE',  ( 9.466951579747838963, 140.2095812714875080, -12.14773935231208313 ) ) ;
#17261=CYLINDRICAL_SURFACE ( 'NONE', #12370, 10.00000000000000178 ) ;
#17263=CARTESIAN_POINT ( 'NONE',  ( 23.58001751434002813, 200.5275637277235887, -15.94334347237690075 ) ) ;
#17266=EDGE_CURVE ( 'NONE', #17478, #15620, #10483, .T. ) ;
#17269=CARTESIAN_POINT ( 'NONE',  ( -43.00000000000000711, 130.0000000000000000, -12.99999999999999822 ) ) ;
#17271=VECTOR ( 'NONE', #12410, 1000.000000000000000 ) ;
#17272=DIRECTION ( 'NONE',  ( -1.000000000000000000, -0.000000000000000000, 0.000000000000000000 ) ) ;
#17273=CARTESIAN_POINT ( 'NONE',  ( -40.85786437626905609, 120.0000000000000142, -10.85786437626904721 ) ) ;
#17274=CARTESIAN_POINT ( 'NONE',  ( 31.30883960485276418, 140.7623173628079485, -16.51208758287211253 ) ) ;
#17280=ORIENTED_EDGE ( 'NONE', *, *, #2680, .F. ) ;
#17281=FACE_OUTER_BOUND ( 'NONE', #14133, .T. ) ;
#17288=EDGE_CURVE ( 'NONE', #13094, #15022, #16054, .T. ) ;
#17290=EDGE_CURVE ( 'NONE', #16339, #5589, #13672, .T. ) ;
#17291=DIRECTION ( 'NONE',  ( 1.000000000000000000, 0.000000000000000000, 0.000000000000000000 ) ) ;
#17292=CARTESIAN_POINT ( 'NONE',  ( -34.99999999999999289, 122.0000000000000284, -15.00000000000000000 ) ) ;
#17293=CARTESIAN_POINT ( 'NONE',  ( 196.0000000000000000, 151.6227766016839098, -5.571800142134973655 ) ) ;
#17294=CARTESIAN_POINT ( 'NONE',  ( -12.55890155933072094, 17.99999999999999645, -7.515612101507581855 ) ) ;
#17296=CARTESIAN_POINT ( 'NONE',  ( -80.00000000000002842, 146.6227766016838245, -35.00200000000000244 ) ) ;
#17297=VERTEX_POINT ( 'NONE', #10833 ) ;
#17298=FACE_OUTER_BOUND ( 'NONE', #14011, .T. ) ;
#17299=CARTESIAN_POINT ( 'NONE',  ( -86.65363293176820036, 200.1176944260899688, -16.66575456205189809 ) ) ;
#17304=CARTESIAN_POINT ( 'NONE',  ( -85.08450508553750069, 152.1614365523548713, -26.65369102675423463 ) ) ;
#17306=EDGE_LOOP ( 'NONE', ( #12141, #6726, #1975, #14804 ) ) ;
#17310=CARTESIAN_POINT ( 'NONE',  ( 24.58837873217347081, 149.2402085794911955, -26.91083197558416629 ) ) ;
#17313=ORIENTED_EDGE ( 'NONE', *, *, #16579, .T. ) ;
#17314=FACE_OUTER_BOUND ( 'NONE', #11620, .T. ) ;
#17317=CARTESIAN_POINT ( 'NONE',  ( -15.18548748502429468, 20.00000000000231992, -6.873064813191830602 ) ) ;
#17322=EDGE_CURVE ( 'NONE', #3758, #10541, #12102, .T. ) ;
#17324=CARTESIAN_POINT ( 'NONE',  ( -43.00000000000000000, 140.0000000000000000, -13.00000000000000000 ) ) ;
#17327=DIRECTION ( 'NONE',  ( 1.000000000000000000, 0.000000000000000000, 0.000000000000000000 ) ) ;
#17333=ORIENTED_EDGE ( 'NONE', *, *, #6019, .F. ) ;
#17334=CARTESIAN_POINT ( 'NONE',  ( -100.0000000000000000, 141.2912748254776147, -13.00000000000000000 ) ) ;
#17335=DIRECTION ( 'NONE',  ( 0.000000000000000000, 0.000000000000000000, 1.000000000000000000 ) ) ;
#17339=ORIENTED_EDGE ( 'NONE', *, *, #7461, .F. ) ;
#17340=CARTESIAN_POINT ( 'NONE',  ( 8.956670050029527985, 133.3372912347335841, -14.64653510947197645 ) ) ;
#17342=CARTESIAN_POINT ( 'NONE',  ( -77.79806300862335888, 152.2211730668986434, -29.13124974281949875 ) ) ;
#17343=CARTESIAN_POINT ( 'NONE',  ( 21.84350049701177809, 141.4638053371992328, -13.40107808329819150 ) ) ;
#17344=EDGE_LOOP ( 'NONE', ( #14358, #5187, #10587, #17388 ) ) ;
#17348=LINE ( 'NONE', #2746, #2486 ) ;
#17350=CARTESIAN_POINT ( 'NONE',  ( 48.00000000000000711, 155.6227766016839098, -15.00000337241049486 ) ) ;
#17354=FACE_OUTER_BOUND ( 'NONE', #5704, .T. ) ;
#17355=CARTESIAN_POINT ( 'NONE',  ( -34.99999999999999289, 120.0000000000000284, -4.999999999999999112 ) ) ;
#17358=DIRECTION ( 'NONE',  ( 1.000000000000000000, 0.000000000000000000, 0.000000000000000000 ) ) ;
#17363=EDGE_CURVE ( 'NONE', #9093, #9313, #11440, .T. ) ;
#17367=ORIENTED_EDGE ( 'NONE', *, *, #4576, .T. ) ;
#17371=AXIS2_PLACEMENT_3D ( 'NONE', #909, #15515, #4886 ) ;
#17373=DIRECTION ( 'NONE',  ( -0.000000000000000000, -0.000000000000000000, 1.000000000000000000 ) ) ;
#17375=CARTESIAN_POINT ( 'NONE',  ( -27.98221281341758626, 18.00000000000000000, -6.321711414556880904 ) ) ;
#17376=ORIENTED_EDGE ( 'NONE', *, *, #3678, .F. ) ;
#17378=VERTEX_POINT ( 'NONE', #16021 ) ;
#17379=CARTESIAN_POINT ( 'NONE',  ( -73.64306072442659001, 192.6156044230848181, -25.46745035168474658 ) ) ;
#17380=DIRECTION ( 'NONE',  ( 0.000000000000000000, 0.000000000000000000, 1.000000000000000000 ) ) ;
#17388=ORIENTED_EDGE ( 'NONE', *, *, #671, .F. ) ;
#17392=DIRECTION ( 'NONE',  ( 0.000000000000000000, 0.000000000000000000, -1.000000000000000000 ) ) ;
#17395=CARTESIAN_POINT ( 'NONE',  ( 39.99999999999998579, 20.00000000000000000, -30.00000000000001066 ) ) ;
#17396=DIRECTION ( 'NONE',  ( 1.000000000000000000, 0.000000000000000000, 0.000000000000000000 ) ) ;
#17400=ORIENTED_EDGE ( 'NONE', *, *, #16063, .F. ) ;
#17401=CARTESIAN_POINT ( 'NONE',  ( -77.50000000000001421, 196.6227766016838245, -16.00000000000000000 ) ) ;
#17403=CARTESIAN_POINT ( 'NONE',  ( 15.00000000000903455, 143.2885527162398489, -16.91661185963483760 ) ) ;
#17404=PLANE ( 'NONE',  #10863 ) ;
#17408=CIRCLE ( 'NONE', #1283, 7.500000000000007105 ) ;
#17409=CARTESIAN_POINT ( 'NONE',  ( -48.00000000000000000, 171.6227766016838245, 0.000000000000000000 ) ) ;
#17410=DIRECTION ( 'NONE',  ( 0.000000000000000000, 0.000000000000000000, -1.000000000000000000 ) ) ;
#17411=AXIS2_PLACEMENT_3D ( 'NONE', #3434, #4669, #15374 ) ;
#17412=VERTEX_POINT ( 'NONE', #4073 ) ;
#17414=ORIENTED_EDGE ( 'NONE', *, *, #12575, .F. ) ;
#17417=CARTESIAN_POINT ( 'NONE',  ( -76.51061601766232911, 141.7273756662291930, -18.20613184929476347 ) ) ;
#17422=DIRECTION ( 'NONE',  ( -1.000000000000000000, -0.000000000000000000, -0.000000000000000000 ) ) ;
#17424=CIRCLE ( 'NONE', #3283, 2.500000000000000000 ) ;
#17426=UNCERTAINTY_MEASURE_WITH_UNIT (LENGTH_MEASURE( 1.000000000000000082E-05 ), #3157, 'distance_accuracy_value', 'NONE');
#17429=ORIENTED_EDGE ( 'NONE', *, *, #5189, .F. ) ;
#17431=DIRECTION ( 'NONE',  ( 0.000000000000000000, -1.000000000000000000, -6.123233995736762338E-17 ) ) ;
#17432=ORIENTED_EDGE ( 'NONE', *, *, #994, .T. ) ;
#17433=CARTESIAN_POINT ( 'NONE',  ( 17.00000000000000000, 143.0439382767972631, -16.49999999999984013 ) ) ;
#17435=CARTESIAN_POINT ( 'NONE',  ( 26.13287303778632165, 139.7415755892579341, -8.533400866158022069 ) ) ;
#17436=AXIS2_PLACEMENT_3D ( 'NONE', #5766, #9836, #4539 ) ;
#17437=ORIENTED_EDGE ( 'NONE', *, *, #8405, .T. ) ;
#17438=CARTESIAN_POINT ( 'NONE',  ( -74.72505082391211317, 201.9542783778900059, -13.00000000000000000 ) ) ;
#17439=CIRCLE ( 'NONE', #6396, 20.00000000000000355 ) ;
#17445=CARTESIAN_POINT ( 'NONE',  ( 29.54149365486396661, 18.00000000000000355, -18.67620474358521676 ) ) ;
#17446=CARTESIAN_POINT ( 'NONE',  ( 17.14315908062561533, 17.99999999999886313, -12.73566125713464636 ) ) ;
#17449=CARTESIAN_POINT ( 'NONE',  ( -27.99999999999998224, 10.00000000000000000, -13.00000000000000000 ) ) ;
#17450=ADVANCED_FACE ( 'NONE', ( #14603 ), #17261, .T. ) ;
#17451=CARTESIAN_POINT ( 'NONE',  ( 27.99999999999998224, 9.999999999999998224, -12.99999999999999822 ) ) ;
#17453=CARTESIAN_POINT ( 'NONE',  ( 15.65639489742288681, 128.1581396164810940, -10.28488489824641761 ) ) ;
#17454=CIRCLE ( 'NONE', #15466, 2.500000000000002220 ) ;
#17455=VERTEX_POINT ( 'NONE', #17438 ) ;
#17456=DIRECTION ( 'NONE',  ( -1.000000000000000000, 0.000000000000000000, 0.000000000000000000 ) ) ;
#17463=ADVANCED_FACE ( 'NONE', ( #10525 ), #10437, .F. ) ;
#17464=LINE ( 'NONE', #5335, #3115 ) ;
#17465=ORIENTED_EDGE ( 'NONE', *, *, #15702, .T. ) ;
#17466=DIRECTION ( 'NONE',  ( 1.000000000000000000, 0.000000000000000000, -0.000000000000000000 ) ) ;
#17474=B_SPLINE_CURVE_WITH_KNOTS ( 'NONE', 3,
 ( #3804, #15853, #11856, #17263, #5408, #10527, #17174, #3905, #15933, #11946 ),
 .UNSPECIFIED., .F., .F.,
 ( 4, 2, 2, 2, 4 ),
 ( 2.030441771438897272E-17, 0.002588446031580682403, 0.005176892063161339652, 0.007765338094741996468, 0.01035378412632265502 ),
 .UNSPECIFIED. ) ;
#17476=VERTEX_POINT ( 'NONE', #10797 ) ;
#17478=VERTEX_POINT ( 'NONE', #15851 ) ;
#17480=CARTESIAN_POINT ( 'NONE',  ( -87.04838423995398955, 199.2315236948359143, -18.09598853029520171 ) ) ;
#17482=CIRCLE ( 'NONE', #10958, 30.00000000000000000 ) ;
#17485=AXIS2_PLACEMENT_3D ( 'NONE', #3726, #6555, #5140 ) ;
#17486=DIRECTION ( 'NONE',  ( -1.000000000000000000, 0.000000000000000000, 0.000000000000000000 ) ) ;
#17487=VERTEX_POINT ( 'NONE', #13452 ) ;
#17489=CARTESIAN_POINT ( 'NONE',  ( 30.00000000000001066, 146.6227766016838245, 0.000000000000000000 ) ) ;
#17493=CARTESIAN_POINT ( 'NONE',  ( -100.0000000000000000, 171.6227766016838245, 0.000000000000000000 ) ) ;
#17496=AXIS2_PLACEMENT_3D ( 'NONE', #11773, #14266, #2135 ) ;
#17498=CIRCLE ( 'NONE', #13825, 2.499999999999998668 ) ;
#17500=LINE ( 'NONE', #17401, #4199 ) ;
#17503=CARTESIAN_POINT ( 'NONE',  ( 27.44407568426044008, 138.8271129316868837, -3.666666666666658081 ) ) ;
#17506=AXIS2_PLACEMENT_3D ( 'NONE', #7784, #17272, #5225 ) ;
#17508=CIRCLE ( 'NONE', #10423, 5.999999999999998224 ) ;
#17509=EDGE_LOOP ( 'NONE', ( #1951, #12330, #5558 ) ) ;
#17510=CARTESIAN_POINT ( 'NONE',  ( 33.99999999999998579, 9.999999999999998224, -16.00000000000000000 ) ) ;
#17512=ORIENTED_EDGE ( 'NONE', *, *, #12035, .T. ) ;
#17514=CARTESIAN_POINT ( 'NONE',  ( 15.93460003626534416, 136.8193095811534761, -3.708327557688629206 ) ) ;
#17516=CARTESIAN_POINT ( 'NONE',  ( -83.47886835550096407, 141.7198527106615984, -18.19376952932830349 ) ) ;
#17517=EDGE_CURVE ( 'NONE', #539, #14780, #3613, .T. ) ;
#17520=VERTEX_POINT ( 'NONE', #6460 ) ;
ENDSEC;
END-ISO-10303-21;
